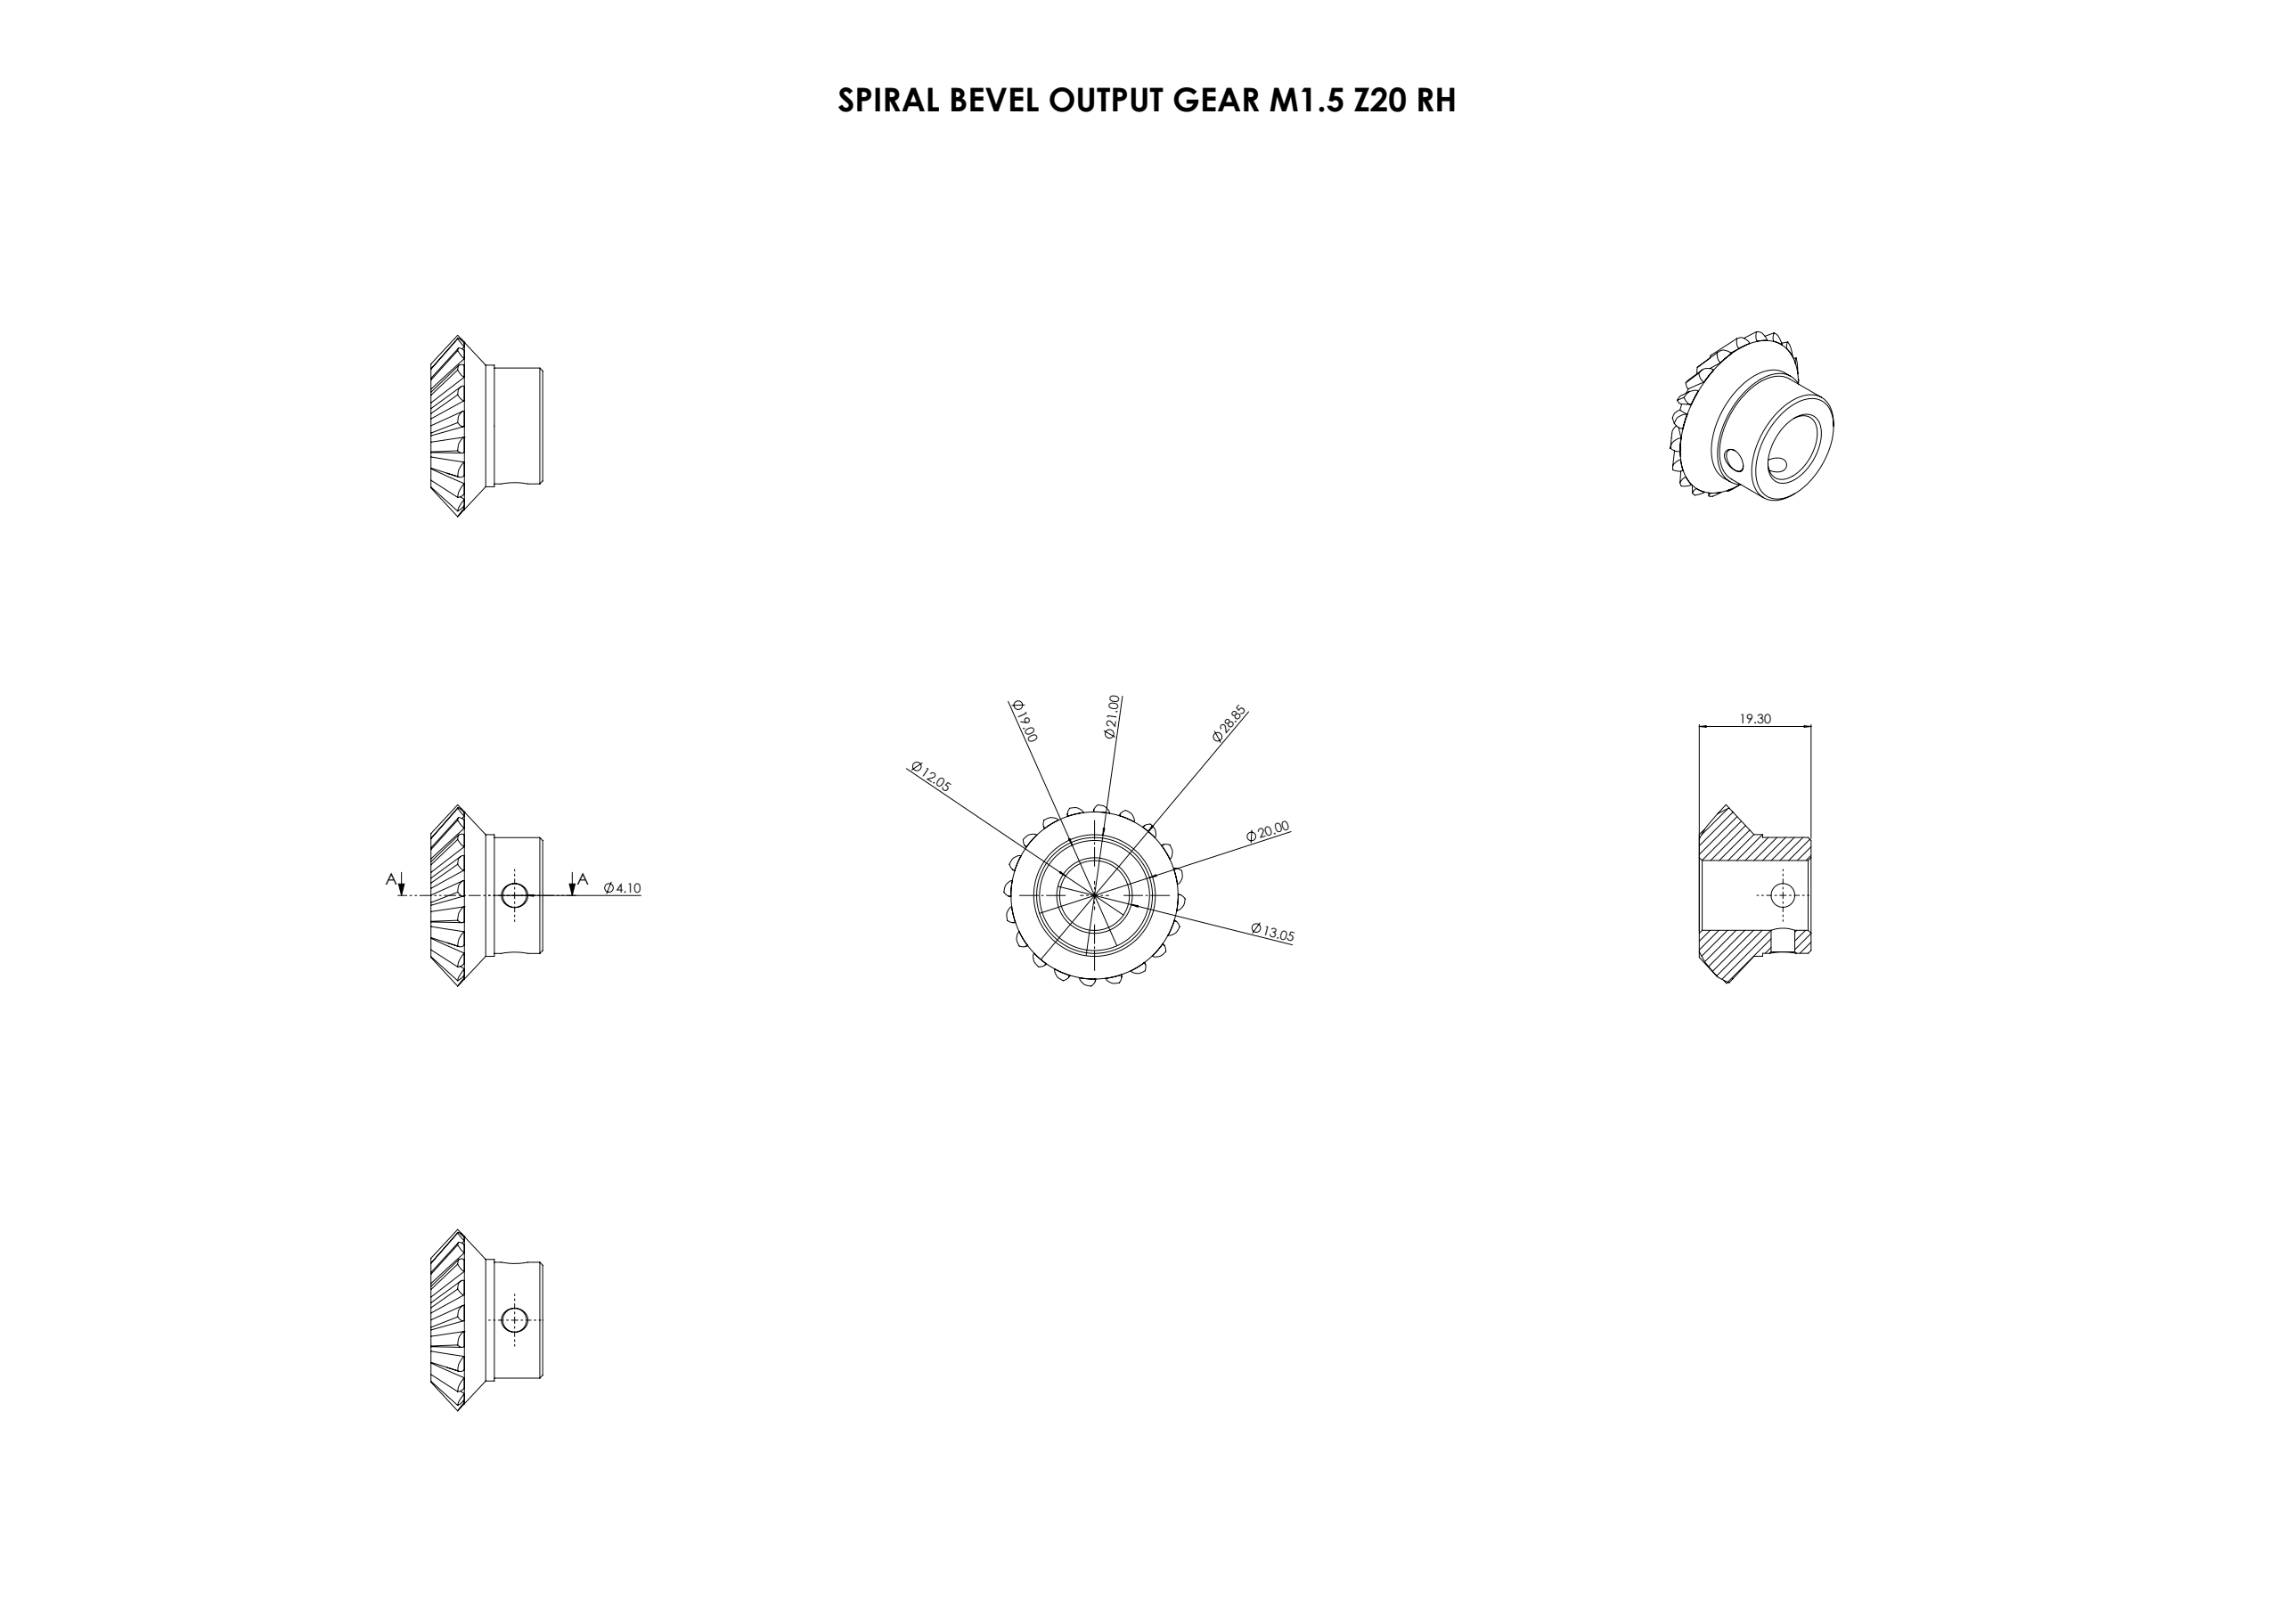
ISO-10303-21;
HEADER;
/* Generated by software containing ST-Developer
 * from STEP Tools, Inc. (www.steptools.com) 
 */

FILE_DESCRIPTION(
/* description */ (''),
/* implementation_level */ '2;1');

FILE_NAME(
/* name */ '03_Spiral_Bevel_Output_Gear_M1.5_Z20_RH.step',
/* time_stamp */ '2026-10-11T09:12:28-07:00',
/* author */ (''),
/* organization */ (''),
/* preprocessor_version */ 'ST-DEVELOPER v20.2',
/* originating_system */ 'Autodesk Translation Framework v15.15.0.0',
/* authorisation */ '');

FILE_SCHEMA (('AUTOMOTIVE_DESIGN { 1 0 10303 214 3 1 1 }'));
ENDSEC;

DATA;
#10=MECHANICAL_DESIGN_GEOMETRIC_PRESENTATION_REPRESENTATION('',(#649),#23254);
#133=B_SPLINE_SURFACE_WITH_KNOTS('',3,3,((#18119,#18120,#18121,#18122),
(#18123,#18124,#18125,#18126),(#18127,#18128,#18129,#18130),(#18131,#18132,
#18133,#18134),(#18135,#18136,#18137,#18138),(#18139,#18140,#18141,#18142)),
 .UNSPECIFIED.,.F.,.F.,.F.,(4,1,1,4),(4,4),(0.,0.285714285714286,0.571428571428571,
1.),(0.,1.),.UNSPECIFIED.);
#134=B_SPLINE_SURFACE_WITH_KNOTS('',3,3,((#18179,#18180,#18181,#18182),
(#18183,#18184,#18185,#18186),(#18187,#18188,#18189,#18190),(#18191,#18192,
#18193,#18194),(#18195,#18196,#18197,#18198),(#18199,#18200,#18201,#18202)),
 .UNSPECIFIED.,.F.,.F.,.F.,(4,1,1,4),(4,4),(0.,0.285714285714286,0.571428571428571,
1.),(0.,1.),.UNSPECIFIED.);
#135=B_SPLINE_SURFACE_WITH_KNOTS('',3,3,((#18239,#18240,#18241,#18242),
(#18243,#18244,#18245,#18246),(#18247,#18248,#18249,#18250),(#18251,#18252,
#18253,#18254),(#18255,#18256,#18257,#18258),(#18259,#18260,#18261,#18262)),
 .UNSPECIFIED.,.F.,.F.,.F.,(4,1,1,4),(4,4),(0.,0.285714285714286,0.571428571428571,
1.),(0.,1.),.UNSPECIFIED.);
#136=B_SPLINE_SURFACE_WITH_KNOTS('',3,3,((#18299,#18300,#18301,#18302),
(#18303,#18304,#18305,#18306),(#18307,#18308,#18309,#18310),(#18311,#18312,
#18313,#18314),(#18315,#18316,#18317,#18318),(#18319,#18320,#18321,#18322)),
 .UNSPECIFIED.,.F.,.F.,.F.,(4,1,1,4),(4,4),(0.,0.285714285714286,0.571428571428571,
1.),(0.,1.),.UNSPECIFIED.);
#137=B_SPLINE_SURFACE_WITH_KNOTS('',3,3,((#18359,#18360,#18361,#18362),
(#18363,#18364,#18365,#18366),(#18367,#18368,#18369,#18370),(#18371,#18372,
#18373,#18374),(#18375,#18376,#18377,#18378),(#18379,#18380,#18381,#18382)),
 .UNSPECIFIED.,.F.,.F.,.F.,(4,1,1,4),(4,4),(0.,0.285714285714286,0.571428571428571,
1.),(0.,1.),.UNSPECIFIED.);
#138=B_SPLINE_SURFACE_WITH_KNOTS('',3,3,((#18419,#18420,#18421,#18422),
(#18423,#18424,#18425,#18426),(#18427,#18428,#18429,#18430),(#18431,#18432,
#18433,#18434),(#18435,#18436,#18437,#18438),(#18439,#18440,#18441,#18442)),
 .UNSPECIFIED.,.F.,.F.,.F.,(4,1,1,4),(4,4),(0.,0.285714285714286,0.571428571428571,
1.),(0.,1.),.UNSPECIFIED.);
#139=B_SPLINE_SURFACE_WITH_KNOTS('',3,3,((#18479,#18480,#18481,#18482),
(#18483,#18484,#18485,#18486),(#18487,#18488,#18489,#18490),(#18491,#18492,
#18493,#18494),(#18495,#18496,#18497,#18498),(#18499,#18500,#18501,#18502)),
 .UNSPECIFIED.,.F.,.F.,.F.,(4,1,1,4),(4,4),(0.,0.285714285714286,0.571428571428571,
1.),(0.,1.),.UNSPECIFIED.);
#140=B_SPLINE_SURFACE_WITH_KNOTS('',3,3,((#18539,#18540,#18541,#18542),
(#18543,#18544,#18545,#18546),(#18547,#18548,#18549,#18550),(#18551,#18552,
#18553,#18554),(#18555,#18556,#18557,#18558),(#18559,#18560,#18561,#18562)),
 .UNSPECIFIED.,.F.,.F.,.F.,(4,1,1,4),(4,4),(0.,0.285714285714286,0.571428571428571,
1.),(0.,1.),.UNSPECIFIED.);
#141=B_SPLINE_SURFACE_WITH_KNOTS('',3,3,((#18599,#18600,#18601,#18602),
(#18603,#18604,#18605,#18606),(#18607,#18608,#18609,#18610),(#18611,#18612,
#18613,#18614),(#18615,#18616,#18617,#18618),(#18619,#18620,#18621,#18622)),
 .UNSPECIFIED.,.F.,.F.,.F.,(4,1,1,4),(4,4),(0.,0.285714285714286,0.571428571428571,
1.),(0.,1.),.UNSPECIFIED.);
#142=B_SPLINE_SURFACE_WITH_KNOTS('',3,3,((#18659,#18660,#18661,#18662),
(#18663,#18664,#18665,#18666),(#18667,#18668,#18669,#18670),(#18671,#18672,
#18673,#18674),(#18675,#18676,#18677,#18678),(#18679,#18680,#18681,#18682)),
 .UNSPECIFIED.,.F.,.F.,.F.,(4,1,1,4),(4,4),(0.,0.285714285714286,0.571428571428571,
1.),(0.,1.),.UNSPECIFIED.);
#143=B_SPLINE_SURFACE_WITH_KNOTS('',3,3,((#18719,#18720,#18721,#18722),
(#18723,#18724,#18725,#18726),(#18727,#18728,#18729,#18730),(#18731,#18732,
#18733,#18734),(#18735,#18736,#18737,#18738),(#18739,#18740,#18741,#18742)),
 .UNSPECIFIED.,.F.,.F.,.F.,(4,1,1,4),(4,4),(0.,0.285714285714286,0.571428571428571,
1.),(0.,1.),.UNSPECIFIED.);
#144=B_SPLINE_SURFACE_WITH_KNOTS('',3,3,((#18779,#18780,#18781,#18782),
(#18783,#18784,#18785,#18786),(#18787,#18788,#18789,#18790),(#18791,#18792,
#18793,#18794),(#18795,#18796,#18797,#18798),(#18799,#18800,#18801,#18802)),
 .UNSPECIFIED.,.F.,.F.,.F.,(4,1,1,4),(4,4),(0.,0.285714285714286,0.571428571428571,
1.),(0.,1.),.UNSPECIFIED.);
#145=B_SPLINE_SURFACE_WITH_KNOTS('',3,3,((#18839,#18840,#18841,#18842),
(#18843,#18844,#18845,#18846),(#18847,#18848,#18849,#18850),(#18851,#18852,
#18853,#18854),(#18855,#18856,#18857,#18858),(#18859,#18860,#18861,#18862)),
 .UNSPECIFIED.,.F.,.F.,.F.,(4,1,1,4),(4,4),(0.,0.285714285714286,0.571428571428571,
1.),(0.,1.),.UNSPECIFIED.);
#146=B_SPLINE_SURFACE_WITH_KNOTS('',3,3,((#18899,#18900,#18901,#18902),
(#18903,#18904,#18905,#18906),(#18907,#18908,#18909,#18910),(#18911,#18912,
#18913,#18914),(#18915,#18916,#18917,#18918),(#18919,#18920,#18921,#18922)),
 .UNSPECIFIED.,.F.,.F.,.F.,(4,1,1,4),(4,4),(0.,0.285714285714286,0.571428571428571,
1.),(0.,1.),.UNSPECIFIED.);
#147=B_SPLINE_SURFACE_WITH_KNOTS('',3,3,((#18959,#18960,#18961,#18962),
(#18963,#18964,#18965,#18966),(#18967,#18968,#18969,#18970),(#18971,#18972,
#18973,#18974),(#18975,#18976,#18977,#18978),(#18979,#18980,#18981,#18982)),
 .UNSPECIFIED.,.F.,.F.,.F.,(4,1,1,4),(4,4),(0.,0.285714285714286,0.571428571428571,
1.),(0.,1.),.UNSPECIFIED.);
#148=B_SPLINE_SURFACE_WITH_KNOTS('',3,3,((#19019,#19020,#19021,#19022),
(#19023,#19024,#19025,#19026),(#19027,#19028,#19029,#19030),(#19031,#19032,
#19033,#19034),(#19035,#19036,#19037,#19038),(#19039,#19040,#19041,#19042)),
 .UNSPECIFIED.,.F.,.F.,.F.,(4,1,1,4),(4,4),(0.,0.285714285714286,0.571428571428571,
1.),(0.,1.),.UNSPECIFIED.);
#149=B_SPLINE_SURFACE_WITH_KNOTS('',3,3,((#19079,#19080,#19081,#19082),
(#19083,#19084,#19085,#19086),(#19087,#19088,#19089,#19090),(#19091,#19092,
#19093,#19094),(#19095,#19096,#19097,#19098),(#19099,#19100,#19101,#19102)),
 .UNSPECIFIED.,.F.,.F.,.F.,(4,1,1,4),(4,4),(0.,0.285714285714286,0.571428571428571,
1.),(0.,1.),.UNSPECIFIED.);
#150=B_SPLINE_SURFACE_WITH_KNOTS('',3,3,((#19139,#19140,#19141,#19142),
(#19143,#19144,#19145,#19146),(#19147,#19148,#19149,#19150),(#19151,#19152,
#19153,#19154),(#19155,#19156,#19157,#19158),(#19159,#19160,#19161,#19162)),
 .UNSPECIFIED.,.F.,.F.,.F.,(4,1,1,4),(4,4),(0.,0.285714285714286,0.571428571428571,
1.),(0.,1.),.UNSPECIFIED.);
#151=B_SPLINE_SURFACE_WITH_KNOTS('',3,3,((#19199,#19200,#19201,#19202),
(#19203,#19204,#19205,#19206),(#19207,#19208,#19209,#19210),(#19211,#19212,
#19213,#19214),(#19215,#19216,#19217,#19218),(#19219,#19220,#19221,#19222)),
 .UNSPECIFIED.,.F.,.F.,.F.,(4,1,1,4),(4,4),(0.,0.285714285714286,0.571428571428571,
1.),(0.,1.),.UNSPECIFIED.);
#152=B_SPLINE_SURFACE_WITH_KNOTS('',3,3,((#19259,#19260,#19261,#19262),
(#19263,#19264,#19265,#19266),(#19267,#19268,#19269,#19270),(#19271,#19272,
#19273,#19274),(#19275,#19276,#19277,#19278),(#19279,#19280,#19281,#19282)),
 .UNSPECIFIED.,.F.,.F.,.F.,(4,1,1,4),(4,4),(0.,0.285714285714286,0.571428571428571,
1.),(0.,1.),.UNSPECIFIED.);
#153=B_SPLINE_SURFACE_WITH_KNOTS('',3,3,((#19319,#19320,#19321,#19322),
(#19323,#19324,#19325,#19326),(#19327,#19328,#19329,#19330),(#19331,#19332,
#19333,#19334),(#19335,#19336,#19337,#19338),(#19339,#19340,#19341,#19342),
(#19343,#19344,#19345,#19346),(#19347,#19348,#19349,#19350),(#19351,#19352,
#19353,#19354),(#19355,#19356,#19357,#19358),(#19359,#19360,#19361,#19362)),
 .UNSPECIFIED.,.F.,.F.,.F.,(4,1,1,1,1,1,1,1,4),(4,4),(0.,0.142857142857143,
0.285714285714286,0.357142857142857,0.428571428571429,0.571428571428571,
0.785714285714286,0.857142857142857,1.),(0.,1.),.UNSPECIFIED.);
#154=B_SPLINE_SURFACE_WITH_KNOTS('',3,3,((#19974,#19975,#19976,#19977),
(#19978,#19979,#19980,#19981),(#19982,#19983,#19984,#19985),(#19986,#19987,
#19988,#19989),(#19990,#19991,#19992,#19993),(#19994,#19995,#19996,#19997),
(#19998,#19999,#20000,#20001),(#20002,#20003,#20004,#20005),(#20006,#20007,
#20008,#20009),(#20010,#20011,#20012,#20013),(#20014,#20015,#20016,#20017)),
 .UNSPECIFIED.,.F.,.F.,.F.,(4,1,1,1,1,1,1,1,4),(4,4),(0.,0.142857142857143,
0.285714285714286,0.357142857142857,0.428571428571429,0.571428571428571,
0.785714285714286,0.857142857142857,1.),(0.,1.),.UNSPECIFIED.);
#155=B_SPLINE_SURFACE_WITH_KNOTS('',3,3,((#20025,#20026,#20027,#20028),
(#20029,#20030,#20031,#20032),(#20033,#20034,#20035,#20036),(#20037,#20038,
#20039,#20040),(#20041,#20042,#20043,#20044),(#20045,#20046,#20047,#20048),
(#20049,#20050,#20051,#20052),(#20053,#20054,#20055,#20056),(#20057,#20058,
#20059,#20060),(#20061,#20062,#20063,#20064),(#20065,#20066,#20067,#20068),
(#20069,#20070,#20071,#20072)),.UNSPECIFIED.,.F.,.F.,.F.,(4,1,1,1,1,1,1,
1,1,4),(4,4),(0.,0.142857142857143,0.285714285714286,0.321428571428571,
0.357142857142857,0.428571428571429,0.571428571428571,0.785714285714286,
0.857142857142857,1.),(0.,1.),.UNSPECIFIED.);
#156=B_SPLINE_SURFACE_WITH_KNOTS('',3,3,((#20080,#20081,#20082,#20083),
(#20084,#20085,#20086,#20087),(#20088,#20089,#20090,#20091),(#20092,#20093,
#20094,#20095),(#20096,#20097,#20098,#20099),(#20100,#20101,#20102,#20103),
(#20104,#20105,#20106,#20107),(#20108,#20109,#20110,#20111),(#20112,#20113,
#20114,#20115),(#20116,#20117,#20118,#20119),(#20120,#20121,#20122,#20123),
(#20124,#20125,#20126,#20127)),.UNSPECIFIED.,.F.,.F.,.F.,(4,1,1,1,1,1,1,
1,1,4),(4,4),(0.,0.142857142857143,0.285714285714286,0.321428571428571,
0.357142857142857,0.428571428571429,0.571428571428571,0.785714285714286,
0.857142857142857,1.),(0.,1.),.UNSPECIFIED.);
#157=B_SPLINE_SURFACE_WITH_KNOTS('',3,3,((#20135,#20136,#20137,#20138),
(#20139,#20140,#20141,#20142),(#20143,#20144,#20145,#20146),(#20147,#20148,
#20149,#20150),(#20151,#20152,#20153,#20154),(#20155,#20156,#20157,#20158),
(#20159,#20160,#20161,#20162),(#20163,#20164,#20165,#20166),(#20167,#20168,
#20169,#20170),(#20171,#20172,#20173,#20174),(#20175,#20176,#20177,#20178)),
 .UNSPECIFIED.,.F.,.F.,.F.,(4,1,1,1,1,1,1,1,4),(4,4),(0.,0.142857142857143,
0.285714285714286,0.357142857142857,0.428571428571429,0.571428571428571,
0.785714285714286,0.857142857142857,1.),(0.,1.),.UNSPECIFIED.);
#158=B_SPLINE_SURFACE_WITH_KNOTS('',3,3,((#20186,#20187,#20188,#20189),
(#20190,#20191,#20192,#20193),(#20194,#20195,#20196,#20197),(#20198,#20199,
#20200,#20201),(#20202,#20203,#20204,#20205),(#20206,#20207,#20208,#20209),
(#20210,#20211,#20212,#20213),(#20214,#20215,#20216,#20217),(#20218,#20219,
#20220,#20221),(#20222,#20223,#20224,#20225),(#20226,#20227,#20228,#20229)),
 .UNSPECIFIED.,.F.,.F.,.F.,(4,1,1,1,1,1,1,1,4),(4,4),(0.,0.142857142857143,
0.285714285714286,0.357142857142857,0.428571428571429,0.571428571428571,
0.785714285714286,0.857142857142857,1.),(0.,1.),.UNSPECIFIED.);
#159=B_SPLINE_SURFACE_WITH_KNOTS('',3,3,((#20237,#20238,#20239,#20240),
(#20241,#20242,#20243,#20244),(#20245,#20246,#20247,#20248),(#20249,#20250,
#20251,#20252),(#20253,#20254,#20255,#20256),(#20257,#20258,#20259,#20260),
(#20261,#20262,#20263,#20264),(#20265,#20266,#20267,#20268),(#20269,#20270,
#20271,#20272),(#20273,#20274,#20275,#20276),(#20277,#20278,#20279,#20280)),
 .UNSPECIFIED.,.F.,.F.,.F.,(4,1,1,1,1,1,1,1,4),(4,4),(0.,0.142857142857143,
0.285714285714286,0.357142857142857,0.428571428571429,0.571428571428571,
0.785714285714286,0.857142857142857,1.),(0.,1.),.UNSPECIFIED.);
#160=B_SPLINE_SURFACE_WITH_KNOTS('',3,3,((#20288,#20289,#20290,#20291),
(#20292,#20293,#20294,#20295),(#20296,#20297,#20298,#20299),(#20300,#20301,
#20302,#20303),(#20304,#20305,#20306,#20307),(#20308,#20309,#20310,#20311),
(#20312,#20313,#20314,#20315),(#20316,#20317,#20318,#20319),(#20320,#20321,
#20322,#20323),(#20324,#20325,#20326,#20327),(#20328,#20329,#20330,#20331),
(#20332,#20333,#20334,#20335)),.UNSPECIFIED.,.F.,.F.,.F.,(4,1,1,1,1,1,1,
1,1,4),(4,4),(0.,0.142857142857143,0.285714285714286,0.321428571428571,
0.357142857142857,0.428571428571429,0.571428571428571,0.785714285714286,
0.857142857142857,1.),(0.,1.),.UNSPECIFIED.);
#161=B_SPLINE_SURFACE_WITH_KNOTS('',3,3,((#20343,#20344,#20345,#20346),
(#20347,#20348,#20349,#20350),(#20351,#20352,#20353,#20354),(#20355,#20356,
#20357,#20358),(#20359,#20360,#20361,#20362),(#20363,#20364,#20365,#20366),
(#20367,#20368,#20369,#20370),(#20371,#20372,#20373,#20374),(#20375,#20376,
#20377,#20378),(#20379,#20380,#20381,#20382),(#20383,#20384,#20385,#20386),
(#20387,#20388,#20389,#20390)),.UNSPECIFIED.,.F.,.F.,.F.,(4,1,1,1,1,1,1,
1,1,4),(4,4),(0.,0.142857142857143,0.285714285714286,0.321428571428571,
0.357142857142857,0.428571428571429,0.571428571428571,0.785714285714286,
0.857142857142857,1.),(0.,1.),.UNSPECIFIED.);
#162=B_SPLINE_SURFACE_WITH_KNOTS('',3,3,((#20398,#20399,#20400,#20401),
(#20402,#20403,#20404,#20405),(#20406,#20407,#20408,#20409),(#20410,#20411,
#20412,#20413),(#20414,#20415,#20416,#20417),(#20418,#20419,#20420,#20421),
(#20422,#20423,#20424,#20425),(#20426,#20427,#20428,#20429),(#20430,#20431,
#20432,#20433),(#20434,#20435,#20436,#20437),(#20438,#20439,#20440,#20441)),
 .UNSPECIFIED.,.F.,.F.,.F.,(4,1,1,1,1,1,1,1,4),(4,4),(0.,0.142857142857143,
0.285714285714286,0.357142857142857,0.428571428571429,0.571428571428571,
0.785714285714286,0.857142857142857,1.),(0.,1.),.UNSPECIFIED.);
#163=B_SPLINE_SURFACE_WITH_KNOTS('',3,3,((#20449,#20450,#20451,#20452),
(#20453,#20454,#20455,#20456),(#20457,#20458,#20459,#20460),(#20461,#20462,
#20463,#20464),(#20465,#20466,#20467,#20468),(#20469,#20470,#20471,#20472),
(#20473,#20474,#20475,#20476),(#20477,#20478,#20479,#20480),(#20481,#20482,
#20483,#20484),(#20485,#20486,#20487,#20488),(#20489,#20490,#20491,#20492)),
 .UNSPECIFIED.,.F.,.F.,.F.,(4,1,1,1,1,1,1,1,4),(4,4),(0.,0.142857142857143,
0.285714285714286,0.357142857142857,0.428571428571429,0.571428571428571,
0.785714285714286,0.857142857142857,1.),(0.,1.),.UNSPECIFIED.);
#164=B_SPLINE_SURFACE_WITH_KNOTS('',3,3,((#20500,#20501,#20502,#20503),
(#20504,#20505,#20506,#20507),(#20508,#20509,#20510,#20511),(#20512,#20513,
#20514,#20515),(#20516,#20517,#20518,#20519),(#20520,#20521,#20522,#20523),
(#20524,#20525,#20526,#20527),(#20528,#20529,#20530,#20531),(#20532,#20533,
#20534,#20535),(#20536,#20537,#20538,#20539),(#20540,#20541,#20542,#20543)),
 .UNSPECIFIED.,.F.,.F.,.F.,(4,1,1,1,1,1,1,1,4),(4,4),(0.,0.142857142857143,
0.285714285714286,0.357142857142857,0.428571428571429,0.571428571428571,
0.785714285714286,0.857142857142857,1.),(0.,1.),.UNSPECIFIED.);
#165=B_SPLINE_SURFACE_WITH_KNOTS('',3,3,((#20551,#20552,#20553,#20554),
(#20555,#20556,#20557,#20558),(#20559,#20560,#20561,#20562),(#20563,#20564,
#20565,#20566),(#20567,#20568,#20569,#20570),(#20571,#20572,#20573,#20574),
(#20575,#20576,#20577,#20578),(#20579,#20580,#20581,#20582),(#20583,#20584,
#20585,#20586),(#20587,#20588,#20589,#20590),(#20591,#20592,#20593,#20594),
(#20595,#20596,#20597,#20598)),.UNSPECIFIED.,.F.,.F.,.F.,(4,1,1,1,1,1,1,
1,1,4),(4,4),(0.,0.142857142857143,0.285714285714286,0.321428571428571,
0.357142857142857,0.428571428571429,0.571428571428571,0.785714285714286,
0.857142857142857,1.),(0.,1.),.UNSPECIFIED.);
#166=B_SPLINE_SURFACE_WITH_KNOTS('',3,3,((#20606,#20607,#20608,#20609),
(#20610,#20611,#20612,#20613),(#20614,#20615,#20616,#20617),(#20618,#20619,
#20620,#20621),(#20622,#20623,#20624,#20625),(#20626,#20627,#20628,#20629),
(#20630,#20631,#20632,#20633),(#20634,#20635,#20636,#20637),(#20638,#20639,
#20640,#20641),(#20642,#20643,#20644,#20645),(#20646,#20647,#20648,#20649),
(#20650,#20651,#20652,#20653)),.UNSPECIFIED.,.F.,.F.,.F.,(4,1,1,1,1,1,1,
1,1,4),(4,4),(0.,0.142857142857143,0.285714285714286,0.321428571428571,
0.357142857142857,0.428571428571429,0.571428571428571,0.785714285714286,
0.857142857142857,1.),(0.,1.),.UNSPECIFIED.);
#167=B_SPLINE_SURFACE_WITH_KNOTS('',3,3,((#20661,#20662,#20663,#20664),
(#20665,#20666,#20667,#20668),(#20669,#20670,#20671,#20672),(#20673,#20674,
#20675,#20676),(#20677,#20678,#20679,#20680),(#20681,#20682,#20683,#20684),
(#20685,#20686,#20687,#20688),(#20689,#20690,#20691,#20692),(#20693,#20694,
#20695,#20696),(#20697,#20698,#20699,#20700),(#20701,#20702,#20703,#20704)),
 .UNSPECIFIED.,.F.,.F.,.F.,(4,1,1,1,1,1,1,1,4),(4,4),(0.,0.142857142857143,
0.285714285714286,0.357142857142857,0.428571428571429,0.571428571428571,
0.785714285714286,0.857142857142857,1.),(0.,1.),.UNSPECIFIED.);
#168=B_SPLINE_SURFACE_WITH_KNOTS('',3,3,((#20712,#20713,#20714,#20715),
(#20716,#20717,#20718,#20719),(#20720,#20721,#20722,#20723),(#20724,#20725,
#20726,#20727),(#20728,#20729,#20730,#20731),(#20732,#20733,#20734,#20735),
(#20736,#20737,#20738,#20739),(#20740,#20741,#20742,#20743),(#20744,#20745,
#20746,#20747),(#20748,#20749,#20750,#20751),(#20752,#20753,#20754,#20755)),
 .UNSPECIFIED.,.F.,.F.,.F.,(4,1,1,1,1,1,1,1,4),(4,4),(0.,0.142857142857143,
0.285714285714286,0.357142857142857,0.428571428571429,0.571428571428571,
0.785714285714286,0.857142857142857,1.),(0.,1.),.UNSPECIFIED.);
#169=B_SPLINE_SURFACE_WITH_KNOTS('',3,3,((#20763,#20764,#20765,#20766),
(#20767,#20768,#20769,#20770),(#20771,#20772,#20773,#20774),(#20775,#20776,
#20777,#20778),(#20779,#20780,#20781,#20782),(#20783,#20784,#20785,#20786),
(#20787,#20788,#20789,#20790),(#20791,#20792,#20793,#20794),(#20795,#20796,
#20797,#20798),(#20799,#20800,#20801,#20802),(#20803,#20804,#20805,#20806)),
 .UNSPECIFIED.,.F.,.F.,.F.,(4,1,1,1,1,1,1,1,4),(4,4),(0.,0.142857142857143,
0.285714285714286,0.357142857142857,0.428571428571429,0.571428571428571,
0.785714285714286,0.857142857142857,1.),(0.,1.),.UNSPECIFIED.);
#170=B_SPLINE_SURFACE_WITH_KNOTS('',3,3,((#20814,#20815,#20816,#20817),
(#20818,#20819,#20820,#20821),(#20822,#20823,#20824,#20825),(#20826,#20827,
#20828,#20829),(#20830,#20831,#20832,#20833),(#20834,#20835,#20836,#20837),
(#20838,#20839,#20840,#20841),(#20842,#20843,#20844,#20845),(#20846,#20847,
#20848,#20849),(#20850,#20851,#20852,#20853),(#20854,#20855,#20856,#20857),
(#20858,#20859,#20860,#20861)),.UNSPECIFIED.,.F.,.F.,.F.,(4,1,1,1,1,1,1,
1,1,4),(4,4),(0.,0.142857142857143,0.285714285714286,0.321428571428571,
0.357142857142857,0.428571428571429,0.571428571428571,0.785714285714286,
0.857142857142857,1.),(0.,1.),.UNSPECIFIED.);
#171=B_SPLINE_SURFACE_WITH_KNOTS('',3,3,((#20869,#20870,#20871,#20872),
(#20873,#20874,#20875,#20876),(#20877,#20878,#20879,#20880),(#20881,#20882,
#20883,#20884),(#20885,#20886,#20887,#20888),(#20889,#20890,#20891,#20892),
(#20893,#20894,#20895,#20896),(#20897,#20898,#20899,#20900),(#20901,#20902,
#20903,#20904),(#20905,#20906,#20907,#20908),(#20909,#20910,#20911,#20912),
(#20913,#20914,#20915,#20916)),.UNSPECIFIED.,.F.,.F.,.F.,(4,1,1,1,1,1,1,
1,1,4),(4,4),(0.,0.142857142857143,0.285714285714286,0.321428571428571,
0.357142857142857,0.428571428571429,0.571428571428571,0.785714285714286,
0.857142857142857,1.),(0.,1.),.UNSPECIFIED.);
#172=B_SPLINE_SURFACE_WITH_KNOTS('',3,3,((#20924,#20925,#20926,#20927),
(#20928,#20929,#20930,#20931),(#20932,#20933,#20934,#20935),(#20936,#20937,
#20938,#20939),(#20940,#20941,#20942,#20943),(#20944,#20945,#20946,#20947),
(#20948,#20949,#20950,#20951),(#20952,#20953,#20954,#20955),(#20956,#20957,
#20958,#20959),(#20960,#20961,#20962,#20963),(#20964,#20965,#20966,#20967)),
 .UNSPECIFIED.,.F.,.F.,.F.,(4,1,1,1,1,1,1,1,4),(4,4),(0.,0.142857142857143,
0.285714285714286,0.357142857142857,0.428571428571429,0.571428571428571,
0.785714285714286,0.857142857142857,1.),(0.,1.),.UNSPECIFIED.);
#255=(
BOUNDED_CURVE()
B_SPLINE_CURVE(5,(#16035,#16036,#16037,#16038,#16039,#16040,#16041,#16042,
#16043,#16044,#16045,#16046,#16047,#16048,#16049,#16050,#16051,#16052,#16053,
#16054,#16055,#16056,#16057,#16058,#16059,#16060,#16061,#16062,#16063,#16064,
#16065,#16066,#16067,#16068,#16069),.UNSPECIFIED.,.F.,.F.)
B_SPLINE_CURVE_WITH_KNOTS((6,1,1,1,1,1,1,1,1,1,1,1,1,1,1,1,1,1,1,1,1,1,
1,1,1,1,1,1,1,1,6),(0.,0.0333333333333333,0.0666666666666667,0.1,0.133333333333333,
0.166666666666667,0.2,0.233333333333333,0.266666666666667,0.3,0.333333333333333,
0.366666666666667,0.4,0.433333333333333,0.466666666666667,0.5,0.533333333333333,
0.566666666666667,0.6,0.633333333333333,0.666666666666667,0.7,0.733333333333333,
0.766666666666667,0.8,0.833333333333333,0.866666666666667,0.9,0.933333333333333,
0.966666666666667,1.),.UNSPECIFIED.)
CURVE()
GEOMETRIC_REPRESENTATION_ITEM()
RATIONAL_B_SPLINE_CURVE((1.,1.,1.,1.,1.,1.,1.,1.,1.,1.,1.,1.,1.,1.,1.,1.,
1.,1.,1.,1.,1.,1.,1.,1.,1.,1.,1.,1.,1.,1.,1.,1.,1.,1.,1.))
REPRESENTATION_ITEM('')
);
#256=(
BOUNDED_CURVE()
B_SPLINE_CURVE(5,(#16071,#16072,#16073,#16074,#16075,#16076,#16077,#16078,
#16079,#16080,#16081,#16082,#16083,#16084,#16085,#16086,#16087,#16088,#16089,
#16090,#16091,#16092,#16093,#16094,#16095,#16096,#16097,#16098,#16099,#16100,
#16101,#16102,#16103,#16104,#16105),.UNSPECIFIED.,.F.,.F.)
B_SPLINE_CURVE_WITH_KNOTS((6,1,1,1,1,1,1,1,1,1,1,1,1,1,1,1,1,1,1,1,1,1,
1,1,1,1,1,1,1,1,6),(0.,0.0333333333333333,0.0666666666666667,0.1,0.133333333333333,
0.166666666666667,0.2,0.233333333333333,0.266666666666667,0.3,0.333333333333333,
0.366666666666667,0.4,0.433333333333333,0.466666666666667,0.5,0.533333333333333,
0.566666666666667,0.6,0.633333333333333,0.666666666666667,0.7,0.733333333333333,
0.766666666666667,0.8,0.833333333333333,0.866666666666667,0.9,0.933333333333333,
0.966666666666667,1.),.UNSPECIFIED.)
CURVE()
GEOMETRIC_REPRESENTATION_ITEM()
RATIONAL_B_SPLINE_CURVE((1.,1.,1.,1.,1.,1.,1.,1.,1.,1.,1.,1.,1.,1.,1.,1.,
1.,1.,1.,1.,1.,1.,1.,1.,1.,1.,1.,1.,1.,1.,1.,1.,1.,1.,1.))
REPRESENTATION_ITEM('')
);
#257=(
BOUNDED_CURVE()
B_SPLINE_CURVE(5,(#16109,#16110,#16111,#16112,#16113,#16114,#16115,#16116,
#16117,#16118,#16119,#16120,#16121,#16122,#16123,#16124,#16125,#16126,#16127,
#16128,#16129,#16130,#16131,#16132,#16133,#16134,#16135,#16136,#16137,#16138,
#16139,#16140,#16141,#16142,#16143),.UNSPECIFIED.,.F.,.F.)
B_SPLINE_CURVE_WITH_KNOTS((6,1,1,1,1,1,1,1,1,1,1,1,1,1,1,1,1,1,1,1,1,1,
1,1,1,1,1,1,1,1,6),(0.,0.0333333333333333,0.0666666666666667,0.1,0.133333333333333,
0.166666666666667,0.2,0.233333333333333,0.266666666666667,0.3,0.333333333333333,
0.366666666666667,0.4,0.433333333333333,0.466666666666667,0.5,0.533333333333333,
0.566666666666667,0.6,0.633333333333333,0.666666666666667,0.7,0.733333333333333,
0.766666666666667,0.8,0.833333333333333,0.866666666666667,0.9,0.933333333333333,
0.966666666666667,1.),.UNSPECIFIED.)
CURVE()
GEOMETRIC_REPRESENTATION_ITEM()
RATIONAL_B_SPLINE_CURVE((1.,1.,1.,1.,1.,1.,1.,1.,1.,1.,1.,1.,1.,1.,1.,1.,
1.,1.,1.,1.,1.,1.,1.,1.,1.,1.,1.,1.,1.,1.,1.,1.,1.,1.,1.))
REPRESENTATION_ITEM('')
);
#258=(
BOUNDED_CURVE()
B_SPLINE_CURVE(5,(#16145,#16146,#16147,#16148,#16149,#16150,#16151,#16152,
#16153,#16154,#16155,#16156,#16157,#16158,#16159,#16160,#16161,#16162,#16163,
#16164,#16165,#16166,#16167,#16168,#16169,#16170,#16171,#16172,#16173,#16174,
#16175,#16176,#16177,#16178,#16179),.UNSPECIFIED.,.F.,.F.)
B_SPLINE_CURVE_WITH_KNOTS((6,1,1,1,1,1,1,1,1,1,1,1,1,1,1,1,1,1,1,1,1,1,
1,1,1,1,1,1,1,1,6),(0.,0.0333333333333333,0.0666666666666667,0.1,0.133333333333333,
0.166666666666667,0.2,0.233333333333333,0.266666666666667,0.3,0.333333333333333,
0.366666666666667,0.4,0.433333333333333,0.466666666666667,0.5,0.533333333333333,
0.566666666666667,0.6,0.633333333333333,0.666666666666667,0.7,0.733333333333333,
0.766666666666667,0.8,0.833333333333333,0.866666666666667,0.9,0.933333333333333,
0.966666666666667,1.),.UNSPECIFIED.)
CURVE()
GEOMETRIC_REPRESENTATION_ITEM()
RATIONAL_B_SPLINE_CURVE((1.,1.,1.,1.,1.,1.,1.,1.,1.,1.,1.,1.,1.,1.,1.,1.,
1.,1.,1.,1.,1.,1.,1.,1.,1.,1.,1.,1.,1.,1.,1.,1.,1.,1.,1.))
REPRESENTATION_ITEM('')
);
#259=(
BOUNDED_CURVE()
B_SPLINE_CURVE(5,(#16183,#16184,#16185,#16186,#16187,#16188,#16189,#16190,
#16191,#16192,#16193,#16194,#16195,#16196,#16197,#16198,#16199,#16200,#16201,
#16202,#16203,#16204,#16205,#16206,#16207,#16208,#16209,#16210,#16211,#16212,
#16213,#16214,#16215,#16216,#16217),.UNSPECIFIED.,.F.,.F.)
B_SPLINE_CURVE_WITH_KNOTS((6,1,1,1,1,1,1,1,1,1,1,1,1,1,1,1,1,1,1,1,1,1,
1,1,1,1,1,1,1,1,6),(0.,0.0333333333333333,0.0666666666666667,0.1,0.133333333333333,
0.166666666666667,0.2,0.233333333333333,0.266666666666667,0.3,0.333333333333333,
0.366666666666667,0.4,0.433333333333333,0.466666666666667,0.5,0.533333333333333,
0.566666666666667,0.6,0.633333333333333,0.666666666666667,0.7,0.733333333333333,
0.766666666666667,0.8,0.833333333333333,0.866666666666667,0.9,0.933333333333333,
0.966666666666667,1.),.UNSPECIFIED.)
CURVE()
GEOMETRIC_REPRESENTATION_ITEM()
RATIONAL_B_SPLINE_CURVE((1.,1.,1.,1.,1.,1.,1.,1.,1.,1.,1.,1.,1.,1.,1.,1.,
1.,1.,1.,1.,1.,1.,1.,1.,1.,1.,1.,1.,1.,1.,1.,1.,1.,1.,1.))
REPRESENTATION_ITEM('')
);
#260=(
BOUNDED_CURVE()
B_SPLINE_CURVE(5,(#16219,#16220,#16221,#16222,#16223,#16224,#16225,#16226,
#16227,#16228,#16229,#16230,#16231,#16232,#16233,#16234,#16235,#16236,#16237,
#16238,#16239,#16240,#16241,#16242,#16243,#16244,#16245,#16246,#16247,#16248,
#16249,#16250,#16251,#16252,#16253),.UNSPECIFIED.,.F.,.F.)
B_SPLINE_CURVE_WITH_KNOTS((6,1,1,1,1,1,1,1,1,1,1,1,1,1,1,1,1,1,1,1,1,1,
1,1,1,1,1,1,1,1,6),(0.,0.0333333333333333,0.0666666666666667,0.1,0.133333333333333,
0.166666666666667,0.2,0.233333333333333,0.266666666666667,0.3,0.333333333333333,
0.366666666666667,0.4,0.433333333333333,0.466666666666667,0.5,0.533333333333333,
0.566666666666667,0.6,0.633333333333333,0.666666666666667,0.7,0.733333333333333,
0.766666666666667,0.8,0.833333333333333,0.866666666666667,0.9,0.933333333333333,
0.966666666666667,1.),.UNSPECIFIED.)
CURVE()
GEOMETRIC_REPRESENTATION_ITEM()
RATIONAL_B_SPLINE_CURVE((1.,1.,1.,1.,1.,1.,1.,1.,1.,1.,1.,1.,1.,1.,1.,1.,
1.,1.,1.,1.,1.,1.,1.,1.,1.,1.,1.,1.,1.,1.,1.,1.,1.,1.,1.))
REPRESENTATION_ITEM('')
);
#261=(
BOUNDED_CURVE()
B_SPLINE_CURVE(5,(#16257,#16258,#16259,#16260,#16261,#16262,#16263,#16264,
#16265,#16266,#16267,#16268,#16269,#16270,#16271,#16272,#16273,#16274,#16275,
#16276,#16277,#16278,#16279,#16280,#16281,#16282,#16283,#16284,#16285,#16286,
#16287,#16288,#16289,#16290,#16291),.UNSPECIFIED.,.F.,.F.)
B_SPLINE_CURVE_WITH_KNOTS((6,1,1,1,1,1,1,1,1,1,1,1,1,1,1,1,1,1,1,1,1,1,
1,1,1,1,1,1,1,1,6),(0.,0.0333333333333333,0.0666666666666667,0.1,0.133333333333333,
0.166666666666667,0.2,0.233333333333333,0.266666666666667,0.3,0.333333333333333,
0.366666666666667,0.4,0.433333333333333,0.466666666666667,0.5,0.533333333333333,
0.566666666666667,0.6,0.633333333333333,0.666666666666667,0.7,0.733333333333333,
0.766666666666667,0.8,0.833333333333333,0.866666666666667,0.9,0.933333333333333,
0.966666666666667,1.),.UNSPECIFIED.)
CURVE()
GEOMETRIC_REPRESENTATION_ITEM()
RATIONAL_B_SPLINE_CURVE((1.,1.,1.,1.,1.,1.,1.,1.,1.,1.,1.,1.,1.,1.,1.,1.,
1.,1.,1.,1.,1.,1.,1.,1.,1.,1.,1.,1.,1.,1.,1.,1.,1.,1.,1.))
REPRESENTATION_ITEM('')
);
#262=(
BOUNDED_CURVE()
B_SPLINE_CURVE(5,(#16293,#16294,#16295,#16296,#16297,#16298,#16299,#16300,
#16301,#16302,#16303,#16304,#16305,#16306,#16307,#16308,#16309,#16310,#16311,
#16312,#16313,#16314,#16315,#16316,#16317,#16318,#16319,#16320,#16321,#16322,
#16323,#16324,#16325,#16326,#16327),.UNSPECIFIED.,.F.,.F.)
B_SPLINE_CURVE_WITH_KNOTS((6,1,1,1,1,1,1,1,1,1,1,1,1,1,1,1,1,1,1,1,1,1,
1,1,1,1,1,1,1,1,6),(0.,0.0333333333333333,0.0666666666666667,0.1,0.133333333333333,
0.166666666666667,0.2,0.233333333333333,0.266666666666667,0.3,0.333333333333333,
0.366666666666667,0.4,0.433333333333333,0.466666666666667,0.5,0.533333333333333,
0.566666666666667,0.6,0.633333333333333,0.666666666666667,0.7,0.733333333333333,
0.766666666666667,0.8,0.833333333333333,0.866666666666667,0.9,0.933333333333333,
0.966666666666667,1.),.UNSPECIFIED.)
CURVE()
GEOMETRIC_REPRESENTATION_ITEM()
RATIONAL_B_SPLINE_CURVE((1.,1.,1.,1.,1.,1.,1.,1.,1.,1.,1.,1.,1.,1.,1.,1.,
1.,1.,1.,1.,1.,1.,1.,1.,1.,1.,1.,1.,1.,1.,1.,1.,1.,1.,1.))
REPRESENTATION_ITEM('')
);
#263=(
BOUNDED_CURVE()
B_SPLINE_CURVE(5,(#16331,#16332,#16333,#16334,#16335,#16336,#16337,#16338,
#16339,#16340,#16341,#16342,#16343,#16344,#16345,#16346,#16347,#16348,#16349,
#16350,#16351,#16352,#16353,#16354,#16355,#16356,#16357,#16358,#16359,#16360,
#16361,#16362,#16363,#16364,#16365),.UNSPECIFIED.,.F.,.F.)
B_SPLINE_CURVE_WITH_KNOTS((6,1,1,1,1,1,1,1,1,1,1,1,1,1,1,1,1,1,1,1,1,1,
1,1,1,1,1,1,1,1,6),(0.,0.0333333333333333,0.0666666666666667,0.1,0.133333333333333,
0.166666666666667,0.2,0.233333333333333,0.266666666666667,0.3,0.333333333333333,
0.366666666666667,0.4,0.433333333333333,0.466666666666667,0.5,0.533333333333333,
0.566666666666667,0.6,0.633333333333333,0.666666666666667,0.7,0.733333333333333,
0.766666666666667,0.8,0.833333333333333,0.866666666666667,0.9,0.933333333333333,
0.966666666666667,1.),.UNSPECIFIED.)
CURVE()
GEOMETRIC_REPRESENTATION_ITEM()
RATIONAL_B_SPLINE_CURVE((1.,1.,1.,1.,1.,1.,1.,1.,1.,1.,1.,1.,1.,1.,1.,1.,
1.,1.,1.,1.,1.,1.,1.,1.,1.,1.,1.,1.,1.,1.,1.,1.,1.,1.,1.))
REPRESENTATION_ITEM('')
);
#264=(
BOUNDED_CURVE()
B_SPLINE_CURVE(5,(#16367,#16368,#16369,#16370,#16371,#16372,#16373,#16374,
#16375,#16376,#16377,#16378,#16379,#16380,#16381,#16382,#16383,#16384,#16385,
#16386,#16387,#16388,#16389,#16390,#16391,#16392,#16393,#16394,#16395,#16396,
#16397,#16398,#16399,#16400,#16401),.UNSPECIFIED.,.F.,.F.)
B_SPLINE_CURVE_WITH_KNOTS((6,1,1,1,1,1,1,1,1,1,1,1,1,1,1,1,1,1,1,1,1,1,
1,1,1,1,1,1,1,1,6),(0.,0.0333333333333333,0.0666666666666667,0.1,0.133333333333333,
0.166666666666667,0.2,0.233333333333333,0.266666666666667,0.3,0.333333333333333,
0.366666666666667,0.4,0.433333333333333,0.466666666666667,0.5,0.533333333333333,
0.566666666666667,0.6,0.633333333333333,0.666666666666667,0.7,0.733333333333333,
0.766666666666667,0.8,0.833333333333333,0.866666666666667,0.9,0.933333333333333,
0.966666666666667,1.),.UNSPECIFIED.)
CURVE()
GEOMETRIC_REPRESENTATION_ITEM()
RATIONAL_B_SPLINE_CURVE((1.,1.,1.,1.,1.,1.,1.,1.,1.,1.,1.,1.,1.,1.,1.,1.,
1.,1.,1.,1.,1.,1.,1.,1.,1.,1.,1.,1.,1.,1.,1.,1.,1.,1.,1.))
REPRESENTATION_ITEM('')
);
#265=(
BOUNDED_CURVE()
B_SPLINE_CURVE(5,(#16405,#16406,#16407,#16408,#16409,#16410,#16411,#16412,
#16413,#16414,#16415,#16416,#16417,#16418,#16419,#16420,#16421,#16422,#16423,
#16424,#16425,#16426,#16427,#16428,#16429,#16430,#16431,#16432,#16433,#16434,
#16435,#16436,#16437,#16438,#16439),.UNSPECIFIED.,.F.,.F.)
B_SPLINE_CURVE_WITH_KNOTS((6,1,1,1,1,1,1,1,1,1,1,1,1,1,1,1,1,1,1,1,1,1,
1,1,1,1,1,1,1,1,6),(0.,0.0333333333333333,0.0666666666666667,0.1,0.133333333333333,
0.166666666666667,0.2,0.233333333333333,0.266666666666667,0.3,0.333333333333333,
0.366666666666667,0.4,0.433333333333333,0.466666666666667,0.5,0.533333333333333,
0.566666666666667,0.6,0.633333333333333,0.666666666666667,0.7,0.733333333333333,
0.766666666666667,0.8,0.833333333333333,0.866666666666667,0.9,0.933333333333333,
0.966666666666667,1.),.UNSPECIFIED.)
CURVE()
GEOMETRIC_REPRESENTATION_ITEM()
RATIONAL_B_SPLINE_CURVE((1.,1.,1.,1.,1.,1.,1.,1.,1.,1.,1.,1.,1.,1.,1.,1.,
1.,1.,1.,1.,1.,1.,1.,1.,1.,1.,1.,1.,1.,1.,1.,1.,1.,1.,1.))
REPRESENTATION_ITEM('')
);
#266=(
BOUNDED_CURVE()
B_SPLINE_CURVE(5,(#16441,#16442,#16443,#16444,#16445,#16446,#16447,#16448,
#16449,#16450,#16451,#16452,#16453,#16454,#16455,#16456,#16457,#16458,#16459,
#16460,#16461,#16462,#16463,#16464,#16465,#16466,#16467,#16468,#16469,#16470,
#16471,#16472,#16473,#16474,#16475),.UNSPECIFIED.,.F.,.F.)
B_SPLINE_CURVE_WITH_KNOTS((6,1,1,1,1,1,1,1,1,1,1,1,1,1,1,1,1,1,1,1,1,1,
1,1,1,1,1,1,1,1,6),(0.,0.0333333333333333,0.0666666666666667,0.1,0.133333333333333,
0.166666666666667,0.2,0.233333333333333,0.266666666666667,0.3,0.333333333333333,
0.366666666666667,0.4,0.433333333333333,0.466666666666667,0.5,0.533333333333333,
0.566666666666667,0.6,0.633333333333333,0.666666666666667,0.7,0.733333333333333,
0.766666666666667,0.8,0.833333333333333,0.866666666666667,0.9,0.933333333333333,
0.966666666666667,1.),.UNSPECIFIED.)
CURVE()
GEOMETRIC_REPRESENTATION_ITEM()
RATIONAL_B_SPLINE_CURVE((1.,1.,1.,1.,1.,1.,1.,1.,1.,1.,1.,1.,1.,1.,1.,1.,
1.,1.,1.,1.,1.,1.,1.,1.,1.,1.,1.,1.,1.,1.,1.,1.,1.,1.,1.))
REPRESENTATION_ITEM('')
);
#267=(
BOUNDED_CURVE()
B_SPLINE_CURVE(5,(#16479,#16480,#16481,#16482,#16483,#16484,#16485,#16486,
#16487,#16488,#16489,#16490,#16491,#16492,#16493,#16494,#16495,#16496,#16497,
#16498,#16499,#16500,#16501,#16502,#16503,#16504,#16505,#16506,#16507,#16508,
#16509,#16510,#16511,#16512,#16513),.UNSPECIFIED.,.F.,.F.)
B_SPLINE_CURVE_WITH_KNOTS((6,1,1,1,1,1,1,1,1,1,1,1,1,1,1,1,1,1,1,1,1,1,
1,1,1,1,1,1,1,1,6),(0.,0.0333333333333333,0.0666666666666667,0.1,0.133333333333333,
0.166666666666667,0.2,0.233333333333333,0.266666666666667,0.3,0.333333333333333,
0.366666666666667,0.4,0.433333333333333,0.466666666666667,0.5,0.533333333333333,
0.566666666666667,0.6,0.633333333333333,0.666666666666667,0.7,0.733333333333333,
0.766666666666667,0.8,0.833333333333333,0.866666666666667,0.9,0.933333333333333,
0.966666666666667,1.),.UNSPECIFIED.)
CURVE()
GEOMETRIC_REPRESENTATION_ITEM()
RATIONAL_B_SPLINE_CURVE((1.,1.,1.,1.,1.,1.,1.,1.,1.,1.,1.,1.,1.,1.,1.,1.,
1.,1.,1.,1.,1.,1.,1.,1.,1.,1.,1.,1.,1.,1.,1.,1.,1.,1.,1.))
REPRESENTATION_ITEM('')
);
#268=(
BOUNDED_CURVE()
B_SPLINE_CURVE(5,(#16515,#16516,#16517,#16518,#16519,#16520,#16521,#16522,
#16523,#16524,#16525,#16526,#16527,#16528,#16529,#16530,#16531,#16532,#16533,
#16534,#16535,#16536,#16537,#16538,#16539,#16540,#16541,#16542,#16543,#16544,
#16545,#16546,#16547,#16548,#16549),.UNSPECIFIED.,.F.,.F.)
B_SPLINE_CURVE_WITH_KNOTS((6,1,1,1,1,1,1,1,1,1,1,1,1,1,1,1,1,1,1,1,1,1,
1,1,1,1,1,1,1,1,6),(0.,0.0333333333333333,0.0666666666666667,0.1,0.133333333333333,
0.166666666666667,0.2,0.233333333333333,0.266666666666667,0.3,0.333333333333333,
0.366666666666667,0.4,0.433333333333333,0.466666666666667,0.5,0.533333333333333,
0.566666666666667,0.6,0.633333333333333,0.666666666666667,0.7,0.733333333333333,
0.766666666666667,0.8,0.833333333333333,0.866666666666667,0.9,0.933333333333333,
0.966666666666667,1.),.UNSPECIFIED.)
CURVE()
GEOMETRIC_REPRESENTATION_ITEM()
RATIONAL_B_SPLINE_CURVE((1.,1.,1.,1.,1.,1.,1.,1.,1.,1.,1.,1.,1.,1.,1.,1.,
1.,1.,1.,1.,1.,1.,1.,1.,1.,1.,1.,1.,1.,1.,1.,1.,1.,1.,1.))
REPRESENTATION_ITEM('')
);
#269=(
BOUNDED_CURVE()
B_SPLINE_CURVE(5,(#16553,#16554,#16555,#16556,#16557,#16558,#16559,#16560,
#16561,#16562,#16563,#16564,#16565,#16566,#16567,#16568,#16569,#16570,#16571,
#16572,#16573,#16574,#16575,#16576,#16577,#16578,#16579,#16580,#16581,#16582,
#16583,#16584,#16585,#16586,#16587),.UNSPECIFIED.,.F.,.F.)
B_SPLINE_CURVE_WITH_KNOTS((6,1,1,1,1,1,1,1,1,1,1,1,1,1,1,1,1,1,1,1,1,1,
1,1,1,1,1,1,1,1,6),(0.,0.0333333333333333,0.0666666666666667,0.1,0.133333333333333,
0.166666666666667,0.2,0.233333333333333,0.266666666666667,0.3,0.333333333333333,
0.366666666666667,0.4,0.433333333333333,0.466666666666667,0.5,0.533333333333333,
0.566666666666667,0.6,0.633333333333333,0.666666666666667,0.7,0.733333333333333,
0.766666666666667,0.8,0.833333333333333,0.866666666666667,0.9,0.933333333333333,
0.966666666666667,1.),.UNSPECIFIED.)
CURVE()
GEOMETRIC_REPRESENTATION_ITEM()
RATIONAL_B_SPLINE_CURVE((1.,1.,1.,1.,1.,1.,1.,1.,1.,1.,1.,1.,1.,1.,1.,1.,
1.,1.,1.,1.,1.,1.,1.,1.,1.,1.,1.,1.,1.,1.,1.,1.,1.,1.,1.))
REPRESENTATION_ITEM('')
);
#270=(
BOUNDED_CURVE()
B_SPLINE_CURVE(5,(#16589,#16590,#16591,#16592,#16593,#16594,#16595,#16596,
#16597,#16598,#16599,#16600,#16601,#16602,#16603,#16604,#16605,#16606,#16607,
#16608,#16609,#16610,#16611,#16612,#16613,#16614,#16615,#16616,#16617,#16618,
#16619,#16620,#16621,#16622,#16623),.UNSPECIFIED.,.F.,.F.)
B_SPLINE_CURVE_WITH_KNOTS((6,1,1,1,1,1,1,1,1,1,1,1,1,1,1,1,1,1,1,1,1,1,
1,1,1,1,1,1,1,1,6),(0.,0.0333333333333333,0.0666666666666667,0.1,0.133333333333333,
0.166666666666667,0.2,0.233333333333333,0.266666666666667,0.3,0.333333333333333,
0.366666666666667,0.4,0.433333333333333,0.466666666666667,0.5,0.533333333333333,
0.566666666666667,0.6,0.633333333333333,0.666666666666667,0.7,0.733333333333333,
0.766666666666667,0.8,0.833333333333333,0.866666666666667,0.9,0.933333333333333,
0.966666666666667,1.),.UNSPECIFIED.)
CURVE()
GEOMETRIC_REPRESENTATION_ITEM()
RATIONAL_B_SPLINE_CURVE((1.,1.,1.,1.,1.,1.,1.,1.,1.,1.,1.,1.,1.,1.,1.,1.,
1.,1.,1.,1.,1.,1.,1.,1.,1.,1.,1.,1.,1.,1.,1.,1.,1.,1.,1.))
REPRESENTATION_ITEM('')
);
#271=(
BOUNDED_CURVE()
B_SPLINE_CURVE(5,(#16627,#16628,#16629,#16630,#16631,#16632,#16633,#16634,
#16635,#16636,#16637,#16638,#16639,#16640,#16641,#16642,#16643,#16644,#16645,
#16646,#16647,#16648,#16649,#16650,#16651,#16652,#16653,#16654,#16655,#16656,
#16657,#16658,#16659,#16660,#16661),.UNSPECIFIED.,.F.,.F.)
B_SPLINE_CURVE_WITH_KNOTS((6,1,1,1,1,1,1,1,1,1,1,1,1,1,1,1,1,1,1,1,1,1,
1,1,1,1,1,1,1,1,6),(0.,0.0333333333333333,0.0666666666666667,0.1,0.133333333333333,
0.166666666666667,0.2,0.233333333333333,0.266666666666667,0.3,0.333333333333333,
0.366666666666667,0.4,0.433333333333333,0.466666666666667,0.5,0.533333333333333,
0.566666666666667,0.6,0.633333333333333,0.666666666666667,0.7,0.733333333333333,
0.766666666666667,0.8,0.833333333333333,0.866666666666667,0.9,0.933333333333333,
0.966666666666667,1.),.UNSPECIFIED.)
CURVE()
GEOMETRIC_REPRESENTATION_ITEM()
RATIONAL_B_SPLINE_CURVE((1.,1.,1.,1.,1.,1.,1.,1.,1.,1.,1.,1.,1.,1.,1.,1.,
1.,1.,1.,1.,1.,1.,1.,1.,1.,1.,1.,1.,1.,1.,1.,1.,1.,1.,1.))
REPRESENTATION_ITEM('')
);
#272=(
BOUNDED_CURVE()
B_SPLINE_CURVE(5,(#16663,#16664,#16665,#16666,#16667,#16668,#16669,#16670,
#16671,#16672,#16673,#16674,#16675,#16676,#16677,#16678,#16679,#16680,#16681,
#16682,#16683,#16684,#16685,#16686,#16687,#16688,#16689,#16690,#16691,#16692,
#16693,#16694,#16695,#16696,#16697),.UNSPECIFIED.,.F.,.F.)
B_SPLINE_CURVE_WITH_KNOTS((6,1,1,1,1,1,1,1,1,1,1,1,1,1,1,1,1,1,1,1,1,1,
1,1,1,1,1,1,1,1,6),(0.,0.0333333333333333,0.0666666666666667,0.1,0.133333333333333,
0.166666666666667,0.2,0.233333333333333,0.266666666666667,0.3,0.333333333333333,
0.366666666666667,0.4,0.433333333333333,0.466666666666667,0.5,0.533333333333333,
0.566666666666667,0.6,0.633333333333333,0.666666666666667,0.7,0.733333333333333,
0.766666666666667,0.8,0.833333333333333,0.866666666666667,0.9,0.933333333333333,
0.966666666666667,1.),.UNSPECIFIED.)
CURVE()
GEOMETRIC_REPRESENTATION_ITEM()
RATIONAL_B_SPLINE_CURVE((1.,1.,1.,1.,1.,1.,1.,1.,1.,1.,1.,1.,1.,1.,1.,1.,
1.,1.,1.,1.,1.,1.,1.,1.,1.,1.,1.,1.,1.,1.,1.,1.,1.,1.,1.))
REPRESENTATION_ITEM('')
);
#273=(
BOUNDED_CURVE()
B_SPLINE_CURVE(5,(#16701,#16702,#16703,#16704,#16705,#16706,#16707,#16708,
#16709,#16710,#16711,#16712,#16713,#16714,#16715,#16716,#16717,#16718,#16719,
#16720,#16721,#16722,#16723,#16724,#16725,#16726,#16727,#16728,#16729,#16730,
#16731,#16732,#16733,#16734,#16735),.UNSPECIFIED.,.F.,.F.)
B_SPLINE_CURVE_WITH_KNOTS((6,1,1,1,1,1,1,1,1,1,1,1,1,1,1,1,1,1,1,1,1,1,
1,1,1,1,1,1,1,1,6),(0.,0.0333333333333333,0.0666666666666667,0.1,0.133333333333333,
0.166666666666667,0.2,0.233333333333333,0.266666666666667,0.3,0.333333333333333,
0.366666666666667,0.4,0.433333333333333,0.466666666666667,0.5,0.533333333333333,
0.566666666666667,0.6,0.633333333333333,0.666666666666667,0.7,0.733333333333333,
0.766666666666667,0.8,0.833333333333333,0.866666666666667,0.9,0.933333333333333,
0.966666666666667,1.),.UNSPECIFIED.)
CURVE()
GEOMETRIC_REPRESENTATION_ITEM()
RATIONAL_B_SPLINE_CURVE((1.,1.,1.,1.,1.,1.,1.,1.,1.,1.,1.,1.,1.,1.,1.,1.,
1.,1.,1.,1.,1.,1.,1.,1.,1.,1.,1.,1.,1.,1.,1.,1.,1.,1.,1.))
REPRESENTATION_ITEM('')
);
#274=(
BOUNDED_CURVE()
B_SPLINE_CURVE(5,(#16737,#16738,#16739,#16740,#16741,#16742,#16743,#16744,
#16745,#16746,#16747,#16748,#16749,#16750,#16751,#16752,#16753,#16754,#16755,
#16756,#16757,#16758,#16759,#16760,#16761,#16762,#16763,#16764,#16765,#16766,
#16767,#16768,#16769,#16770,#16771),.UNSPECIFIED.,.F.,.F.)
B_SPLINE_CURVE_WITH_KNOTS((6,1,1,1,1,1,1,1,1,1,1,1,1,1,1,1,1,1,1,1,1,1,
1,1,1,1,1,1,1,1,6),(0.,0.0333333333333333,0.0666666666666667,0.1,0.133333333333333,
0.166666666666667,0.2,0.233333333333333,0.266666666666667,0.3,0.333333333333333,
0.366666666666667,0.4,0.433333333333333,0.466666666666667,0.5,0.533333333333333,
0.566666666666667,0.6,0.633333333333333,0.666666666666667,0.7,0.733333333333333,
0.766666666666667,0.8,0.833333333333333,0.866666666666667,0.9,0.933333333333333,
0.966666666666667,1.),.UNSPECIFIED.)
CURVE()
GEOMETRIC_REPRESENTATION_ITEM()
RATIONAL_B_SPLINE_CURVE((1.,1.,1.,1.,1.,1.,1.,1.,1.,1.,1.,1.,1.,1.,1.,1.,
1.,1.,1.,1.,1.,1.,1.,1.,1.,1.,1.,1.,1.,1.,1.,1.,1.,1.,1.))
REPRESENTATION_ITEM('')
);
#275=(
BOUNDED_CURVE()
B_SPLINE_CURVE(5,(#16775,#16776,#16777,#16778,#16779,#16780,#16781,#16782,
#16783,#16784,#16785,#16786,#16787,#16788,#16789,#16790,#16791,#16792,#16793,
#16794,#16795,#16796,#16797,#16798,#16799,#16800,#16801,#16802,#16803,#16804,
#16805,#16806,#16807,#16808,#16809),.UNSPECIFIED.,.F.,.F.)
B_SPLINE_CURVE_WITH_KNOTS((6,1,1,1,1,1,1,1,1,1,1,1,1,1,1,1,1,1,1,1,1,1,
1,1,1,1,1,1,1,1,6),(0.,0.0333333333333333,0.0666666666666667,0.1,0.133333333333333,
0.166666666666667,0.2,0.233333333333333,0.266666666666667,0.3,0.333333333333333,
0.366666666666667,0.4,0.433333333333333,0.466666666666667,0.5,0.533333333333333,
0.566666666666667,0.6,0.633333333333333,0.666666666666667,0.7,0.733333333333333,
0.766666666666667,0.8,0.833333333333333,0.866666666666667,0.9,0.933333333333333,
0.966666666666667,1.),.UNSPECIFIED.)
CURVE()
GEOMETRIC_REPRESENTATION_ITEM()
RATIONAL_B_SPLINE_CURVE((1.,1.,1.,1.,1.,1.,1.,1.,1.,1.,1.,1.,1.,1.,1.,1.,
1.,1.,1.,1.,1.,1.,1.,1.,1.,1.,1.,1.,1.,1.,1.,1.,1.,1.,1.))
REPRESENTATION_ITEM('')
);
#276=(
BOUNDED_CURVE()
B_SPLINE_CURVE(5,(#16811,#16812,#16813,#16814,#16815,#16816,#16817,#16818,
#16819,#16820,#16821,#16822,#16823,#16824,#16825,#16826,#16827,#16828,#16829,
#16830,#16831,#16832,#16833,#16834,#16835,#16836,#16837,#16838,#16839,#16840,
#16841,#16842,#16843,#16844,#16845),.UNSPECIFIED.,.F.,.F.)
B_SPLINE_CURVE_WITH_KNOTS((6,1,1,1,1,1,1,1,1,1,1,1,1,1,1,1,1,1,1,1,1,1,
1,1,1,1,1,1,1,1,6),(0.,0.0333333333333333,0.0666666666666667,0.1,0.133333333333333,
0.166666666666667,0.2,0.233333333333333,0.266666666666667,0.3,0.333333333333333,
0.366666666666667,0.4,0.433333333333333,0.466666666666667,0.5,0.533333333333333,
0.566666666666667,0.6,0.633333333333333,0.666666666666667,0.7,0.733333333333333,
0.766666666666667,0.8,0.833333333333333,0.866666666666667,0.9,0.933333333333333,
0.966666666666667,1.),.UNSPECIFIED.)
CURVE()
GEOMETRIC_REPRESENTATION_ITEM()
RATIONAL_B_SPLINE_CURVE((1.,1.,1.,1.,1.,1.,1.,1.,1.,1.,1.,1.,1.,1.,1.,1.,
1.,1.,1.,1.,1.,1.,1.,1.,1.,1.,1.,1.,1.,1.,1.,1.,1.,1.,1.))
REPRESENTATION_ITEM('')
);
#277=(
BOUNDED_CURVE()
B_SPLINE_CURVE(5,(#16849,#16850,#16851,#16852,#16853,#16854,#16855,#16856,
#16857,#16858,#16859,#16860,#16861,#16862,#16863,#16864,#16865,#16866,#16867,
#16868,#16869,#16870,#16871,#16872,#16873,#16874,#16875,#16876,#16877,#16878,
#16879,#16880,#16881,#16882,#16883),.UNSPECIFIED.,.F.,.F.)
B_SPLINE_CURVE_WITH_KNOTS((6,1,1,1,1,1,1,1,1,1,1,1,1,1,1,1,1,1,1,1,1,1,
1,1,1,1,1,1,1,1,6),(0.,0.0333333333333333,0.0666666666666667,0.1,0.133333333333333,
0.166666666666667,0.2,0.233333333333333,0.266666666666667,0.3,0.333333333333333,
0.366666666666667,0.4,0.433333333333333,0.466666666666667,0.5,0.533333333333333,
0.566666666666667,0.6,0.633333333333333,0.666666666666667,0.7,0.733333333333333,
0.766666666666667,0.8,0.833333333333333,0.866666666666667,0.9,0.933333333333333,
0.966666666666667,1.),.UNSPECIFIED.)
CURVE()
GEOMETRIC_REPRESENTATION_ITEM()
RATIONAL_B_SPLINE_CURVE((1.,1.,1.,1.,1.,1.,1.,1.,1.,1.,1.,1.,1.,1.,1.,1.,
1.,1.,1.,1.,1.,1.,1.,1.,1.,1.,1.,1.,1.,1.,1.,1.,1.,1.,1.))
REPRESENTATION_ITEM('')
);
#278=(
BOUNDED_CURVE()
B_SPLINE_CURVE(5,(#16885,#16886,#16887,#16888,#16889,#16890,#16891,#16892,
#16893,#16894,#16895,#16896,#16897,#16898,#16899,#16900,#16901,#16902,#16903,
#16904,#16905,#16906,#16907,#16908,#16909,#16910,#16911,#16912,#16913,#16914,
#16915,#16916,#16917,#16918,#16919),.UNSPECIFIED.,.F.,.F.)
B_SPLINE_CURVE_WITH_KNOTS((6,1,1,1,1,1,1,1,1,1,1,1,1,1,1,1,1,1,1,1,1,1,
1,1,1,1,1,1,1,1,6),(0.,0.0333333333333333,0.0666666666666667,0.1,0.133333333333333,
0.166666666666667,0.2,0.233333333333333,0.266666666666667,0.3,0.333333333333333,
0.366666666666667,0.4,0.433333333333333,0.466666666666667,0.5,0.533333333333333,
0.566666666666667,0.6,0.633333333333333,0.666666666666667,0.7,0.733333333333333,
0.766666666666667,0.8,0.833333333333333,0.866666666666667,0.9,0.933333333333333,
0.966666666666667,1.),.UNSPECIFIED.)
CURVE()
GEOMETRIC_REPRESENTATION_ITEM()
RATIONAL_B_SPLINE_CURVE((1.,1.,1.,1.,1.,1.,1.,1.,1.,1.,1.,1.,1.,1.,1.,1.,
1.,1.,1.,1.,1.,1.,1.,1.,1.,1.,1.,1.,1.,1.,1.,1.,1.,1.,1.))
REPRESENTATION_ITEM('')
);
#279=(
BOUNDED_CURVE()
B_SPLINE_CURVE(5,(#16923,#16924,#16925,#16926,#16927,#16928,#16929,#16930,
#16931,#16932,#16933,#16934,#16935,#16936,#16937,#16938,#16939,#16940,#16941,
#16942,#16943,#16944,#16945,#16946,#16947,#16948,#16949,#16950,#16951,#16952,
#16953,#16954,#16955,#16956,#16957),.UNSPECIFIED.,.F.,.F.)
B_SPLINE_CURVE_WITH_KNOTS((6,1,1,1,1,1,1,1,1,1,1,1,1,1,1,1,1,1,1,1,1,1,
1,1,1,1,1,1,1,1,6),(0.,0.0333333333333333,0.0666666666666667,0.1,0.133333333333333,
0.166666666666667,0.2,0.233333333333333,0.266666666666667,0.3,0.333333333333333,
0.366666666666667,0.4,0.433333333333333,0.466666666666667,0.5,0.533333333333333,
0.566666666666667,0.6,0.633333333333333,0.666666666666667,0.7,0.733333333333333,
0.766666666666667,0.8,0.833333333333333,0.866666666666667,0.9,0.933333333333333,
0.966666666666667,1.),.UNSPECIFIED.)
CURVE()
GEOMETRIC_REPRESENTATION_ITEM()
RATIONAL_B_SPLINE_CURVE((1.,1.,1.,1.,1.,1.,1.,1.,1.,1.,1.,1.,1.,1.,1.,1.,
1.,1.,1.,1.,1.,1.,1.,1.,1.,1.,1.,1.,1.,1.,1.,1.,1.,1.,1.))
REPRESENTATION_ITEM('')
);
#280=(
BOUNDED_CURVE()
B_SPLINE_CURVE(5,(#16959,#16960,#16961,#16962,#16963,#16964,#16965,#16966,
#16967,#16968,#16969,#16970,#16971,#16972,#16973,#16974,#16975,#16976,#16977,
#16978,#16979,#16980,#16981,#16982,#16983,#16984,#16985,#16986,#16987,#16988,
#16989,#16990,#16991,#16992,#16993),.UNSPECIFIED.,.F.,.F.)
B_SPLINE_CURVE_WITH_KNOTS((6,1,1,1,1,1,1,1,1,1,1,1,1,1,1,1,1,1,1,1,1,1,
1,1,1,1,1,1,1,1,6),(0.,0.0333333333333333,0.0666666666666667,0.1,0.133333333333333,
0.166666666666667,0.2,0.233333333333333,0.266666666666667,0.3,0.333333333333333,
0.366666666666667,0.4,0.433333333333333,0.466666666666667,0.5,0.533333333333333,
0.566666666666667,0.6,0.633333333333333,0.666666666666667,0.7,0.733333333333333,
0.766666666666667,0.8,0.833333333333333,0.866666666666667,0.9,0.933333333333333,
0.966666666666667,1.),.UNSPECIFIED.)
CURVE()
GEOMETRIC_REPRESENTATION_ITEM()
RATIONAL_B_SPLINE_CURVE((1.,1.,1.,1.,1.,1.,1.,1.,1.,1.,1.,1.,1.,1.,1.,1.,
1.,1.,1.,1.,1.,1.,1.,1.,1.,1.,1.,1.,1.,1.,1.,1.,1.,1.,1.))
REPRESENTATION_ITEM('')
);
#281=(
BOUNDED_CURVE()
B_SPLINE_CURVE(5,(#16997,#16998,#16999,#17000,#17001,#17002,#17003,#17004,
#17005,#17006,#17007,#17008,#17009,#17010,#17011,#17012,#17013,#17014,#17015,
#17016,#17017,#17018,#17019,#17020,#17021,#17022,#17023,#17024,#17025,#17026,
#17027,#17028,#17029,#17030,#17031),.UNSPECIFIED.,.F.,.F.)
B_SPLINE_CURVE_WITH_KNOTS((6,1,1,1,1,1,1,1,1,1,1,1,1,1,1,1,1,1,1,1,1,1,
1,1,1,1,1,1,1,1,6),(0.,0.0333333333333333,0.0666666666666667,0.1,0.133333333333333,
0.166666666666667,0.2,0.233333333333333,0.266666666666667,0.3,0.333333333333333,
0.366666666666667,0.4,0.433333333333333,0.466666666666667,0.5,0.533333333333333,
0.566666666666667,0.6,0.633333333333333,0.666666666666667,0.7,0.733333333333333,
0.766666666666667,0.8,0.833333333333333,0.866666666666667,0.9,0.933333333333333,
0.966666666666667,1.),.UNSPECIFIED.)
CURVE()
GEOMETRIC_REPRESENTATION_ITEM()
RATIONAL_B_SPLINE_CURVE((1.,1.,1.,1.,1.,1.,1.,1.,1.,1.,1.,1.,1.,1.,1.,1.,
1.,1.,1.,1.,1.,1.,1.,1.,1.,1.,1.,1.,1.,1.,1.,1.,1.,1.,1.))
REPRESENTATION_ITEM('')
);
#282=(
BOUNDED_CURVE()
B_SPLINE_CURVE(5,(#17033,#17034,#17035,#17036,#17037,#17038,#17039,#17040,
#17041,#17042,#17043,#17044,#17045,#17046,#17047,#17048,#17049,#17050,#17051,
#17052,#17053,#17054,#17055,#17056,#17057,#17058,#17059,#17060,#17061,#17062,
#17063,#17064,#17065,#17066,#17067),.UNSPECIFIED.,.F.,.F.)
B_SPLINE_CURVE_WITH_KNOTS((6,1,1,1,1,1,1,1,1,1,1,1,1,1,1,1,1,1,1,1,1,1,
1,1,1,1,1,1,1,1,6),(0.,0.0333333333333333,0.0666666666666667,0.1,0.133333333333333,
0.166666666666667,0.2,0.233333333333333,0.266666666666667,0.3,0.333333333333333,
0.366666666666667,0.4,0.433333333333333,0.466666666666667,0.5,0.533333333333333,
0.566666666666667,0.6,0.633333333333333,0.666666666666667,0.7,0.733333333333333,
0.766666666666667,0.8,0.833333333333333,0.866666666666667,0.9,0.933333333333333,
0.966666666666667,1.),.UNSPECIFIED.)
CURVE()
GEOMETRIC_REPRESENTATION_ITEM()
RATIONAL_B_SPLINE_CURVE((1.,1.,1.,1.,1.,1.,1.,1.,1.,1.,1.,1.,1.,1.,1.,1.,
1.,1.,1.,1.,1.,1.,1.,1.,1.,1.,1.,1.,1.,1.,1.,1.,1.,1.,1.))
REPRESENTATION_ITEM('')
);
#283=(
BOUNDED_CURVE()
B_SPLINE_CURVE(5,(#17071,#17072,#17073,#17074,#17075,#17076,#17077,#17078,
#17079,#17080,#17081,#17082,#17083,#17084,#17085,#17086,#17087,#17088,#17089,
#17090,#17091,#17092,#17093,#17094,#17095,#17096,#17097,#17098,#17099,#17100,
#17101,#17102,#17103,#17104,#17105),.UNSPECIFIED.,.F.,.F.)
B_SPLINE_CURVE_WITH_KNOTS((6,1,1,1,1,1,1,1,1,1,1,1,1,1,1,1,1,1,1,1,1,1,
1,1,1,1,1,1,1,1,6),(0.,0.0333333333333333,0.0666666666666667,0.1,0.133333333333333,
0.166666666666667,0.2,0.233333333333333,0.266666666666667,0.3,0.333333333333333,
0.366666666666667,0.4,0.433333333333333,0.466666666666667,0.5,0.533333333333333,
0.566666666666667,0.6,0.633333333333333,0.666666666666667,0.7,0.733333333333333,
0.766666666666667,0.8,0.833333333333333,0.866666666666667,0.9,0.933333333333333,
0.966666666666667,1.),.UNSPECIFIED.)
CURVE()
GEOMETRIC_REPRESENTATION_ITEM()
RATIONAL_B_SPLINE_CURVE((1.,1.,1.,1.,1.,1.,1.,1.,1.,1.,1.,1.,1.,1.,1.,1.,
1.,1.,1.,1.,1.,1.,1.,1.,1.,1.,1.,1.,1.,1.,1.,1.,1.,1.,1.))
REPRESENTATION_ITEM('')
);
#284=(
BOUNDED_CURVE()
B_SPLINE_CURVE(5,(#17107,#17108,#17109,#17110,#17111,#17112,#17113,#17114,
#17115,#17116,#17117,#17118,#17119,#17120,#17121,#17122,#17123,#17124,#17125,
#17126,#17127,#17128,#17129,#17130,#17131,#17132,#17133,#17134,#17135,#17136,
#17137,#17138,#17139,#17140,#17141),.UNSPECIFIED.,.F.,.F.)
B_SPLINE_CURVE_WITH_KNOTS((6,1,1,1,1,1,1,1,1,1,1,1,1,1,1,1,1,1,1,1,1,1,
1,1,1,1,1,1,1,1,6),(0.,0.0333333333333333,0.0666666666666667,0.1,0.133333333333333,
0.166666666666667,0.2,0.233333333333333,0.266666666666667,0.3,0.333333333333333,
0.366666666666667,0.4,0.433333333333333,0.466666666666667,0.5,0.533333333333333,
0.566666666666667,0.6,0.633333333333333,0.666666666666667,0.7,0.733333333333333,
0.766666666666667,0.8,0.833333333333333,0.866666666666667,0.9,0.933333333333333,
0.966666666666667,1.),.UNSPECIFIED.)
CURVE()
GEOMETRIC_REPRESENTATION_ITEM()
RATIONAL_B_SPLINE_CURVE((1.,1.,1.,1.,1.,1.,1.,1.,1.,1.,1.,1.,1.,1.,1.,1.,
1.,1.,1.,1.,1.,1.,1.,1.,1.,1.,1.,1.,1.,1.,1.,1.,1.,1.,1.))
REPRESENTATION_ITEM('')
);
#285=(
BOUNDED_CURVE()
B_SPLINE_CURVE(5,(#17145,#17146,#17147,#17148,#17149,#17150,#17151,#17152,
#17153,#17154,#17155,#17156,#17157,#17158,#17159,#17160,#17161,#17162,#17163,
#17164,#17165,#17166,#17167,#17168,#17169,#17170,#17171,#17172,#17173,#17174,
#17175,#17176,#17177,#17178,#17179),.UNSPECIFIED.,.F.,.F.)
B_SPLINE_CURVE_WITH_KNOTS((6,1,1,1,1,1,1,1,1,1,1,1,1,1,1,1,1,1,1,1,1,1,
1,1,1,1,1,1,1,1,6),(0.,0.0333333333333333,0.0666666666666667,0.1,0.133333333333333,
0.166666666666667,0.2,0.233333333333333,0.266666666666667,0.3,0.333333333333333,
0.366666666666667,0.4,0.433333333333333,0.466666666666667,0.5,0.533333333333333,
0.566666666666667,0.6,0.633333333333333,0.666666666666667,0.7,0.733333333333333,
0.766666666666667,0.8,0.833333333333333,0.866666666666667,0.9,0.933333333333333,
0.966666666666667,1.),.UNSPECIFIED.)
CURVE()
GEOMETRIC_REPRESENTATION_ITEM()
RATIONAL_B_SPLINE_CURVE((1.,1.,1.,1.,1.,1.,1.,1.,1.,1.,1.,1.,1.,1.,1.,1.,
1.,1.,1.,1.,1.,1.,1.,1.,1.,1.,1.,1.,1.,1.,1.,1.,1.,1.,1.))
REPRESENTATION_ITEM('')
);
#286=(
BOUNDED_CURVE()
B_SPLINE_CURVE(5,(#17181,#17182,#17183,#17184,#17185,#17186,#17187,#17188,
#17189,#17190,#17191,#17192,#17193,#17194,#17195,#17196,#17197,#17198,#17199,
#17200,#17201,#17202,#17203,#17204,#17205,#17206,#17207,#17208,#17209,#17210,
#17211,#17212,#17213,#17214,#17215),.UNSPECIFIED.,.F.,.F.)
B_SPLINE_CURVE_WITH_KNOTS((6,1,1,1,1,1,1,1,1,1,1,1,1,1,1,1,1,1,1,1,1,1,
1,1,1,1,1,1,1,1,6),(0.,0.0333333333333333,0.0666666666666667,0.1,0.133333333333333,
0.166666666666667,0.2,0.233333333333333,0.266666666666667,0.3,0.333333333333333,
0.366666666666667,0.4,0.433333333333333,0.466666666666667,0.5,0.533333333333333,
0.566666666666667,0.6,0.633333333333333,0.666666666666667,0.7,0.733333333333333,
0.766666666666667,0.8,0.833333333333333,0.866666666666667,0.9,0.933333333333333,
0.966666666666667,1.),.UNSPECIFIED.)
CURVE()
GEOMETRIC_REPRESENTATION_ITEM()
RATIONAL_B_SPLINE_CURVE((1.,1.,1.,1.,1.,1.,1.,1.,1.,1.,1.,1.,1.,1.,1.,1.,
1.,1.,1.,1.,1.,1.,1.,1.,1.,1.,1.,1.,1.,1.,1.,1.,1.,1.,1.))
REPRESENTATION_ITEM('')
);
#287=(
BOUNDED_CURVE()
B_SPLINE_CURVE(5,(#17219,#17220,#17221,#17222,#17223,#17224,#17225,#17226,
#17227,#17228,#17229,#17230,#17231,#17232,#17233,#17234,#17235,#17236,#17237,
#17238,#17239,#17240,#17241,#17242,#17243,#17244,#17245,#17246,#17247,#17248,
#17249,#17250,#17251,#17252,#17253),.UNSPECIFIED.,.F.,.F.)
B_SPLINE_CURVE_WITH_KNOTS((6,1,1,1,1,1,1,1,1,1,1,1,1,1,1,1,1,1,1,1,1,1,
1,1,1,1,1,1,1,1,6),(0.,0.0333333333333333,0.0666666666666667,0.1,0.133333333333333,
0.166666666666667,0.2,0.233333333333333,0.266666666666667,0.3,0.333333333333333,
0.366666666666667,0.4,0.433333333333333,0.466666666666667,0.5,0.533333333333333,
0.566666666666667,0.6,0.633333333333333,0.666666666666667,0.7,0.733333333333333,
0.766666666666667,0.8,0.833333333333333,0.866666666666667,0.9,0.933333333333333,
0.966666666666667,1.),.UNSPECIFIED.)
CURVE()
GEOMETRIC_REPRESENTATION_ITEM()
RATIONAL_B_SPLINE_CURVE((1.,1.,1.,1.,1.,1.,1.,1.,1.,1.,1.,1.,1.,1.,1.,1.,
1.,1.,1.,1.,1.,1.,1.,1.,1.,1.,1.,1.,1.,1.,1.,1.,1.,1.,1.))
REPRESENTATION_ITEM('')
);
#288=(
BOUNDED_CURVE()
B_SPLINE_CURVE(5,(#17255,#17256,#17257,#17258,#17259,#17260,#17261,#17262,
#17263,#17264,#17265,#17266,#17267,#17268,#17269,#17270,#17271,#17272,#17273,
#17274,#17275,#17276,#17277,#17278,#17279,#17280,#17281,#17282,#17283,#17284,
#17285,#17286,#17287,#17288,#17289),.UNSPECIFIED.,.F.,.F.)
B_SPLINE_CURVE_WITH_KNOTS((6,1,1,1,1,1,1,1,1,1,1,1,1,1,1,1,1,1,1,1,1,1,
1,1,1,1,1,1,1,1,6),(0.,0.0333333333333333,0.0666666666666667,0.1,0.133333333333333,
0.166666666666667,0.2,0.233333333333333,0.266666666666667,0.3,0.333333333333333,
0.366666666666667,0.4,0.433333333333333,0.466666666666667,0.5,0.533333333333333,
0.566666666666667,0.6,0.633333333333333,0.666666666666667,0.7,0.733333333333333,
0.766666666666667,0.8,0.833333333333333,0.866666666666667,0.9,0.933333333333333,
0.966666666666667,1.),.UNSPECIFIED.)
CURVE()
GEOMETRIC_REPRESENTATION_ITEM()
RATIONAL_B_SPLINE_CURVE((1.,1.,1.,1.,1.,1.,1.,1.,1.,1.,1.,1.,1.,1.,1.,1.,
1.,1.,1.,1.,1.,1.,1.,1.,1.,1.,1.,1.,1.,1.,1.,1.,1.,1.,1.))
REPRESENTATION_ITEM('')
);
#289=(
BOUNDED_CURVE()
B_SPLINE_CURVE(5,(#17293,#17294,#17295,#17296,#17297,#17298,#17299,#17300,
#17301,#17302,#17303,#17304,#17305,#17306,#17307,#17308,#17309,#17310,#17311,
#17312,#17313,#17314,#17315,#17316,#17317,#17318,#17319,#17320,#17321,#17322,
#17323,#17324,#17325,#17326,#17327),.UNSPECIFIED.,.F.,.F.)
B_SPLINE_CURVE_WITH_KNOTS((6,1,1,1,1,1,1,1,1,1,1,1,1,1,1,1,1,1,1,1,1,1,
1,1,1,1,1,1,1,1,6),(0.,0.0333333333333333,0.0666666666666667,0.1,0.133333333333333,
0.166666666666667,0.2,0.233333333333333,0.266666666666667,0.3,0.333333333333333,
0.366666666666667,0.4,0.433333333333333,0.466666666666667,0.5,0.533333333333333,
0.566666666666667,0.6,0.633333333333333,0.666666666666667,0.7,0.733333333333333,
0.766666666666667,0.8,0.833333333333333,0.866666666666667,0.9,0.933333333333333,
0.966666666666667,1.),.UNSPECIFIED.)
CURVE()
GEOMETRIC_REPRESENTATION_ITEM()
RATIONAL_B_SPLINE_CURVE((1.,1.,1.,1.,1.,1.,1.,1.,1.,1.,1.,1.,1.,1.,1.,1.,
1.,1.,1.,1.,1.,1.,1.,1.,1.,1.,1.,1.,1.,1.,1.,1.,1.,1.,1.))
REPRESENTATION_ITEM('')
);
#290=(
BOUNDED_CURVE()
B_SPLINE_CURVE(5,(#17329,#17330,#17331,#17332,#17333,#17334,#17335,#17336,
#17337,#17338,#17339,#17340,#17341,#17342,#17343,#17344,#17345,#17346,#17347,
#17348,#17349,#17350,#17351,#17352,#17353,#17354,#17355,#17356,#17357,#17358,
#17359,#17360,#17361,#17362,#17363),.UNSPECIFIED.,.F.,.F.)
B_SPLINE_CURVE_WITH_KNOTS((6,1,1,1,1,1,1,1,1,1,1,1,1,1,1,1,1,1,1,1,1,1,
1,1,1,1,1,1,1,1,6),(0.,0.0333333333333333,0.0666666666666667,0.1,0.133333333333333,
0.166666666666667,0.2,0.233333333333333,0.266666666666667,0.3,0.333333333333333,
0.366666666666667,0.4,0.433333333333333,0.466666666666667,0.5,0.533333333333333,
0.566666666666667,0.6,0.633333333333333,0.666666666666667,0.7,0.733333333333333,
0.766666666666667,0.8,0.833333333333333,0.866666666666667,0.9,0.933333333333333,
0.966666666666667,1.),.UNSPECIFIED.)
CURVE()
GEOMETRIC_REPRESENTATION_ITEM()
RATIONAL_B_SPLINE_CURVE((1.,1.,1.,1.,1.,1.,1.,1.,1.,1.,1.,1.,1.,1.,1.,1.,
1.,1.,1.,1.,1.,1.,1.,1.,1.,1.,1.,1.,1.,1.,1.,1.,1.,1.,1.))
REPRESENTATION_ITEM('')
);
#291=(
BOUNDED_CURVE()
B_SPLINE_CURVE(5,(#17367,#17368,#17369,#17370,#17371,#17372,#17373,#17374,
#17375,#17376,#17377,#17378,#17379,#17380,#17381,#17382,#17383,#17384,#17385,
#17386,#17387,#17388,#17389,#17390,#17391,#17392,#17393,#17394,#17395,#17396,
#17397,#17398,#17399,#17400,#17401),.UNSPECIFIED.,.F.,.F.)
B_SPLINE_CURVE_WITH_KNOTS((6,1,1,1,1,1,1,1,1,1,1,1,1,1,1,1,1,1,1,1,1,1,
1,1,1,1,1,1,1,1,6),(0.,0.0333333333333333,0.0666666666666667,0.1,0.133333333333333,
0.166666666666667,0.2,0.233333333333333,0.266666666666667,0.3,0.333333333333333,
0.366666666666667,0.4,0.433333333333333,0.466666666666667,0.5,0.533333333333333,
0.566666666666667,0.6,0.633333333333333,0.666666666666667,0.7,0.733333333333333,
0.766666666666667,0.8,0.833333333333333,0.866666666666667,0.9,0.933333333333333,
0.966666666666667,1.),.UNSPECIFIED.)
CURVE()
GEOMETRIC_REPRESENTATION_ITEM()
RATIONAL_B_SPLINE_CURVE((1.,1.,1.,1.,1.,1.,1.,1.,1.,1.,1.,1.,1.,1.,1.,1.,
1.,1.,1.,1.,1.,1.,1.,1.,1.,1.,1.,1.,1.,1.,1.,1.,1.,1.,1.))
REPRESENTATION_ITEM('')
);
#292=(
BOUNDED_CURVE()
B_SPLINE_CURVE(5,(#17403,#17404,#17405,#17406,#17407,#17408,#17409,#17410,
#17411,#17412,#17413,#17414,#17415,#17416,#17417,#17418,#17419,#17420,#17421,
#17422,#17423,#17424,#17425,#17426,#17427,#17428,#17429,#17430,#17431,#17432,
#17433,#17434,#17435,#17436,#17437),.UNSPECIFIED.,.F.,.F.)
B_SPLINE_CURVE_WITH_KNOTS((6,1,1,1,1,1,1,1,1,1,1,1,1,1,1,1,1,1,1,1,1,1,
1,1,1,1,1,1,1,1,6),(0.,0.0333333333333333,0.0666666666666667,0.1,0.133333333333333,
0.166666666666667,0.2,0.233333333333333,0.266666666666667,0.3,0.333333333333333,
0.366666666666667,0.4,0.433333333333333,0.466666666666667,0.5,0.533333333333333,
0.566666666666667,0.6,0.633333333333333,0.666666666666667,0.7,0.733333333333333,
0.766666666666667,0.8,0.833333333333333,0.866666666666667,0.9,0.933333333333333,
0.966666666666667,1.),.UNSPECIFIED.)
CURVE()
GEOMETRIC_REPRESENTATION_ITEM()
RATIONAL_B_SPLINE_CURVE((1.,1.,1.,1.,1.,1.,1.,1.,1.,1.,1.,1.,1.,1.,1.,1.,
1.,1.,1.,1.,1.,1.,1.,1.,1.,1.,1.,1.,1.,1.,1.,1.,1.,1.,1.))
REPRESENTATION_ITEM('')
);
#293=(
BOUNDED_CURVE()
B_SPLINE_CURVE(5,(#17441,#17442,#17443,#17444,#17445,#17446,#17447,#17448,
#17449,#17450,#17451,#17452,#17453,#17454,#17455,#17456,#17457,#17458,#17459,
#17460,#17461,#17462,#17463,#17464,#17465,#17466,#17467,#17468,#17469,#17470,
#17471,#17472,#17473,#17474,#17475),.UNSPECIFIED.,.F.,.F.)
B_SPLINE_CURVE_WITH_KNOTS((6,1,1,1,1,1,1,1,1,1,1,1,1,1,1,1,1,1,1,1,1,1,
1,1,1,1,1,1,1,1,6),(0.,0.0333333333333333,0.0666666666666667,0.1,0.133333333333333,
0.166666666666667,0.2,0.233333333333333,0.266666666666667,0.3,0.333333333333333,
0.366666666666667,0.4,0.433333333333333,0.466666666666667,0.5,0.533333333333333,
0.566666666666667,0.6,0.633333333333333,0.666666666666667,0.7,0.733333333333333,
0.766666666666667,0.8,0.833333333333333,0.866666666666667,0.9,0.933333333333333,
0.966666666666667,1.),.UNSPECIFIED.)
CURVE()
GEOMETRIC_REPRESENTATION_ITEM()
RATIONAL_B_SPLINE_CURVE((1.,1.,1.,1.,1.,1.,1.,1.,1.,1.,1.,1.,1.,1.,1.,1.,
1.,1.,1.,1.,1.,1.,1.,1.,1.,1.,1.,1.,1.,1.,1.,1.,1.,1.,1.))
REPRESENTATION_ITEM('')
);
#294=(
BOUNDED_CURVE()
B_SPLINE_CURVE(5,(#17476,#17477,#17478,#17479,#17480,#17481,#17482,#17483,
#17484,#17485,#17486,#17487,#17488,#17489,#17490,#17491,#17492,#17493,#17494,
#17495,#17496,#17497,#17498,#17499,#17500,#17501,#17502,#17503,#17504,#17505,
#17506,#17507,#17508,#17509,#17510),.UNSPECIFIED.,.F.,.F.)
B_SPLINE_CURVE_WITH_KNOTS((6,1,1,1,1,1,1,1,1,1,1,1,1,1,1,1,1,1,1,1,1,1,
1,1,1,1,1,1,1,1,6),(0.,0.0333333333333333,0.0666666666666667,0.1,0.133333333333333,
0.166666666666667,0.2,0.233333333333333,0.266666666666667,0.3,0.333333333333333,
0.366666666666667,0.4,0.433333333333333,0.466666666666667,0.5,0.533333333333333,
0.566666666666667,0.6,0.633333333333333,0.666666666666667,0.7,0.733333333333333,
0.766666666666667,0.8,0.833333333333333,0.866666666666667,0.9,0.933333333333333,
0.966666666666667,1.),.UNSPECIFIED.)
CURVE()
GEOMETRIC_REPRESENTATION_ITEM()
RATIONAL_B_SPLINE_CURVE((1.,1.,1.,1.,1.,1.,1.,1.,1.,1.,1.,1.,1.,1.,1.,1.,
1.,1.,1.,1.,1.,1.,1.,1.,1.,1.,1.,1.,1.,1.,1.,1.,1.,1.,1.))
REPRESENTATION_ITEM('')
);
#295=(
BOUNDED_CURVE()
B_SPLINE_CURVE(5,(#18173,#18174,#18175,#18176,#18177,#18178),
 .UNSPECIFIED.,.F.,.F.)
B_SPLINE_CURVE_WITH_KNOTS((6,6),(0.,0.0167044419729414),.UNSPECIFIED.)
CURVE()
GEOMETRIC_REPRESENTATION_ITEM()
RATIONAL_B_SPLINE_CURVE((1.,1.,1.,1.,1.,1.))
REPRESENTATION_ITEM('')
);
#296=(
BOUNDED_CURVE()
B_SPLINE_CURVE(5,(#18233,#18234,#18235,#18236,#18237,#18238),
 .UNSPECIFIED.,.F.,.F.)
B_SPLINE_CURVE_WITH_KNOTS((6,6),(0.,0.0167044419729412),.UNSPECIFIED.)
CURVE()
GEOMETRIC_REPRESENTATION_ITEM()
RATIONAL_B_SPLINE_CURVE((1.,1.,1.,1.,1.,1.))
REPRESENTATION_ITEM('')
);
#297=(
BOUNDED_CURVE()
B_SPLINE_CURVE(5,(#18293,#18294,#18295,#18296,#18297,#18298),
 .UNSPECIFIED.,.F.,.F.)
B_SPLINE_CURVE_WITH_KNOTS((6,6),(0.,0.016704441972942),.UNSPECIFIED.)
CURVE()
GEOMETRIC_REPRESENTATION_ITEM()
RATIONAL_B_SPLINE_CURVE((1.,1.,1.,1.,1.,1.))
REPRESENTATION_ITEM('')
);
#298=(
BOUNDED_CURVE()
B_SPLINE_CURVE(5,(#18353,#18354,#18355,#18356,#18357,#18358),
 .UNSPECIFIED.,.F.,.F.)
B_SPLINE_CURVE_WITH_KNOTS((6,6),(0.,0.0167044419729414),.UNSPECIFIED.)
CURVE()
GEOMETRIC_REPRESENTATION_ITEM()
RATIONAL_B_SPLINE_CURVE((1.,1.,1.,1.,1.,1.))
REPRESENTATION_ITEM('')
);
#299=(
BOUNDED_CURVE()
B_SPLINE_CURVE(5,(#18413,#18414,#18415,#18416,#18417,#18418),
 .UNSPECIFIED.,.F.,.F.)
B_SPLINE_CURVE_WITH_KNOTS((6,6),(0.,0.0167044419729419),.UNSPECIFIED.)
CURVE()
GEOMETRIC_REPRESENTATION_ITEM()
RATIONAL_B_SPLINE_CURVE((1.,1.,1.,1.,1.,1.))
REPRESENTATION_ITEM('')
);
#300=(
BOUNDED_CURVE()
B_SPLINE_CURVE(5,(#18473,#18474,#18475,#18476,#18477,#18478),
 .UNSPECIFIED.,.F.,.F.)
B_SPLINE_CURVE_WITH_KNOTS((6,6),(0.,0.0167044419729413),.UNSPECIFIED.)
CURVE()
GEOMETRIC_REPRESENTATION_ITEM()
RATIONAL_B_SPLINE_CURVE((1.,1.,1.,1.,1.,1.))
REPRESENTATION_ITEM('')
);
#301=(
BOUNDED_CURVE()
B_SPLINE_CURVE(5,(#18533,#18534,#18535,#18536,#18537,#18538),
 .UNSPECIFIED.,.F.,.F.)
B_SPLINE_CURVE_WITH_KNOTS((6,6),(0.,0.016704441972941),.UNSPECIFIED.)
CURVE()
GEOMETRIC_REPRESENTATION_ITEM()
RATIONAL_B_SPLINE_CURVE((1.,1.,1.,1.,1.,1.))
REPRESENTATION_ITEM('')
);
#302=(
BOUNDED_CURVE()
B_SPLINE_CURVE(5,(#18593,#18594,#18595,#18596,#18597,#18598),
 .UNSPECIFIED.,.F.,.F.)
B_SPLINE_CURVE_WITH_KNOTS((6,6),(0.,0.0167044419729416),.UNSPECIFIED.)
CURVE()
GEOMETRIC_REPRESENTATION_ITEM()
RATIONAL_B_SPLINE_CURVE((1.,1.,1.,1.,1.,1.))
REPRESENTATION_ITEM('')
);
#303=(
BOUNDED_CURVE()
B_SPLINE_CURVE(5,(#18653,#18654,#18655,#18656,#18657,#18658),
 .UNSPECIFIED.,.F.,.F.)
B_SPLINE_CURVE_WITH_KNOTS((6,6),(0.,0.0167044419729408),.UNSPECIFIED.)
CURVE()
GEOMETRIC_REPRESENTATION_ITEM()
RATIONAL_B_SPLINE_CURVE((1.,1.,1.,1.,1.,1.))
REPRESENTATION_ITEM('')
);
#304=(
BOUNDED_CURVE()
B_SPLINE_CURVE(5,(#18713,#18714,#18715,#18716,#18717,#18718),
 .UNSPECIFIED.,.F.,.F.)
B_SPLINE_CURVE_WITH_KNOTS((6,6),(0.,0.0167044419729419),.UNSPECIFIED.)
CURVE()
GEOMETRIC_REPRESENTATION_ITEM()
RATIONAL_B_SPLINE_CURVE((1.,1.,1.,1.,1.,1.))
REPRESENTATION_ITEM('')
);
#305=(
BOUNDED_CURVE()
B_SPLINE_CURVE(5,(#18773,#18774,#18775,#18776,#18777,#18778),
 .UNSPECIFIED.,.F.,.F.)
B_SPLINE_CURVE_WITH_KNOTS((6,6),(0.,0.016704441972942),.UNSPECIFIED.)
CURVE()
GEOMETRIC_REPRESENTATION_ITEM()
RATIONAL_B_SPLINE_CURVE((1.,1.,1.,1.,1.,1.))
REPRESENTATION_ITEM('')
);
#306=(
BOUNDED_CURVE()
B_SPLINE_CURVE(5,(#18833,#18834,#18835,#18836,#18837,#18838),
 .UNSPECIFIED.,.F.,.F.)
B_SPLINE_CURVE_WITH_KNOTS((6,6),(0.,0.016704441972941),.UNSPECIFIED.)
CURVE()
GEOMETRIC_REPRESENTATION_ITEM()
RATIONAL_B_SPLINE_CURVE((1.,1.,1.,1.,1.,1.))
REPRESENTATION_ITEM('')
);
#307=(
BOUNDED_CURVE()
B_SPLINE_CURVE(5,(#18893,#18894,#18895,#18896,#18897,#18898),
 .UNSPECIFIED.,.F.,.F.)
B_SPLINE_CURVE_WITH_KNOTS((6,6),(0.,0.0167044419729416),.UNSPECIFIED.)
CURVE()
GEOMETRIC_REPRESENTATION_ITEM()
RATIONAL_B_SPLINE_CURVE((1.,1.,1.,1.,1.,1.))
REPRESENTATION_ITEM('')
);
#308=(
BOUNDED_CURVE()
B_SPLINE_CURVE(5,(#18953,#18954,#18955,#18956,#18957,#18958),
 .UNSPECIFIED.,.F.,.F.)
B_SPLINE_CURVE_WITH_KNOTS((6,6),(0.,0.0167044419729408),.UNSPECIFIED.)
CURVE()
GEOMETRIC_REPRESENTATION_ITEM()
RATIONAL_B_SPLINE_CURVE((1.,1.,1.,1.,1.,1.))
REPRESENTATION_ITEM('')
);
#309=(
BOUNDED_CURVE()
B_SPLINE_CURVE(5,(#19013,#19014,#19015,#19016,#19017,#19018),
 .UNSPECIFIED.,.F.,.F.)
B_SPLINE_CURVE_WITH_KNOTS((6,6),(0.,0.0167044419729419),.UNSPECIFIED.)
CURVE()
GEOMETRIC_REPRESENTATION_ITEM()
RATIONAL_B_SPLINE_CURVE((1.,1.,1.,1.,1.,1.))
REPRESENTATION_ITEM('')
);
#310=(
BOUNDED_CURVE()
B_SPLINE_CURVE(5,(#19073,#19074,#19075,#19076,#19077,#19078),
 .UNSPECIFIED.,.F.,.F.)
B_SPLINE_CURVE_WITH_KNOTS((6,6),(0.,0.0167044419729415),.UNSPECIFIED.)
CURVE()
GEOMETRIC_REPRESENTATION_ITEM()
RATIONAL_B_SPLINE_CURVE((1.,1.,1.,1.,1.,1.))
REPRESENTATION_ITEM('')
);
#311=(
BOUNDED_CURVE()
B_SPLINE_CURVE(5,(#19133,#19134,#19135,#19136,#19137,#19138),
 .UNSPECIFIED.,.F.,.F.)
B_SPLINE_CURVE_WITH_KNOTS((6,6),(0.,0.0167044419729417),.UNSPECIFIED.)
CURVE()
GEOMETRIC_REPRESENTATION_ITEM()
RATIONAL_B_SPLINE_CURVE((1.,1.,1.,1.,1.,1.))
REPRESENTATION_ITEM('')
);
#312=(
BOUNDED_CURVE()
B_SPLINE_CURVE(5,(#19193,#19194,#19195,#19196,#19197,#19198),
 .UNSPECIFIED.,.F.,.F.)
B_SPLINE_CURVE_WITH_KNOTS((6,6),(0.,0.0167044419729418),.UNSPECIFIED.)
CURVE()
GEOMETRIC_REPRESENTATION_ITEM()
RATIONAL_B_SPLINE_CURVE((1.,1.,1.,1.,1.,1.))
REPRESENTATION_ITEM('')
);
#313=(
BOUNDED_CURVE()
B_SPLINE_CURVE(5,(#19253,#19254,#19255,#19256,#19257,#19258),
 .UNSPECIFIED.,.F.,.F.)
B_SPLINE_CURVE_WITH_KNOTS((6,6),(0.,0.0167044419729408),.UNSPECIFIED.)
CURVE()
GEOMETRIC_REPRESENTATION_ITEM()
RATIONAL_B_SPLINE_CURVE((1.,1.,1.,1.,1.,1.))
REPRESENTATION_ITEM('')
);
#314=(
BOUNDED_CURVE()
B_SPLINE_CURVE(5,(#19313,#19314,#19315,#19316,#19317,#19318),
 .UNSPECIFIED.,.F.,.F.)
B_SPLINE_CURVE_WITH_KNOTS((6,6),(0.,0.0167044419729419),.UNSPECIFIED.)
CURVE()
GEOMETRIC_REPRESENTATION_ITEM()
RATIONAL_B_SPLINE_CURVE((1.,1.,1.,1.,1.,1.))
REPRESENTATION_ITEM('')
);
#315=(
BOUNDED_CURVE()
B_SPLINE_CURVE(5,(#19364,#19365,#19366,#19367,#19368,#19369),
 .UNSPECIFIED.,.F.,.F.)
B_SPLINE_CURVE_WITH_KNOTS((6,6),(0.984324037881896,1.),.UNSPECIFIED.)
CURVE()
GEOMETRIC_REPRESENTATION_ITEM()
RATIONAL_B_SPLINE_CURVE((1.,1.,1.,1.,1.,1.))
REPRESENTATION_ITEM('')
);
#316=(
BOUNDED_CURVE()
B_SPLINE_CURVE(5,(#20018,#20019,#20020,#20021,#20022,#20023),
 .UNSPECIFIED.,.F.,.F.)
B_SPLINE_CURVE_WITH_KNOTS((6,6),(0.984324037881896,1.),.UNSPECIFIED.)
CURVE()
GEOMETRIC_REPRESENTATION_ITEM()
RATIONAL_B_SPLINE_CURVE((1.,1.,1.,1.,1.,1.))
REPRESENTATION_ITEM('')
);
#317=(
BOUNDED_CURVE()
B_SPLINE_CURVE(5,(#20073,#20074,#20075,#20076,#20077,#20078),
 .UNSPECIFIED.,.F.,.F.)
B_SPLINE_CURVE_WITH_KNOTS((6,6),(0.984324037881895,1.),.UNSPECIFIED.)
CURVE()
GEOMETRIC_REPRESENTATION_ITEM()
RATIONAL_B_SPLINE_CURVE((1.,1.,1.,1.,1.,1.))
REPRESENTATION_ITEM('')
);
#318=(
BOUNDED_CURVE()
B_SPLINE_CURVE(5,(#20128,#20129,#20130,#20131,#20132,#20133),
 .UNSPECIFIED.,.F.,.F.)
B_SPLINE_CURVE_WITH_KNOTS((6,6),(0.984324037881896,1.),.UNSPECIFIED.)
CURVE()
GEOMETRIC_REPRESENTATION_ITEM()
RATIONAL_B_SPLINE_CURVE((1.,1.,1.,1.,1.,1.))
REPRESENTATION_ITEM('')
);
#319=(
BOUNDED_CURVE()
B_SPLINE_CURVE(5,(#20179,#20180,#20181,#20182,#20183,#20184),
 .UNSPECIFIED.,.F.,.F.)
B_SPLINE_CURVE_WITH_KNOTS((6,6),(0.984324037881896,1.),.UNSPECIFIED.)
CURVE()
GEOMETRIC_REPRESENTATION_ITEM()
RATIONAL_B_SPLINE_CURVE((1.,1.,1.,1.,1.,1.))
REPRESENTATION_ITEM('')
);
#320=(
BOUNDED_CURVE()
B_SPLINE_CURVE(5,(#20230,#20231,#20232,#20233,#20234,#20235),
 .UNSPECIFIED.,.F.,.F.)
B_SPLINE_CURVE_WITH_KNOTS((6,6),(0.984324037881896,1.),.UNSPECIFIED.)
CURVE()
GEOMETRIC_REPRESENTATION_ITEM()
RATIONAL_B_SPLINE_CURVE((1.,1.,1.,1.,1.,1.))
REPRESENTATION_ITEM('')
);
#321=(
BOUNDED_CURVE()
B_SPLINE_CURVE(5,(#20281,#20282,#20283,#20284,#20285,#20286),
 .UNSPECIFIED.,.F.,.F.)
B_SPLINE_CURVE_WITH_KNOTS((6,6),(0.984324037881896,1.),.UNSPECIFIED.)
CURVE()
GEOMETRIC_REPRESENTATION_ITEM()
RATIONAL_B_SPLINE_CURVE((1.,1.,1.,1.,1.,1.))
REPRESENTATION_ITEM('')
);
#322=(
BOUNDED_CURVE()
B_SPLINE_CURVE(5,(#20336,#20337,#20338,#20339,#20340,#20341),
 .UNSPECIFIED.,.F.,.F.)
B_SPLINE_CURVE_WITH_KNOTS((6,6),(0.984324037881896,1.),.UNSPECIFIED.)
CURVE()
GEOMETRIC_REPRESENTATION_ITEM()
RATIONAL_B_SPLINE_CURVE((1.,1.,1.,1.,1.,1.))
REPRESENTATION_ITEM('')
);
#323=(
BOUNDED_CURVE()
B_SPLINE_CURVE(5,(#20391,#20392,#20393,#20394,#20395,#20396),
 .UNSPECIFIED.,.F.,.F.)
B_SPLINE_CURVE_WITH_KNOTS((6,6),(0.984324037881896,1.),.UNSPECIFIED.)
CURVE()
GEOMETRIC_REPRESENTATION_ITEM()
RATIONAL_B_SPLINE_CURVE((1.,1.,1.,1.,1.,1.))
REPRESENTATION_ITEM('')
);
#324=(
BOUNDED_CURVE()
B_SPLINE_CURVE(5,(#20442,#20443,#20444,#20445,#20446,#20447),
 .UNSPECIFIED.,.F.,.F.)
B_SPLINE_CURVE_WITH_KNOTS((6,6),(0.984324037881896,1.),.UNSPECIFIED.)
CURVE()
GEOMETRIC_REPRESENTATION_ITEM()
RATIONAL_B_SPLINE_CURVE((1.,1.,1.,1.,1.,1.))
REPRESENTATION_ITEM('')
);
#325=(
BOUNDED_CURVE()
B_SPLINE_CURVE(5,(#20493,#20494,#20495,#20496,#20497,#20498),
 .UNSPECIFIED.,.F.,.F.)
B_SPLINE_CURVE_WITH_KNOTS((6,6),(0.984324037881895,1.),.UNSPECIFIED.)
CURVE()
GEOMETRIC_REPRESENTATION_ITEM()
RATIONAL_B_SPLINE_CURVE((1.,1.,1.,1.,1.,1.))
REPRESENTATION_ITEM('')
);
#326=(
BOUNDED_CURVE()
B_SPLINE_CURVE(5,(#20544,#20545,#20546,#20547,#20548,#20549),
 .UNSPECIFIED.,.F.,.F.)
B_SPLINE_CURVE_WITH_KNOTS((6,6),(0.984324037881896,1.),.UNSPECIFIED.)
CURVE()
GEOMETRIC_REPRESENTATION_ITEM()
RATIONAL_B_SPLINE_CURVE((1.,1.,1.,1.,1.,1.))
REPRESENTATION_ITEM('')
);
#327=(
BOUNDED_CURVE()
B_SPLINE_CURVE(5,(#20599,#20600,#20601,#20602,#20603,#20604),
 .UNSPECIFIED.,.F.,.F.)
B_SPLINE_CURVE_WITH_KNOTS((6,6),(0.984324037881896,1.),.UNSPECIFIED.)
CURVE()
GEOMETRIC_REPRESENTATION_ITEM()
RATIONAL_B_SPLINE_CURVE((1.,1.,1.,1.,1.,1.))
REPRESENTATION_ITEM('')
);
#328=(
BOUNDED_CURVE()
B_SPLINE_CURVE(5,(#20654,#20655,#20656,#20657,#20658,#20659),
 .UNSPECIFIED.,.F.,.F.)
B_SPLINE_CURVE_WITH_KNOTS((6,6),(0.984324037881896,1.),.UNSPECIFIED.)
CURVE()
GEOMETRIC_REPRESENTATION_ITEM()
RATIONAL_B_SPLINE_CURVE((1.,1.,1.,1.,1.,1.))
REPRESENTATION_ITEM('')
);
#329=(
BOUNDED_CURVE()
B_SPLINE_CURVE(5,(#20705,#20706,#20707,#20708,#20709,#20710),
 .UNSPECIFIED.,.F.,.F.)
B_SPLINE_CURVE_WITH_KNOTS((6,6),(0.984324037881896,1.),.UNSPECIFIED.)
CURVE()
GEOMETRIC_REPRESENTATION_ITEM()
RATIONAL_B_SPLINE_CURVE((1.,1.,1.,1.,1.,1.))
REPRESENTATION_ITEM('')
);
#330=(
BOUNDED_CURVE()
B_SPLINE_CURVE(5,(#20756,#20757,#20758,#20759,#20760,#20761),
 .UNSPECIFIED.,.F.,.F.)
B_SPLINE_CURVE_WITH_KNOTS((6,6),(0.984324037881896,1.),.UNSPECIFIED.)
CURVE()
GEOMETRIC_REPRESENTATION_ITEM()
RATIONAL_B_SPLINE_CURVE((1.,1.,1.,1.,1.,1.))
REPRESENTATION_ITEM('')
);
#331=(
BOUNDED_CURVE()
B_SPLINE_CURVE(5,(#20807,#20808,#20809,#20810,#20811,#20812),
 .UNSPECIFIED.,.F.,.F.)
B_SPLINE_CURVE_WITH_KNOTS((6,6),(0.984324037881896,1.),.UNSPECIFIED.)
CURVE()
GEOMETRIC_REPRESENTATION_ITEM()
RATIONAL_B_SPLINE_CURVE((1.,1.,1.,1.,1.,1.))
REPRESENTATION_ITEM('')
);
#332=(
BOUNDED_CURVE()
B_SPLINE_CURVE(5,(#20862,#20863,#20864,#20865,#20866,#20867),
 .UNSPECIFIED.,.F.,.F.)
B_SPLINE_CURVE_WITH_KNOTS((6,6),(0.984324037881896,1.),.UNSPECIFIED.)
CURVE()
GEOMETRIC_REPRESENTATION_ITEM()
RATIONAL_B_SPLINE_CURVE((1.,1.,1.,1.,1.,1.))
REPRESENTATION_ITEM('')
);
#333=(
BOUNDED_CURVE()
B_SPLINE_CURVE(5,(#20917,#20918,#20919,#20920,#20921,#20922),
 .UNSPECIFIED.,.F.,.F.)
B_SPLINE_CURVE_WITH_KNOTS((6,6),(0.984324037881896,1.),.UNSPECIFIED.)
CURVE()
GEOMETRIC_REPRESENTATION_ITEM()
RATIONAL_B_SPLINE_CURVE((1.,1.,1.,1.,1.,1.))
REPRESENTATION_ITEM('')
);
#334=(
BOUNDED_CURVE()
B_SPLINE_CURVE(5,(#20968,#20969,#20970,#20971,#20972,#20973),
 .UNSPECIFIED.,.F.,.F.)
B_SPLINE_CURVE_WITH_KNOTS((6,6),(0.984324037881896,1.),.UNSPECIFIED.)
CURVE()
GEOMETRIC_REPRESENTATION_ITEM()
RATIONAL_B_SPLINE_CURVE((1.,1.,1.,1.,1.,1.))
REPRESENTATION_ITEM('')
);
#427=B_SPLINE_CURVE_WITH_KNOTS('',3,(#15846,#15847,#15848,#15849,#15850,
#15851,#15852,#15853,#15854,#15855),.UNSPECIFIED.,.F.,.F.,(4,2,2,2,4),(0.331186461688063,
0.41497096063171,0.498755459575358,0.580564191475742,0.662372923376126),
 .UNSPECIFIED.);
#428=B_SPLINE_CURVE_WITH_KNOTS('',3,(#15857,#15858,#15859,#15860,#15861,
#15862,#15863,#15864,#15865,#15866,#15867,#15868,#15869,#15870,#15871,#15872,
#15873,#15874,#15875),.UNSPECIFIED.,.F.,.F.,(4,2,2,2,3,2,2,2,4),(0.993559385064188,
1.07734388400784,1.16112838295148,1.24293711485187,1.32474584675225,1.40655457865263,
1.48836331055302,1.57214780949667,1.65593230844031),.UNSPECIFIED.);
#429=B_SPLINE_CURVE_WITH_KNOTS('',3,(#15876,#15877,#15878,#15879,#15880,
#15881,#15882,#15883,#15884,#15885),.UNSPECIFIED.,.F.,.F.,(4,2,2,2,4),(0.662372923376126,
0.744181655276509,0.825990387176893,0.909774886120541,0.993559385064188),
 .UNSPECIFIED.);
#430=B_SPLINE_CURVE_WITH_KNOTS('',3,(#15893,#15894,#15895,#15896,#15897,
#15898,#15899,#15900,#15901,#15902),.UNSPECIFIED.,.F.,.F.,(4,2,2,2,4),(0.934777550778115,
1.01265597092338,1.09053439106865,1.1684522293864,1.24637006770415),
 .UNSPECIFIED.);
#431=B_SPLINE_CURVE_WITH_KNOTS('',3,(#15904,#15905,#15906,#15907,#15908,
#15909,#15910,#15911,#15912,#15913,#15914,#15915,#15916,#15917,#15918,#15919,
#15920,#15921),.UNSPECIFIED.,.F.,.F.,(4,2,2,2,2,2,2,2,4),(0.311592516926038,
0.389470937071308,0.467349357216578,0.545267195534327,0.623185033852077,
0.701102872169826,0.779020710487576,0.856899130632846,0.934777550778115),
 .UNSPECIFIED.);
#432=B_SPLINE_CURVE_WITH_KNOTS('',3,(#15922,#15923,#15924,#15925,#15926,
#15927,#15928,#15929,#15930,#15931),.UNSPECIFIED.,.F.,.F.,(4,2,2,2,4),(0.,
0.0779178383177495,0.155835676635499,0.233714096780769,0.311592516926038),
 .UNSPECIFIED.);
#433=B_SPLINE_CURVE_WITH_KNOTS('',3,(#15935,#15936,#15937,#15938,#15939,
#15940,#15941,#15942,#15943,#15944,#15945,#15946,#15947,#15948,#15949,#15950,
#15951,#15952),.UNSPECIFIED.,.F.,.F.,(4,2,2,2,2,2,2,2,4),(0.331186461688063,
0.41497096063171,0.498755459575358,0.580564191475742,0.662372923376126,
0.744181655276509,0.825990387176893,0.909774886120541,0.993559385064188),
 .UNSPECIFIED.);
#434=B_SPLINE_CURVE_WITH_KNOTS('',3,(#15956,#15957,#15958,#15959,#15960,
#15961,#15962,#15963,#15964,#15965,#15966,#15967,#15968,#15969,#15970,#15971,
#15972,#15973,#15974),.UNSPECIFIED.,.F.,.F.,(4,2,2,2,3,2,2,2,4),(0.993559385064188,
1.07734388400784,1.16112838295148,1.24293711485187,1.32474584675225,1.40655457865263,
1.48836331055302,1.57214780949667,1.65593230844031),.UNSPECIFIED.);
#435=B_SPLINE_CURVE_WITH_KNOTS('',3,(#15979,#15980,#15981,#15982,#15983,
#15984,#15985,#15986,#15987,#15988),.UNSPECIFIED.,.F.,.F.,(4,2,2,2,4),(0.,
0.0779178383177495,0.155835676635499,0.233714096780769,0.311592516926038),
 .UNSPECIFIED.);
#436=B_SPLINE_CURVE_WITH_KNOTS('',3,(#15989,#15990,#15991,#15992,#15993,
#15994,#15995,#15996,#15997,#15998,#15999,#16000,#16001,#16002,#16003,#16004,
#16005,#16006,#16007,#16008,#16009,#16010,#16011,#16012,#16013,#16014),
 .UNSPECIFIED.,.F.,.F.,(4,2,2,2,2,2,2,2,2,2,2,2,4),(0.311592516926038,0.389470937071308,
0.467349357216578,0.545267195534327,0.623185033852077,0.701102872169826,
0.779020710487576,0.856899130632846,0.934777550778115,1.01265597092338,
1.09053439106865,1.1684522293864,1.24637006770415),.UNSPECIFIED.);
#437=B_SPLINE_CURVE_WITH_KNOTS('',3,(#17532,#17533,#17534,#17535,#17536,
#17537,#17538,#17539,#17540,#17541,#17542,#17543,#17544,#17545),
 .UNSPECIFIED.,.F.,.F.,(4,2,2,2,2,2,4),(-0.255031134424107,-0.227793077275375,
-0.200453310558795,-0.154190090586012,-0.0736931236043211,-0.0424502065770208,
0.),.UNSPECIFIED.);
#438=B_SPLINE_CURVE_WITH_KNOTS('',3,(#17547,#17548,#17549,#17550,#17551,
#17552,#17553,#17554,#17555,#17556),.UNSPECIFIED.,.F.,.F.,(4,2,2,2,4),(-0.479798392309333,
-0.376300454690274,-0.276804242236344,-0.133663587529964,0.),
 .UNSPECIFIED.);
#439=B_SPLINE_CURVE_WITH_KNOTS('',3,(#17561,#17562,#17563,#17564,#17565,
#17566,#17567,#17568,#17569,#17570,#17571,#17572,#17573,#17574),
 .UNSPECIFIED.,.F.,.F.,(4,2,2,2,2,2,4),(-0.255031134475439,-0.227793077318937,
-0.200453310595062,-0.154190090611401,-0.0736931236137319,-0.0424502065803019,
0.),.UNSPECIFIED.);
#440=B_SPLINE_CURVE_WITH_KNOTS('',3,(#17576,#17577,#17578,#17579,#17580,
#17581,#17582,#17583,#17584,#17585),.UNSPECIFIED.,.F.,.F.,(4,2,2,2,4),(-0.479798392297146,
-0.37630045468042,-0.27680424222853,-0.133663587527001,0.),
 .UNSPECIFIED.);
#441=B_SPLINE_CURVE_WITH_KNOTS('',3,(#17590,#17591,#17592,#17593,#17594,
#17595,#17596,#17597,#17598,#17599,#17600,#17601,#17602,#17603),
 .UNSPECIFIED.,.F.,.F.,(4,2,2,2,2,2,4),(-0.255031134390982,-0.227793077246187,
-0.200453310533645,-0.154190090567835,-0.0736931235979434,-0.0424502065748416,
0.),.UNSPECIFIED.);
#442=B_SPLINE_CURVE_WITH_KNOTS('',3,(#17605,#17606,#17607,#17608,#17609,
#17610,#17611,#17612,#17613,#17614),.UNSPECIFIED.,.F.,.F.,(4,2,2,2,4),(-0.479798392957855,
-0.376300455154524,-0.276804242523407,-0.133663587595138,0.),
 .UNSPECIFIED.);
#443=B_SPLINE_CURVE_WITH_KNOTS('',3,(#17619,#17620,#17621,#17622,#17623,
#17624,#17625,#17626,#17627,#17628,#17629,#17630,#17631,#17632),
 .UNSPECIFIED.,.F.,.F.,(4,2,2,2,2,2,4),(-0.25503113453975,-0.227793077375508,
-0.200453310643473,-0.154190090645765,-0.0736931236262053,-0.042450206584545,
0.),.UNSPECIFIED.);
#444=B_SPLINE_CURVE_WITH_KNOTS('',3,(#17634,#17635,#17636,#17637,#17638,
#17639,#17640,#17641,#17642,#17643),.UNSPECIFIED.,.F.,.F.,(4,2,2,2,4),(-0.4797983929588,
-0.376300455156708,-0.276804242527526,-0.133663587598599,0.),
 .UNSPECIFIED.);
#445=B_SPLINE_CURVE_WITH_KNOTS('',3,(#17648,#17649,#17650,#17651,#17652,
#17653,#17654,#17655,#17656,#17657,#17658,#17659,#17660,#17661),
 .UNSPECIFIED.,.F.,.F.,(4,2,2,2,2,2,4),(-0.255031134416776,-0.227793077270562,
-0.200453310555608,-0.15419009058357,-0.0736931236038192,-0.0424502065768682,
0.),.UNSPECIFIED.);
#446=B_SPLINE_CURVE_WITH_KNOTS('',3,(#17663,#17664,#17665,#17666,#17667,
#17668,#17669,#17670,#17671,#17672),.UNSPECIFIED.,.F.,.F.,(4,2,2,2,4),(-0.479798392586391,
-0.376300454883909,-0.276804242349972,-0.133663587552267,0.),
 .UNSPECIFIED.);
#447=B_SPLINE_CURVE_WITH_KNOTS('',3,(#17677,#17678,#17679,#17680,#17681,
#17682,#17683,#17684,#17685,#17686,#17687,#17688,#17689,#17690),
 .UNSPECIFIED.,.F.,.F.,(4,2,2,2,2,2,4),(-0.255031134441827,-0.227793077287078,
-0.200453310565949,-0.154190090589066,-0.0736931236047745,-0.0424502065771008,
0.),.UNSPECIFIED.);
#448=B_SPLINE_CURVE_WITH_KNOTS('',3,(#17692,#17693,#17694,#17695,#17696,
#17697,#17698,#17699,#17700,#17701),.UNSPECIFIED.,.F.,.F.,(4,2,2,2,4),(-0.479798392309589,
-0.376300454691115,-0.276804242237601,-0.133663587530458,0.),
 .UNSPECIFIED.);
#449=B_SPLINE_CURVE_WITH_KNOTS('',3,(#17706,#17707,#17708,#17709,#17710,
#17711,#17712,#17713,#17714,#17715,#17716,#17717,#17718,#17719),
 .UNSPECIFIED.,.F.,.F.,(4,2,2,2,2,2,4),(-0.255031134477938,-0.227793077321361,
-0.20045331059734,-0.154190090613293,-0.0736931236147239,-0.0424502065806451,
0.),.UNSPECIFIED.);
#450=B_SPLINE_CURVE_WITH_KNOTS('',3,(#17721,#17722,#17723,#17724,#17725,
#17726,#17727,#17728,#17729,#17730),.UNSPECIFIED.,.F.,.F.,(4,2,2,2,4),(-0.479798392040146,
-0.376300454496221,-0.276804242114272,-0.133663587500383,0.),
 .UNSPECIFIED.);
#451=B_SPLINE_CURVE_WITH_KNOTS('',3,(#17735,#17736,#17737,#17738,#17739,
#17740,#17741,#17742,#17743,#17744,#17745,#17746,#17747,#17748),
 .UNSPECIFIED.,.F.,.F.,(4,2,2,2,2,2,4),(-0.255031134491615,-0.227793077335448,
-0.200453310611234,-0.154190090625469,-0.0736931236214063,-0.0424502065831927,
0.),.UNSPECIFIED.);
#452=B_SPLINE_CURVE_WITH_KNOTS('',3,(#17750,#17751,#17752,#17753,#17754,
#17755,#17756,#17757,#17758,#17759),.UNSPECIFIED.,.F.,.F.,(4,2,2,2,4),(-0.479798392731553,
-0.376300454992231,-0.276804242422527,-0.133663587571995,0.),
 .UNSPECIFIED.);
#453=B_SPLINE_CURVE_WITH_KNOTS('',3,(#17764,#17765,#17766,#17767,#17768,
#17769,#17770,#17771,#17772,#17773,#17774,#17775,#17776,#17777),
 .UNSPECIFIED.,.F.,.F.,(4,2,2,2,2,2,4),(-0.255031134337196,-0.227793077196323,
-0.200453310488615,-0.154190090533156,-0.0736931235840354,-0.0424502065698458,
0.),.UNSPECIFIED.);
#454=B_SPLINE_CURVE_WITH_KNOTS('',3,(#17779,#17780,#17781,#17782,#17783,
#17784,#17785,#17786,#17787,#17788),.UNSPECIFIED.,.F.,.F.,(4,2,2,2,4),(-0.479798391697847,
-0.376300454258333,-0.276804241976759,-0.133663587475283,0.),
 .UNSPECIFIED.);
#455=B_SPLINE_CURVE_WITH_KNOTS('',3,(#17793,#17794,#17795,#17796,#17797,
#17798,#17799,#17800,#17801,#17802,#17803,#17804,#17805,#17806),
 .UNSPECIFIED.,.F.,.F.,(4,2,2,2,2,2,4),(-0.255031134300382,-0.227793077166129,
-0.200453310466903,-0.154190090528462,-0.0736931235865039,-0.0424502065710793,
0.),.UNSPECIFIED.);
#456=B_SPLINE_CURVE_WITH_KNOTS('',3,(#17808,#17809,#17810,#17811,#17812,
#17813,#17814,#17815,#17816,#17817),.UNSPECIFIED.,.F.,.F.,(4,2,2,2,4),(-0.479798391515407,
-0.376300454120398,-0.276804241882046,-0.133663587447611,0.),
 .UNSPECIFIED.);
#457=B_SPLINE_CURVE_WITH_KNOTS('',3,(#17822,#17823,#17824,#17825,#17826,
#17827,#17828,#17829,#17830,#17831,#17832,#17833,#17834,#17835),
 .UNSPECIFIED.,.F.,.F.,(4,2,2,2,2,2,4),(-0.255031134433992,-0.227793077286409,
-0.200453310570116,-0.154190090595771,-0.0736931236079108,-0.0424502065782311,
0.),.UNSPECIFIED.);
#458=B_SPLINE_CURVE_WITH_KNOTS('',3,(#17837,#17838,#17839,#17840,#17841,
#17842,#17843,#17844,#17845,#17846),.UNSPECIFIED.,.F.,.F.,(4,2,2,2,4),(-0.479798392302676,
-0.376300454686334,-0.276804242234968,-0.133663587529961,0.),
 .UNSPECIFIED.);
#459=B_SPLINE_CURVE_WITH_KNOTS('',3,(#17851,#17852,#17853,#17854,#17855,
#17856,#17857,#17858,#17859,#17860,#17861,#17862,#17863,#17864),
 .UNSPECIFIED.,.F.,.F.,(4,2,2,2,2,2,4),(-0.255031134436975,-0.227793077286682,
-0.200453310569877,-0.154190090598983,-0.0736931236101461,-0.0424502065791056,
0.),.UNSPECIFIED.);
#460=B_SPLINE_CURVE_WITH_KNOTS('',3,(#17866,#17867,#17868,#17869,#17870,
#17871,#17872,#17873,#17874,#17875),.UNSPECIFIED.,.F.,.F.,(4,2,2,2,4),(-0.479798392050366,
-0.37630045450428,-0.276804242120537,-0.133663587502534,0.),
 .UNSPECIFIED.);
#461=B_SPLINE_CURVE_WITH_KNOTS('',3,(#17880,#17881,#17882,#17883,#17884,
#17885,#17886,#17887,#17888,#17889,#17890,#17891,#17892,#17893),
 .UNSPECIFIED.,.F.,.F.,(4,2,2,2,2,2,4),(-0.255031134555854,-0.227793077394919,
-0.200453310664611,-0.154190090665751,-0.0736931236342781,-0.0424502065874606,
0.),.UNSPECIFIED.);
#462=B_SPLINE_CURVE_WITH_KNOTS('',3,(#17895,#17896,#17897,#17898,#17899,
#17900,#17901,#17902,#17903,#17904),.UNSPECIFIED.,.F.,.F.,(4,2,2,2,4),(-0.479798392574118,
-0.376300454878286,-0.276804242350487,-0.133663587555216,0.),
 .UNSPECIFIED.);
#463=B_SPLINE_CURVE_WITH_KNOTS('',3,(#17909,#17910,#17911,#17912,#17913,
#17914,#17915,#17916,#17917,#17918,#17919,#17920,#17921,#17922),
 .UNSPECIFIED.,.F.,.F.,(4,2,2,2,2,2,4),(-0.255031134589258,-0.227793077418444,
-0.200453310681013,-0.154190090675844,-0.0736931236365812,-0.042450206588134,
0.),.UNSPECIFIED.);
#464=B_SPLINE_CURVE_WITH_KNOTS('',3,(#17924,#17925,#17926,#17927,#17928,
#17929,#17930,#17931,#17932,#17933),.UNSPECIFIED.,.F.,.F.,(4,2,2,2,4),(-0.479798391705042,
-0.376300454262635,-0.276804241978204,-0.13366358747526,0.),
 .UNSPECIFIED.);
#465=B_SPLINE_CURVE_WITH_KNOTS('',3,(#17938,#17939,#17940,#17941,#17942,
#17943,#17944,#17945,#17946,#17947,#17948,#17949,#17950,#17951),
 .UNSPECIFIED.,.F.,.F.,(4,2,2,2,2,2,4),(-0.255031134410801,-0.227793077261618,
-0.200453310546074,-0.154190090578359,-0.0736931236015757,-0.0424502065760304,
0.),.UNSPECIFIED.);
#466=B_SPLINE_CURVE_WITH_KNOTS('',3,(#17953,#17954,#17955,#17956,#17957,
#17958,#17959,#17960,#17961,#17962),.UNSPECIFIED.,.F.,.F.,(4,2,2,2,4),(-0.47979839227541,
-0.376300454666073,-0.27680424222116,-0.133663587524637,0.),
 .UNSPECIFIED.);
#467=B_SPLINE_CURVE_WITH_KNOTS('',3,(#17967,#17968,#17969,#17970,#17971,
#17972,#17973,#17974,#17975,#17976,#17977,#17978,#17979,#17980),
 .UNSPECIFIED.,.F.,.F.,(4,2,2,2,2,2,4),(-0.255031134458131,-0.227793077304459,
-0.200453310582776,-0.154190090601721,-0.0736931236097356,-0.0424502065788514,
0.),.UNSPECIFIED.);
#468=B_SPLINE_CURVE_WITH_KNOTS('',3,(#17982,#17983,#17984,#17985,#17986,
#17987,#17988,#17989,#17990,#17991),.UNSPECIFIED.,.F.,.F.,(4,2,2,2,4),(-0.479798392316289,
-0.37630045469605,-0.276804242240997,-0.133663587531333,0.),
 .UNSPECIFIED.);
#469=B_SPLINE_CURVE_WITH_KNOTS('',3,(#17996,#17997,#17998,#17999,#18000,
#18001,#18002,#18003,#18004,#18005,#18006,#18007,#18008,#18009),
 .UNSPECIFIED.,.F.,.F.,(4,2,2,2,2,2,4),(-0.255031134442356,-0.227793077291177,
-0.200453310572288,-0.154190090596086,-0.0736931236086164,-0.0424502065785607,
0.),.UNSPECIFIED.);
#470=B_SPLINE_CURVE_WITH_KNOTS('',3,(#18011,#18012,#18013,#18014,#18015,
#18016,#18017,#18018,#18019,#18020),.UNSPECIFIED.,.F.,.F.,(4,2,2,2,4),(-0.479798392585983,
-0.37630045488836,-0.276804242358604,-0.133663587557499,0.),
 .UNSPECIFIED.);
#471=B_SPLINE_CURVE_WITH_KNOTS('',3,(#18025,#18026,#18027,#18028,#18029,
#18030,#18031,#18032,#18033,#18034,#18035,#18036,#18037,#18038),
 .UNSPECIFIED.,.F.,.F.,(4,2,2,2,2,2,4),(-0.255031134477192,-0.227793077319635,
-0.200453310596239,-0.154190090616096,-0.0736931236157987,-0.0424502065810278,
0.),.UNSPECIFIED.);
#472=B_SPLINE_CURVE_WITH_KNOTS('',3,(#18040,#18041,#18042,#18043,#18044,
#18045,#18046,#18047,#18048,#18049),.UNSPECIFIED.,.F.,.F.,(4,2,2,2,4),(-0.479798392969913,
-0.376300455164432,-0.276804242530612,-0.133663587597497,0.),
 .UNSPECIFIED.);
#473=B_SPLINE_CURVE_WITH_KNOTS('',3,(#18054,#18055,#18056,#18057,#18058,
#18059,#18060,#18061,#18062,#18063,#18064,#18065,#18066,#18067),
 .UNSPECIFIED.,.F.,.F.,(4,2,2,2,2,2,4),(-0.255031134454417,-0.227793077300734,
-0.200453310579618,-0.154190090600756,-0.0736931236102396,-0.0424502065790721,
0.),.UNSPECIFIED.);
#474=B_SPLINE_CURVE_WITH_KNOTS('',3,(#18069,#18070,#18071,#18072,#18073,
#18074,#18075,#18076,#18077,#18078),.UNSPECIFIED.,.F.,.F.,(4,2,2,2,4),(-0.479798391685298,
-0.376300454251086,-0.276804241974231,-0.13366358747526,0.),
 .UNSPECIFIED.);
#475=B_SPLINE_CURVE_WITH_KNOTS('',3,(#18093,#18094,#18095,#18096,#18097,
#18098,#18099,#18100,#18101,#18102,#18103,#18104,#18105,#18106),
 .UNSPECIFIED.,.F.,.F.,(4,2,2,2,2,2,4),(-0.255031134441405,-0.227793077289669,
-0.200453310571579,-0.154190090599269,-0.073693123610816,-0.0424502065793788,
0.),.UNSPECIFIED.);
#476=B_SPLINE_CURVE_WITH_KNOTS('',3,(#18108,#18109,#18110,#18111,#18112,
#18113,#18114,#18115,#18116,#18117),.UNSPECIFIED.,.F.,.F.,(4,2,2,2,4),(-0.47979839202925,
-0.37630045448809,-0.276804242109191,-0.13366358749908,0.),
 .UNSPECIFIED.);
#477=B_SPLINE_CURVE_WITH_KNOTS('',3,(#18145,#18146,#18147,#18148,#18149,
#18150,#18151,#18152,#18153,#18154,#18155,#18156,#18157,#18158,#18159,#18160,
#18161,#18162,#18163,#18164,#18165,#18166,#18167,#18168,#18169,#18170,#18171,
#18172),.UNSPECIFIED.,.F.,.F.,(4,3,3,3,3,3,3,3,3,4),(0.,0.10419502125344,
0.208837694316349,0.315309080210678,0.394143302470623,0.474642117912927,
0.555269967633744,0.636143661419361,0.718213150424091,0.797153516796196),
 .UNSPECIFIED.);
#478=B_SPLINE_CURVE_WITH_KNOTS('',3,(#18205,#18206,#18207,#18208,#18209,
#18210,#18211,#18212,#18213,#18214,#18215,#18216,#18217,#18218,#18219,#18220,
#18221,#18222,#18223,#18224,#18225,#18226,#18227,#18228,#18229,#18230,#18231,
#18232),.UNSPECIFIED.,.F.,.F.,(4,3,3,3,3,3,3,3,3,4),(0.,0.104195149650902,
0.208837865524772,0.315309089419264,0.394143302470425,0.474642042092398,
0.555269910768279,0.636143270035123,0.718211827223173,0.797153516795923),
 .UNSPECIFIED.);
#479=B_SPLINE_CURVE_WITH_KNOTS('',3,(#18265,#18266,#18267,#18268,#18269,
#18270,#18271,#18272,#18273,#18274,#18275,#18276,#18277,#18278,#18279,#18280,
#18281,#18282,#18283,#18284,#18285,#18286,#18287,#18288,#18289,#18290,#18291,
#18292),.UNSPECIFIED.,.F.,.F.,(4,3,3,3,3,3,3,3,3,4),(0.,0.104195119607756,
0.208837825459222,0.315309087260799,0.394143302470401,0.474642059835697,
0.555269924075725,0.636143361633792,0.718212136889593,0.797153516795811),
 .UNSPECIFIED.);
#480=B_SPLINE_CURVE_WITH_KNOTS('',3,(#18325,#18326,#18327,#18328,#18329,
#18330,#18331,#18332,#18333,#18334,#18335,#18336,#18337,#18338,#18339,#18340,
#18341,#18342,#18343,#18344,#18345,#18346,#18347,#18348,#18349,#18350,#18351,
#18352),.UNSPECIFIED.,.F.,.F.,(4,3,3,3,3,3,3,3,3,4),(0.,0.104194925859371,
0.208837567155458,0.315309073394225,0.394143302470344,0.474642174225039,
0.555270009867713,0.636143952047701,0.718214133082137,0.797153516795737),
 .UNSPECIFIED.);
#481=B_SPLINE_CURVE_WITH_KNOTS('',3,(#18385,#18386,#18387,#18388,#18389,
#18390,#18391,#18392,#18393,#18394,#18395,#18396,#18397,#18398,#18399,#18400,
#18401,#18402,#18403,#18404,#18405,#18406,#18407,#18408,#18409,#18410,#18411,
#18412),.UNSPECIFIED.,.F.,.F.,(4,3,3,3,3,3,3,3,3,4),(0.,0.104194711471012,
0.208837281501618,0.315309058162189,0.394143302470344,0.47464230072316,
0.555270104741296,0.636144604731537,0.71821634019969,0.797153516795704),
 .UNSPECIFIED.);
#482=B_SPLINE_CURVE_WITH_KNOTS('',3,(#18445,#18446,#18447,#18448,#18449,
#18450,#18451,#18452,#18453,#18454,#18455,#18456,#18457,#18458,#18459,#18460,
#18461,#18462,#18463,#18464,#18465,#18466,#18467,#18468,#18469,#18470,#18471,
#18472),.UNSPECIFIED.,.F.,.F.,(4,3,3,3,3,3,3,3,3,4),(0.,0.104195021253205,
0.208837694315724,0.315309080210004,0.394143302470563,0.474642117912995,
0.555269967633764,0.636143661419282,0.718213150423912,0.797153516796073),
 .UNSPECIFIED.);
#483=B_SPLINE_CURVE_WITH_KNOTS('',3,(#18505,#18506,#18507,#18508,#18509,
#18510,#18511,#18512,#18513,#18514,#18515,#18516,#18517,#18518,#18519,#18520,
#18521,#18522,#18523,#18524,#18525,#18526,#18527,#18528,#18529,#18530,#18531,
#18532),.UNSPECIFIED.,.F.,.F.,(4,3,3,3,3,3,3,3,3,4),(0.,0.104195149651105,
0.208837865524873,0.315309089419088,0.394143302470483,0.474642042092258,
0.555269910768202,0.636143270034896,0.718211827223,0.797153516796034),
 .UNSPECIFIED.);
#484=B_SPLINE_CURVE_WITH_KNOTS('',3,(#18565,#18566,#18567,#18568,#18569,
#18570,#18571,#18572,#18573,#18574,#18575,#18576,#18577,#18578,#18579,#18580,
#18581,#18582,#18583,#18584,#18585,#18586,#18587,#18588,#18589,#18590,#18591,
#18592),.UNSPECIFIED.,.F.,.F.,(4,3,3,3,3,3,3,3,3,4),(0.,0.104195119607856,
0.208837825459762,0.315309087261884,0.394143302470623,0.474642059835987,
0.555269924076029,0.636143361634067,0.718212136889809,0.797153516796157),
 .UNSPECIFIED.);
#485=B_SPLINE_CURVE_WITH_KNOTS('',3,(#18625,#18626,#18627,#18628,#18629,
#18630,#18631,#18632,#18633,#18634,#18635,#18636,#18637,#18638,#18639,#18640,
#18641,#18642,#18643,#18644,#18645,#18646,#18647,#18648,#18649,#18650,#18651,
#18652),.UNSPECIFIED.,.F.,.F.,(4,3,3,3,3,3,3,3,3,4),(0.,0.104194925859672,
0.208837567155869,0.31530907339494,0.394143302470401,0.474642174225063,
0.555270009867749,0.636143952047726,0.71821413308218,0.797153516795805),
 .UNSPECIFIED.);
#486=B_SPLINE_CURVE_WITH_KNOTS('',3,(#18685,#18686,#18687,#18688,#18689,
#18690,#18691,#18692,#18693,#18694,#18695,#18696,#18697,#18698,#18699,#18700,
#18701,#18702,#18703,#18704,#18705,#18706,#18707,#18708,#18709,#18710,#18711,
#18712),.UNSPECIFIED.,.F.,.F.,(4,3,3,3,3,3,3,3,3,4),(0.,0.104194711471136,
0.208837281501506,0.315309058162058,0.394143302470353,0.474642300722815,
0.555270104741049,0.636144604731284,0.718216340199488,0.797153516795751),
 .UNSPECIFIED.);
#487=B_SPLINE_CURVE_WITH_KNOTS('',3,(#18745,#18746,#18747,#18748,#18749,
#18750,#18751,#18752,#18753,#18754,#18755,#18756,#18757,#18758,#18759,#18760,
#18761,#18762,#18763,#18764,#18765,#18766,#18767,#18768,#18769,#18770,#18771,
#18772),.UNSPECIFIED.,.F.,.F.,(4,3,3,3,3,3,3,3,3,4),(0.,0.104195021253541,
0.208837694316027,0.315309080210591,0.394143302470527,0.474642117912781,
0.555269967633599,0.636143661419217,0.718213150423855,0.797153516796053),
 .UNSPECIFIED.);
#488=B_SPLINE_CURVE_WITH_KNOTS('',3,(#18805,#18806,#18807,#18808,#18809,
#18810,#18811,#18812,#18813,#18814,#18815,#18816,#18817,#18818,#18819,#18820,
#18821,#18822,#18823,#18824,#18825,#18826,#18827,#18828,#18829,#18830,#18831,
#18832),.UNSPECIFIED.,.F.,.F.,(4,3,3,3,3,3,3,3,3,4),(0.,0.104195149650553,
0.208837865524795,0.315309089419618,0.394143302470498,0.474642042092278,
0.555269910768226,0.636143270034951,0.718211827223001,0.797153516796067),
 .UNSPECIFIED.);
#489=B_SPLINE_CURVE_WITH_KNOTS('',3,(#18865,#18866,#18867,#18868,#18869,
#18870,#18871,#18872,#18873,#18874,#18875,#18876,#18877,#18878,#18879,#18880,
#18881,#18882,#18883,#18884,#18885,#18886,#18887,#18888,#18889,#18890,#18891,
#18892),.UNSPECIFIED.,.F.,.F.,(4,3,3,3,3,3,3,3,3,4),(0.,0.104195119607818,
0.208837825459189,0.315309087261459,0.394143302470449,0.474642059835694,
0.555269924075731,0.636143361633688,0.718212136889352,0.797153516795842),
 .UNSPECIFIED.);
#490=B_SPLINE_CURVE_WITH_KNOTS('',3,(#18925,#18926,#18927,#18928,#18929,
#18930,#18931,#18932,#18933,#18934,#18935,#18936,#18937,#18938,#18939,#18940,
#18941,#18942,#18943,#18944,#18945,#18946,#18947,#18948,#18949,#18950,#18951,
#18952),.UNSPECIFIED.,.F.,.F.,(4,3,3,3,3,3,3,3,3,4),(0.,0.104194925859784,
0.208837567155939,0.31530907339513,0.394143302470471,0.474642174225348,
0.555270009867996,0.636143952047895,0.718214133082319,0.797153516795942),
 .UNSPECIFIED.);
#491=B_SPLINE_CURVE_WITH_KNOTS('',3,(#18985,#18986,#18987,#18988,#18989,
#18990,#18991,#18992,#18993,#18994,#18995,#18996,#18997,#18998,#18999,#19000,
#19001,#19002,#19003,#19004,#19005,#19006,#19007,#19008,#19009,#19010,#19011,
#19012),.UNSPECIFIED.,.F.,.F.,(4,3,3,3,3,3,3,3,3,4),(0.,0.104194711471186,
0.208837281501366,0.315309058162388,0.394143302470451,0.474642300723038,
0.555270104741255,0.636144604731555,0.718216340199711,0.797153516795907),
 .UNSPECIFIED.);
#492=B_SPLINE_CURVE_WITH_KNOTS('',3,(#19045,#19046,#19047,#19048,#19049,
#19050,#19051,#19052,#19053,#19054,#19055,#19056,#19057,#19058,#19059,#19060,
#19061,#19062,#19063,#19064,#19065,#19066,#19067,#19068,#19069,#19070,#19071,
#19072),.UNSPECIFIED.,.F.,.F.,(4,3,3,3,3,3,3,3,3,4),(0.,0.104195021253042,
0.208837694315628,0.315309080210067,0.394143302470476,0.474642117912826,
0.55526996763361,0.636143661419199,0.718213150423859,0.797153516795962),
 .UNSPECIFIED.);
#493=B_SPLINE_CURVE_WITH_KNOTS('',3,(#19105,#19106,#19107,#19108,#19109,
#19110,#19111,#19112,#19113,#19114,#19115,#19116,#19117,#19118,#19119,#19120,
#19121,#19122,#19123,#19124,#19125,#19126,#19127,#19128,#19129,#19130,#19131,
#19132),.UNSPECIFIED.,.F.,.F.,(4,3,3,3,3,3,3,3,3,4),(0.,0.104195149650775,
0.208837865524784,0.315309089419042,0.394143302470323,0.474642042092065,
0.555269910767973,0.636143270034795,0.71821182722283,0.797153516795697),
 .UNSPECIFIED.);
#494=B_SPLINE_CURVE_WITH_KNOTS('',3,(#19165,#19166,#19167,#19168,#19169,
#19170,#19171,#19172,#19173,#19174,#19175,#19176,#19177,#19178,#19179,#19180,
#19181,#19182,#19183,#19184,#19185,#19186,#19187,#19188,#19189,#19190,#19191,
#19192),.UNSPECIFIED.,.F.,.F.,(4,3,3,3,3,3,3,3,3,4),(0.,0.104195119607863,
0.208837825459412,0.31530908726121,0.394143302470542,0.474642059835598,
0.555269924075699,0.63614336163368,0.718212136889433,0.797153516796002),
 .UNSPECIFIED.);
#495=B_SPLINE_CURVE_WITH_KNOTS('',3,(#19225,#19226,#19227,#19228,#19229,
#19230,#19231,#19232,#19233,#19234,#19235,#19236,#19237,#19238,#19239,#19240,
#19241,#19242,#19243,#19244,#19245,#19246,#19247,#19248,#19249,#19250,#19251,
#19252),.UNSPECIFIED.,.F.,.F.,(4,3,3,3,3,3,3,3,3,4),(0.,0.104194925859466,
0.208837567155331,0.315309073394099,0.394143302470382,0.474642174224968,
0.555270009867677,0.636143952047661,0.718214133082044,0.797153516795802),
 .UNSPECIFIED.);
#496=B_SPLINE_CURVE_WITH_KNOTS('',3,(#19285,#19286,#19287,#19288,#19289,
#19290,#19291,#19292,#19293,#19294,#19295,#19296,#19297,#19298,#19299,#19300,
#19301,#19302,#19303,#19304,#19305,#19306,#19307,#19308,#19309,#19310,#19311,
#19312),.UNSPECIFIED.,.F.,.F.,(4,3,3,3,3,3,3,3,3,4),(0.,0.104194711470983,
0.208837281501467,0.315309058162056,0.394143302470363,0.474642300723069,
0.555270104741244,0.636144604731482,0.718216340199667,0.797153516795768),
 .UNSPECIFIED.);
#497=B_SPLINE_CURVE_WITH_KNOTS('',3,(#19370,#19371,#19372,#19373,#19374,
#19375,#19376,#19377,#19378,#19379,#19380,#19381,#19382,#19383,#19384,#19385,
#19386,#19387,#19388,#19389,#19390,#19391,#19392,#19393,#19394,#19395,#19396,
#19397),.UNSPECIFIED.,.F.,.F.,(4,3,3,3,3,3,3,3,3,4),(0.,0.0913693045581491,
0.175304752632241,0.256829545365516,0.336180776983803,0.39678509935003,
0.504865678023162,0.611029081983863,0.715415587626191,0.795801737615653),
 .UNSPECIFIED.);
#498=B_SPLINE_CURVE_WITH_KNOTS('',3,(#19405,#19406,#19407,#19408,#19409,
#19410,#19411,#19412,#19413,#19414,#19415,#19416,#19417,#19418,#19419,#19420,
#19421,#19422,#19423,#19424,#19425,#19426,#19427,#19428,#19429,#19430,#19431,
#19432),.UNSPECIFIED.,.F.,.F.,(4,3,3,3,3,3,3,3,3,4),(0.,0.091300847639123,
0.17522519587234,0.256743850114013,0.336091868063455,0.396785099350019,
0.50484847748811,0.610985103772719,0.715329935719015,0.795801737615632),
 .UNSPECIFIED.);
#499=B_SPLINE_CURVE_WITH_KNOTS('',3,(#19435,#19436,#19437,#19438,#19439,
#19440,#19441,#19442,#19443,#19444,#19445,#19446,#19447,#19448,#19449,#19450,
#19451,#19452,#19453,#19454,#19455,#19456,#19457,#19458,#19459,#19460,#19461,
#19462),.UNSPECIFIED.,.F.,.F.,(4,3,3,3,3,3,3,3,3,4),(0.,0.0913055244675908,
0.175231740459174,0.256751333955076,0.336099680903453,0.396785099350007,
0.504849076375648,0.610985832253314,0.715329675493193,0.795801737615589),
 .UNSPECIFIED.);
#500=B_SPLINE_CURVE_WITH_KNOTS('',3,(#19465,#19466,#19467,#19468,#19469,
#19470,#19471,#19472,#19473,#19474,#19475,#19476,#19477,#19478,#19479,#19480,
#19481,#19482,#19483,#19484,#19485,#19486,#19487,#19488,#19489,#19490,#19491,
#19492),.UNSPECIFIED.,.F.,.F.,(4,3,3,3,3,3,3,3,3,4),(0.,0.0913671480398549,
0.1753017609357,0.256826133349693,0.336177213290906,0.396785099349999,0.504865390200783,
0.611028723085786,0.71541568566786,0.795801737615528),.UNSPECIFIED.);
#501=B_SPLINE_CURVE_WITH_KNOTS('',3,(#19495,#19496,#19497,#19498,#19499,
#19500,#19501,#19502,#19503,#19504,#19505,#19506,#19507,#19508,#19509,#19510,
#19511,#19512,#19513,#19514,#19515,#19516,#19517,#19518,#19519,#19520,#19521,
#19522),.UNSPECIFIED.,.F.,.F.,(4,3,3,3,3,3,3,3,3,4),(0.,0.0913693045581935,
0.175304752632336,0.256829545365578,0.336180776983921,0.396785099350045,
0.504865678023515,0.611029081984597,0.715415587626544,0.795801737615703),
 .UNSPECIFIED.);
#502=B_SPLINE_CURVE_WITH_KNOTS('',3,(#19525,#19526,#19527,#19528,#19529,
#19530,#19531,#19532,#19533,#19534,#19535,#19536,#19537,#19538,#19539,#19540,
#19541,#19542,#19543,#19544,#19545,#19546,#19547,#19548,#19549,#19550,#19551,
#19552),.UNSPECIFIED.,.F.,.F.,(4,3,3,3,3,3,3,3,3,4),(0.,0.0913663024514722,
0.175300588104174,0.256824795817819,0.336175816276576,0.396785099350014,
0.504865277207551,0.611028582106192,0.71541572388289,0.795801737615583),
 .UNSPECIFIED.);
#503=B_SPLINE_CURVE_WITH_KNOTS('',3,(#19555,#19556,#19557,#19558,#19559,
#19560,#19561,#19562,#19563,#19564,#19565,#19566,#19567,#19568,#19569,#19570,
#19571,#19572,#19573,#19574,#19575,#19576,#19577,#19578,#19579,#19580,#19581,
#19582),.UNSPECIFIED.,.F.,.F.,(4,3,3,3,3,3,3,3,3,4),(0.,0.0913008476389673,
0.175225195872217,0.256743850113661,0.3360918680631,0.396785099350015,0.504848477488003,
0.610985103772403,0.715329935719092,0.795801737615593),.UNSPECIFIED.);
#504=B_SPLINE_CURVE_WITH_KNOTS('',3,(#19585,#19586,#19587,#19588,#19589,
#19590,#19591,#19592,#19593,#19594,#19595,#19596,#19597,#19598,#19599,#19600,
#19601,#19602,#19603,#19604,#19605,#19606,#19607,#19608,#19609,#19610,#19611,
#19612),.UNSPECIFIED.,.F.,.F.,(4,3,3,3,3,3,3,3,3,4),(0.,0.0913055244674033,
0.175231740458983,0.256751333954684,0.336099680903084,0.396785099350008,
0.504849076375157,0.610985832252606,0.715329675492173,0.795801737615577),
 .UNSPECIFIED.);
#505=B_SPLINE_CURVE_WITH_KNOTS('',3,(#19615,#19616,#19617,#19618,#19619,
#19620,#19621,#19622,#19623,#19624,#19625,#19626,#19627,#19628,#19629,#19630,
#19631,#19632,#19633,#19634,#19635,#19636,#19637,#19638,#19639,#19640,#19641,
#19642),.UNSPECIFIED.,.F.,.F.,(4,3,3,3,3,3,3,3,3,4),(0.,0.0913671480397717,
0.175301760935616,0.256826133349839,0.33617721329114,0.396785099349993,
0.504865390200107,0.611028723084967,0.715415685666501,0.795801737615502),
 .UNSPECIFIED.);
#506=B_SPLINE_CURVE_WITH_KNOTS('',3,(#19645,#19646,#19647,#19648,#19649,
#19650,#19651,#19652,#19653,#19654,#19655,#19656,#19657,#19658,#19659,#19660,
#19661,#19662,#19663,#19664,#19665,#19666,#19667,#19668,#19669,#19670,#19671,
#19672),.UNSPECIFIED.,.F.,.F.,(4,3,3,3,3,3,3,3,3,4),(0.,0.0913663024513228,
0.175300588104033,0.256824795817617,0.336175816276443,0.396785099350013,
0.504865277207549,0.61102858210682,0.715415723883384,0.795801737615587),
 .UNSPECIFIED.);
#507=B_SPLINE_CURVE_WITH_KNOTS('',3,(#19675,#19676,#19677,#19678,#19679,
#19680,#19681,#19682,#19683,#19684,#19685,#19686,#19687,#19688,#19689,#19690,
#19691,#19692,#19693,#19694,#19695,#19696,#19697,#19698,#19699,#19700,#19701,
#19702),.UNSPECIFIED.,.F.,.F.,(4,3,3,3,3,3,3,3,3,4),(0.,0.0913008476389372,
0.175225195872126,0.256743850113633,0.336091868062983,0.396785099350007,
0.504848477488055,0.610985103772565,0.715329935719059,0.795801737615582),
 .UNSPECIFIED.);
#508=B_SPLINE_CURVE_WITH_KNOTS('',3,(#19705,#19706,#19707,#19708,#19709,
#19710,#19711,#19712,#19713,#19714,#19715,#19716,#19717,#19718,#19719,#19720,
#19721,#19722,#19723,#19724,#19725,#19726,#19727,#19728,#19729,#19730,#19731,
#19732),.UNSPECIFIED.,.F.,.F.,(4,3,3,3,3,3,3,3,3,4),(0.,0.0913055244673888,
0.175231740458997,0.256751333954802,0.336099680903054,0.396785099350015,
0.504849076375127,0.610985832252708,0.715329675492648,0.795801737615576),
 .UNSPECIFIED.);
#509=B_SPLINE_CURVE_WITH_KNOTS('',3,(#19735,#19736,#19737,#19738,#19739,
#19740,#19741,#19742,#19743,#19744,#19745,#19746,#19747,#19748,#19749,#19750,
#19751,#19752,#19753,#19754,#19755,#19756,#19757,#19758,#19759,#19760,#19761,
#19762),.UNSPECIFIED.,.F.,.F.,(4,3,3,3,3,3,3,3,3,4),(0.,0.0913671480401054,
0.175301760935917,0.256826133350214,0.336177213291394,0.396785099349986,
0.504865390200262,0.611028723085204,0.715415685667019,0.795801737615469),
 .UNSPECIFIED.);
#510=B_SPLINE_CURVE_WITH_KNOTS('',3,(#19765,#19766,#19767,#19768,#19769,
#19770,#19771,#19772,#19773,#19774,#19775,#19776,#19777,#19778,#19779,#19780,
#19781,#19782,#19783,#19784,#19785,#19786,#19787,#19788,#19789,#19790,#19791,
#19792),.UNSPECIFIED.,.F.,.F.,(4,3,3,3,3,3,3,3,3,4),(0.,0.0913693045578756,
0.175304752632037,0.256829545365211,0.336180776983551,0.396785099350051,
0.504865678023637,0.611029081985028,0.715415587627274,0.79580173761574),
 .UNSPECIFIED.);
#511=B_SPLINE_CURVE_WITH_KNOTS('',3,(#19795,#19796,#19797,#19798,#19799,
#19800,#19801,#19802,#19803,#19804,#19805,#19806,#19807,#19808,#19809,#19810,
#19811,#19812,#19813,#19814,#19815,#19816,#19817,#19818,#19819,#19820,#19821,
#19822),.UNSPECIFIED.,.F.,.F.,(4,3,3,3,3,3,3,3,3,4),(0.,0.0913663024515618,
0.175300588104283,0.256824795817736,0.336175816276531,0.396785099350011,
0.504865277207547,0.611028582106704,0.715415723883272,0.795801737615553),
 .UNSPECIFIED.);
#512=B_SPLINE_CURVE_WITH_KNOTS('',3,(#19825,#19826,#19827,#19828,#19829,
#19830,#19831,#19832,#19833,#19834,#19835,#19836,#19837,#19838,#19839,#19840,
#19841,#19842,#19843,#19844,#19845,#19846,#19847,#19848,#19849,#19850,#19851,
#19852),.UNSPECIFIED.,.F.,.F.,(4,3,3,3,3,3,3,3,3,4),(0.,0.0913008476390098,
0.175225195872273,0.256743850113871,0.3360918680633,0.396785099350018,0.5048484774884,
0.610985103772909,0.715329935719289,0.795801737615643),.UNSPECIFIED.);
#513=B_SPLINE_CURVE_WITH_KNOTS('',3,(#19855,#19856,#19857,#19858,#19859,
#19860,#19861,#19862,#19863,#19864,#19865,#19866,#19867,#19868,#19869,#19870,
#19871,#19872,#19873,#19874,#19875,#19876,#19877,#19878,#19879,#19880,#19881,
#19882),.UNSPECIFIED.,.F.,.F.,(4,3,3,3,3,3,3,3,3,4),(0.,0.0913055244672643,
0.175231740458797,0.256751333954625,0.336099680903062,0.396785099349991,
0.504849076374745,0.610985832251881,0.715329675491931,0.795801737615494),
 .UNSPECIFIED.);
#514=B_SPLINE_CURVE_WITH_KNOTS('',3,(#19885,#19886,#19887,#19888,#19889,
#19890,#19891,#19892,#19893,#19894,#19895,#19896,#19897,#19898,#19899,#19900,
#19901,#19902,#19903,#19904,#19905,#19906,#19907,#19908,#19909,#19910,#19911,
#19912),.UNSPECIFIED.,.F.,.F.,(4,3,3,3,3,3,3,3,3,4),(0.,0.0913671480398292,
0.175301760935665,0.256826133349879,0.336177213291251,0.396785099350001,
0.504865390199928,0.611028723084993,0.715415685666863,0.795801737615546),
 .UNSPECIFIED.);
#515=B_SPLINE_CURVE_WITH_KNOTS('',3,(#19915,#19916,#19917,#19918,#19919,
#19920,#19921,#19922,#19923,#19924,#19925,#19926,#19927,#19928,#19929,#19930,
#19931,#19932,#19933,#19934,#19935,#19936,#19937,#19938,#19939,#19940,#19941,
#19942),.UNSPECIFIED.,.F.,.F.,(4,3,3,3,3,3,3,3,3,4),(0.,0.0913693045582462,
0.175304752632388,0.256829545365668,0.336180776983957,0.396785099350025,
0.50486567802321,0.6110290819841,0.715415587626411,0.795801737615617),
 .UNSPECIFIED.);
#516=B_SPLINE_CURVE_WITH_KNOTS('',3,(#19945,#19946,#19947,#19948,#19949,
#19950,#19951,#19952,#19953,#19954,#19955,#19956,#19957,#19958,#19959,#19960,
#19961,#19962,#19963,#19964,#19965,#19966,#19967,#19968,#19969,#19970,#19971,
#19972),.UNSPECIFIED.,.F.,.F.,(4,3,3,3,3,3,3,3,3,4),(0.,0.0913663024513698,
0.175300588104129,0.256824795817702,0.336175816276519,0.396785099350012,
0.504865277207553,0.611028582106785,0.71541572388335,0.795801737615573),
 .UNSPECIFIED.);
#629=SHAPE_REPRESENTATION_RELATIONSHIP('SRR','None',#23302,#639);
#639=ADVANCED_BREP_SHAPE_REPRESENTATION('',(#659),#23246);
#649=STYLED_ITEM('',(#23455),#659);
#659=MANIFOLD_SOLID_BREP('Body1',#7027);
#708=CONICAL_SURFACE('',#7413,2.175,0.785398163397448);
#709=CONICAL_SURFACE('',#7416,2.175,0.785398163397448);
#710=CONICAL_SURFACE('',#7419,6.275,0.785398163397448);
#711=CONICAL_SURFACE('',#7447,6.275,0.785398163397451);
#712=CONICAL_SURFACE('',#7451,9.75,0.785398163397451);
#713=CONICAL_SURFACE('',#7456,14.5,0.817645045832702);
#714=CONICAL_SURFACE('',#7458,14.5,0.817645045832702);
#715=CONICAL_SURFACE('',#7460,14.5,0.817645045832702);
#716=CONICAL_SURFACE('',#7462,14.5,0.817645045832702);
#717=CONICAL_SURFACE('',#7464,14.5,0.817645045832702);
#718=CONICAL_SURFACE('',#7466,14.5,0.817645045832702);
#719=CONICAL_SURFACE('',#7468,14.5,0.817645045832702);
#720=CONICAL_SURFACE('',#7470,14.5,0.817645045832702);
#721=CONICAL_SURFACE('',#7472,14.5,0.817645045832702);
#722=CONICAL_SURFACE('',#7474,14.5,0.817645045832702);
#723=CONICAL_SURFACE('',#7476,14.5,0.817645045832702);
#724=CONICAL_SURFACE('',#7478,14.5,0.817645045832702);
#725=CONICAL_SURFACE('',#7480,14.5,0.817645045832702);
#726=CONICAL_SURFACE('',#7482,14.5,0.817645045832702);
#727=CONICAL_SURFACE('',#7484,14.5,0.817645045832702);
#728=CONICAL_SURFACE('',#7486,14.5,0.817645045832702);
#729=CONICAL_SURFACE('',#7488,14.5,0.817645045832702);
#730=CONICAL_SURFACE('',#7490,14.5,0.817645045832702);
#731=CONICAL_SURFACE('',#7492,14.5,0.817645045832702);
#732=CONICAL_SURFACE('',#7494,14.5,0.817645045832702);
#733=CONICAL_SURFACE('',#7499,14.5,0.817645045832702);
#734=CONICAL_SURFACE('',#7503,12.1473403730037,0.739193465255218);
#803=FACE_BOUND('',#1569,.T.);
#804=FACE_BOUND('',#1571,.T.);
#805=FACE_BOUND('',#1574,.T.);
#806=FACE_BOUND('',#1577,.T.);
#807=FACE_BOUND('',#1662,.T.);
#909=PLANE('',#7426);
#910=PLANE('',#7449);
#911=PLANE('',#7501);
#912=PLANE('',#7524);
#913=PLANE('',#7525);
#914=PLANE('',#7526);
#915=PLANE('',#7527);
#916=PLANE('',#7528);
#917=PLANE('',#7529);
#918=PLANE('',#7530);
#919=PLANE('',#7531);
#920=PLANE('',#7532);
#921=PLANE('',#7533);
#922=PLANE('',#7534);
#923=PLANE('',#7535);
#924=PLANE('',#7536);
#925=PLANE('',#7537);
#926=PLANE('',#7538);
#927=PLANE('',#7539);
#928=PLANE('',#7540);
#929=PLANE('',#7541);
#930=PLANE('',#7542);
#931=PLANE('',#7543);
#1145=FACE_OUTER_BOUND('',#1563,.T.);
#1146=FACE_OUTER_BOUND('',#1564,.T.);
#1147=FACE_OUTER_BOUND('',#1565,.T.);
#1148=FACE_OUTER_BOUND('',#1566,.T.);
#1149=FACE_OUTER_BOUND('',#1567,.T.);
#1150=FACE_OUTER_BOUND('',#1568,.T.);
#1151=FACE_OUTER_BOUND('',#1570,.T.);
#1152=FACE_OUTER_BOUND('',#1572,.T.);
#1153=FACE_OUTER_BOUND('',#1573,.T.);
#1154=FACE_OUTER_BOUND('',#1575,.T.);
#1155=FACE_OUTER_BOUND('',#1576,.T.);
#1156=FACE_OUTER_BOUND('',#1578,.T.);
#1157=FACE_OUTER_BOUND('',#1579,.T.);
#1158=FACE_OUTER_BOUND('',#1580,.T.);
#1159=FACE_OUTER_BOUND('',#1581,.T.);
#1160=FACE_OUTER_BOUND('',#1582,.T.);
#1161=FACE_OUTER_BOUND('',#1583,.T.);
#1162=FACE_OUTER_BOUND('',#1584,.T.);
#1163=FACE_OUTER_BOUND('',#1585,.T.);
#1164=FACE_OUTER_BOUND('',#1586,.T.);
#1165=FACE_OUTER_BOUND('',#1587,.T.);
#1166=FACE_OUTER_BOUND('',#1588,.T.);
#1167=FACE_OUTER_BOUND('',#1589,.T.);
#1168=FACE_OUTER_BOUND('',#1590,.T.);
#1169=FACE_OUTER_BOUND('',#1591,.T.);
#1170=FACE_OUTER_BOUND('',#1592,.T.);
#1171=FACE_OUTER_BOUND('',#1593,.T.);
#1172=FACE_OUTER_BOUND('',#1594,.T.);
#1173=FACE_OUTER_BOUND('',#1595,.T.);
#1174=FACE_OUTER_BOUND('',#1596,.T.);
#1175=FACE_OUTER_BOUND('',#1597,.T.);
#1176=FACE_OUTER_BOUND('',#1598,.T.);
#1177=FACE_OUTER_BOUND('',#1599,.T.);
#1178=FACE_OUTER_BOUND('',#1600,.T.);
#1179=FACE_OUTER_BOUND('',#1601,.T.);
#1180=FACE_OUTER_BOUND('',#1602,.T.);
#1181=FACE_OUTER_BOUND('',#1603,.T.);
#1182=FACE_OUTER_BOUND('',#1604,.T.);
#1183=FACE_OUTER_BOUND('',#1605,.T.);
#1184=FACE_OUTER_BOUND('',#1606,.T.);
#1185=FACE_OUTER_BOUND('',#1607,.T.);
#1186=FACE_OUTER_BOUND('',#1608,.T.);
#1187=FACE_OUTER_BOUND('',#1609,.T.);
#1188=FACE_OUTER_BOUND('',#1610,.T.);
#1189=FACE_OUTER_BOUND('',#1611,.T.);
#1190=FACE_OUTER_BOUND('',#1612,.T.);
#1191=FACE_OUTER_BOUND('',#1613,.T.);
#1192=FACE_OUTER_BOUND('',#1614,.T.);
#1193=FACE_OUTER_BOUND('',#1615,.T.);
#1194=FACE_OUTER_BOUND('',#1616,.T.);
#1195=FACE_OUTER_BOUND('',#1617,.T.);
#1196=FACE_OUTER_BOUND('',#1618,.T.);
#1197=FACE_OUTER_BOUND('',#1619,.T.);
#1198=FACE_OUTER_BOUND('',#1620,.T.);
#1199=FACE_OUTER_BOUND('',#1621,.T.);
#1200=FACE_OUTER_BOUND('',#1622,.T.);
#1201=FACE_OUTER_BOUND('',#1623,.T.);
#1202=FACE_OUTER_BOUND('',#1624,.T.);
#1203=FACE_OUTER_BOUND('',#1625,.T.);
#1204=FACE_OUTER_BOUND('',#1626,.T.);
#1205=FACE_OUTER_BOUND('',#1627,.T.);
#1206=FACE_OUTER_BOUND('',#1628,.T.);
#1207=FACE_OUTER_BOUND('',#1629,.T.);
#1208=FACE_OUTER_BOUND('',#1630,.T.);
#1209=FACE_OUTER_BOUND('',#1631,.T.);
#1210=FACE_OUTER_BOUND('',#1632,.T.);
#1211=FACE_OUTER_BOUND('',#1633,.T.);
#1212=FACE_OUTER_BOUND('',#1634,.T.);
#1213=FACE_OUTER_BOUND('',#1635,.T.);
#1214=FACE_OUTER_BOUND('',#1636,.T.);
#1215=FACE_OUTER_BOUND('',#1637,.T.);
#1216=FACE_OUTER_BOUND('',#1638,.T.);
#1217=FACE_OUTER_BOUND('',#1639,.T.);
#1218=FACE_OUTER_BOUND('',#1640,.T.);
#1219=FACE_OUTER_BOUND('',#1641,.T.);
#1220=FACE_OUTER_BOUND('',#1642,.T.);
#1221=FACE_OUTER_BOUND('',#1643,.T.);
#1222=FACE_OUTER_BOUND('',#1644,.T.);
#1223=FACE_OUTER_BOUND('',#1645,.T.);
#1224=FACE_OUTER_BOUND('',#1646,.T.);
#1225=FACE_OUTER_BOUND('',#1647,.T.);
#1226=FACE_OUTER_BOUND('',#1648,.T.);
#1227=FACE_OUTER_BOUND('',#1649,.T.);
#1228=FACE_OUTER_BOUND('',#1650,.T.);
#1229=FACE_OUTER_BOUND('',#1651,.T.);
#1230=FACE_OUTER_BOUND('',#1652,.T.);
#1231=FACE_OUTER_BOUND('',#1653,.T.);
#1232=FACE_OUTER_BOUND('',#1654,.T.);
#1233=FACE_OUTER_BOUND('',#1655,.T.);
#1234=FACE_OUTER_BOUND('',#1656,.T.);
#1235=FACE_OUTER_BOUND('',#1657,.T.);
#1236=FACE_OUTER_BOUND('',#1658,.T.);
#1237=FACE_OUTER_BOUND('',#1659,.T.);
#1238=FACE_OUTER_BOUND('',#1660,.T.);
#1239=FACE_OUTER_BOUND('',#1661,.T.);
#1563=EDGE_LOOP('',(#5313,#5314,#5315,#5316,#5317,#5318));
#1564=EDGE_LOOP('',(#5319,#5320,#5321,#5322,#5323,#5324));
#1565=EDGE_LOOP('',(#5325,#5326,#5327,#5328,#5329));
#1566=EDGE_LOOP('',(#5330,#5331,#5332,#5333,#5334));
#1567=EDGE_LOOP('',(#5335,#5336,#5337,#5338,#5339));
#1568=EDGE_LOOP('',(#5340,#5341,#5342,#5343,#5344,#5345,#5346,#5347,#5348,
#5349,#5350));
#1569=EDGE_LOOP('',(#5351,#5352));
#1570=EDGE_LOOP('',(#5353,#5354,#5355,#5356,#5357,#5358,#5359,#5360,#5361,
#5362,#5363,#5364,#5365,#5366,#5367,#5368,#5369,#5370,#5371,#5372,#5373,
#5374,#5375,#5376,#5377,#5378,#5379,#5380,#5381,#5382,#5383,#5384,#5385,
#5386,#5387,#5388,#5389,#5390,#5391,#5392,#5393,#5394,#5395,#5396,#5397,
#5398,#5399,#5400,#5401,#5402,#5403,#5404,#5405,#5406,#5407,#5408,#5409,
#5410,#5411,#5412));
#1571=EDGE_LOOP('',(#5413));
#1572=EDGE_LOOP('',(#5414,#5415,#5416,#5417,#5418));
#1573=EDGE_LOOP('',(#5419));
#1574=EDGE_LOOP('',(#5420));
#1575=EDGE_LOOP('',(#5421,#5422,#5423,#5424,#5425));
#1576=EDGE_LOOP('',(#5426,#5427,#5428,#5429,#5430,#5431,#5432,#5433,#5434,
#5435));
#1577=EDGE_LOOP('',(#5436,#5437));
#1578=EDGE_LOOP('',(#5438,#5439,#5440));
#1579=EDGE_LOOP('',(#5441,#5442,#5443));
#1580=EDGE_LOOP('',(#5444,#5445,#5446));
#1581=EDGE_LOOP('',(#5447,#5448,#5449));
#1582=EDGE_LOOP('',(#5450,#5451,#5452));
#1583=EDGE_LOOP('',(#5453,#5454,#5455));
#1584=EDGE_LOOP('',(#5456,#5457,#5458));
#1585=EDGE_LOOP('',(#5459,#5460,#5461));
#1586=EDGE_LOOP('',(#5462,#5463,#5464));
#1587=EDGE_LOOP('',(#5465,#5466,#5467));
#1588=EDGE_LOOP('',(#5468,#5469,#5470));
#1589=EDGE_LOOP('',(#5471,#5472,#5473));
#1590=EDGE_LOOP('',(#5474,#5475,#5476));
#1591=EDGE_LOOP('',(#5477,#5478,#5479));
#1592=EDGE_LOOP('',(#5480,#5481,#5482));
#1593=EDGE_LOOP('',(#5483,#5484,#5485));
#1594=EDGE_LOOP('',(#5486,#5487,#5488));
#1595=EDGE_LOOP('',(#5489,#5490,#5491));
#1596=EDGE_LOOP('',(#5492,#5493,#5494));
#1597=EDGE_LOOP('',(#5495,#5496,#5497,#5498));
#1598=EDGE_LOOP('',(#5499,#5500,#5501,#5502));
#1599=EDGE_LOOP('',(#5503,#5504,#5505));
#1600=EDGE_LOOP('',(#5506,#5507,#5508,#5509,#5510));
#1601=EDGE_LOOP('',(#5511,#5512,#5513,#5514,#5515));
#1602=EDGE_LOOP('',(#5516,#5517,#5518,#5519,#5520));
#1603=EDGE_LOOP('',(#5521,#5522,#5523,#5524,#5525));
#1604=EDGE_LOOP('',(#5526,#5527,#5528,#5529,#5530));
#1605=EDGE_LOOP('',(#5531,#5532,#5533,#5534,#5535));
#1606=EDGE_LOOP('',(#5536,#5537,#5538,#5539,#5540));
#1607=EDGE_LOOP('',(#5541,#5542,#5543,#5544,#5545));
#1608=EDGE_LOOP('',(#5546,#5547,#5548,#5549,#5550));
#1609=EDGE_LOOP('',(#5551,#5552,#5553,#5554,#5555));
#1610=EDGE_LOOP('',(#5556,#5557,#5558,#5559,#5560));
#1611=EDGE_LOOP('',(#5561,#5562,#5563,#5564,#5565));
#1612=EDGE_LOOP('',(#5566,#5567,#5568,#5569,#5570));
#1613=EDGE_LOOP('',(#5571,#5572,#5573,#5574,#5575));
#1614=EDGE_LOOP('',(#5576,#5577,#5578,#5579,#5580));
#1615=EDGE_LOOP('',(#5581,#5582,#5583,#5584,#5585));
#1616=EDGE_LOOP('',(#5586,#5587,#5588,#5589,#5590));
#1617=EDGE_LOOP('',(#5591,#5592,#5593,#5594,#5595));
#1618=EDGE_LOOP('',(#5596,#5597,#5598,#5599,#5600));
#1619=EDGE_LOOP('',(#5601,#5602,#5603,#5604,#5605));
#1620=EDGE_LOOP('',(#5606,#5607,#5608,#5609,#5610));
#1621=EDGE_LOOP('',(#5611,#5612,#5613,#5614));
#1622=EDGE_LOOP('',(#5615,#5616,#5617,#5618,#5619,#5620,#5621,#5622,#5623,
#5624,#5625,#5626,#5627,#5628,#5629,#5630,#5631,#5632,#5633,#5634,#5635,
#5636,#5637,#5638,#5639,#5640,#5641,#5642,#5643,#5644,#5645,#5646,#5647,
#5648,#5649,#5650,#5651,#5652,#5653,#5654,#5655,#5656,#5657,#5658,#5659,
#5660,#5661,#5662,#5663,#5664,#5665,#5666,#5667,#5668,#5669,#5670,#5671,
#5672,#5673,#5674,#5675,#5676,#5677,#5678,#5679,#5680,#5681,#5682,#5683,
#5684,#5685,#5686,#5687,#5688,#5689,#5690,#5691,#5692,#5693,#5694,#5695,
#5696,#5697,#5698));
#1623=EDGE_LOOP('',(#5699,#5700,#5701,#5702,#5703));
#1624=EDGE_LOOP('',(#5704,#5705,#5706,#5707));
#1625=EDGE_LOOP('',(#5708,#5709,#5710,#5711,#5712));
#1626=EDGE_LOOP('',(#5713,#5714,#5715,#5716));
#1627=EDGE_LOOP('',(#5717,#5718,#5719,#5720,#5721));
#1628=EDGE_LOOP('',(#5722,#5723,#5724,#5725));
#1629=EDGE_LOOP('',(#5726,#5727,#5728,#5729,#5730));
#1630=EDGE_LOOP('',(#5731,#5732,#5733,#5734));
#1631=EDGE_LOOP('',(#5735,#5736,#5737,#5738,#5739));
#1632=EDGE_LOOP('',(#5740,#5741,#5742,#5743));
#1633=EDGE_LOOP('',(#5744,#5745,#5746,#5747,#5748));
#1634=EDGE_LOOP('',(#5749,#5750,#5751,#5752));
#1635=EDGE_LOOP('',(#5753,#5754,#5755,#5756,#5757));
#1636=EDGE_LOOP('',(#5758,#5759,#5760,#5761));
#1637=EDGE_LOOP('',(#5762,#5763,#5764,#5765,#5766));
#1638=EDGE_LOOP('',(#5767,#5768,#5769,#5770));
#1639=EDGE_LOOP('',(#5771,#5772,#5773,#5774,#5775));
#1640=EDGE_LOOP('',(#5776,#5777,#5778,#5779,#5780));
#1641=EDGE_LOOP('',(#5781,#5782,#5783,#5784,#5785));
#1642=EDGE_LOOP('',(#5786,#5787,#5788,#5789));
#1643=EDGE_LOOP('',(#5790,#5791,#5792,#5793,#5794));
#1644=EDGE_LOOP('',(#5795,#5796,#5797,#5798));
#1645=EDGE_LOOP('',(#5799,#5800,#5801,#5802,#5803));
#1646=EDGE_LOOP('',(#5804,#5805,#5806,#5807));
#1647=EDGE_LOOP('',(#5808,#5809,#5810,#5811,#5812));
#1648=EDGE_LOOP('',(#5813,#5814,#5815,#5816));
#1649=EDGE_LOOP('',(#5817,#5818,#5819,#5820,#5821));
#1650=EDGE_LOOP('',(#5822,#5823,#5824,#5825));
#1651=EDGE_LOOP('',(#5826,#5827,#5828,#5829,#5830));
#1652=EDGE_LOOP('',(#5831,#5832,#5833,#5834));
#1653=EDGE_LOOP('',(#5835,#5836,#5837,#5838,#5839));
#1654=EDGE_LOOP('',(#5840,#5841,#5842,#5843));
#1655=EDGE_LOOP('',(#5844,#5845,#5846,#5847,#5848));
#1656=EDGE_LOOP('',(#5849,#5850,#5851,#5852));
#1657=EDGE_LOOP('',(#5853,#5854,#5855,#5856,#5857));
#1658=EDGE_LOOP('',(#5858,#5859,#5860,#5861));
#1659=EDGE_LOOP('',(#5862,#5863,#5864,#5865,#5866));
#1660=EDGE_LOOP('',(#5867,#5868,#5869,#5870));
#1661=EDGE_LOOP('',(#5871));
#1662=EDGE_LOOP('',(#5872));
#1959=LINE('',#15887,#2218);
#1960=LINE('',#15891,#2219);
#1961=LINE('',#15954,#2220);
#1962=LINE('',#15977,#2221);
#1963=LINE('',#16019,#2222);
#1964=LINE('',#16028,#2223);
#1965=LINE('',#16029,#2224);
#1966=LINE('',#17513,#2225);
#1967=LINE('',#17520,#2226);
#1968=LINE('',#17525,#2227);
#1969=LINE('',#17527,#2228);
#1970=LINE('',#18084,#2229);
#1971=LINE('',#18088,#2230);
#1972=LINE('',#18143,#2231);
#1973=LINE('',#18203,#2232);
#1974=LINE('',#18263,#2233);
#1975=LINE('',#18323,#2234);
#1976=LINE('',#18383,#2235);
#1977=LINE('',#18443,#2236);
#1978=LINE('',#18503,#2237);
#1979=LINE('',#18563,#2238);
#1980=LINE('',#18623,#2239);
#1981=LINE('',#18683,#2240);
#1982=LINE('',#18743,#2241);
#1983=LINE('',#18803,#2242);
#1984=LINE('',#18863,#2243);
#1985=LINE('',#18923,#2244);
#1986=LINE('',#18983,#2245);
#1987=LINE('',#19043,#2246);
#1988=LINE('',#19103,#2247);
#1989=LINE('',#19163,#2248);
#1990=LINE('',#19223,#2249);
#1991=LINE('',#19283,#2250);
#1992=LINE('',#19402,#2251);
#2218=VECTOR('',#8485,2.175);
#2219=VECTOR('',#8490,2.05);
#2220=VECTOR('',#8493,2.175);
#2221=VECTOR('',#8498,2.05);
#2222=VECTOR('',#8503,6.275);
#2223=VECTOR('',#8514,6.025);
#2224=VECTOR('',#8515,6.025);
#2225=VECTOR('',#8560,6.275);
#2226=VECTOR('',#8569,9.75);
#2227=VECTOR('',#8576,10.);
#2228=VECTOR('',#8577,10.);
#2229=VECTOR('',#8660,14.5);
#2230=VECTOR('',#8665,10.5);
#2231=VECTOR('',#8672,8.74592262443523);
#2232=VECTOR('',#8673,8.74592262443523);
#2233=VECTOR('',#8674,8.74592262443523);
#2234=VECTOR('',#8675,8.74592262443523);
#2235=VECTOR('',#8676,8.74592262443523);
#2236=VECTOR('',#8677,8.74592262443523);
#2237=VECTOR('',#8678,8.74592262443523);
#2238=VECTOR('',#8679,8.74592262443523);
#2239=VECTOR('',#8680,8.74592262443523);
#2240=VECTOR('',#8681,8.74592262443523);
#2241=VECTOR('',#8682,8.74592262443523);
#2242=VECTOR('',#8683,8.74592262443523);
#2243=VECTOR('',#8684,8.74592262443523);
#2244=VECTOR('',#8685,8.74592262443523);
#2245=VECTOR('',#8686,8.74592262443523);
#2246=VECTOR('',#8687,8.74592262443523);
#2247=VECTOR('',#8688,8.74592262443523);
#2248=VECTOR('',#8689,8.74592262443523);
#2249=VECTOR('',#8690,8.74592262443523);
#2250=VECTOR('',#8691,8.74592262443523);
#2251=VECTOR('',#8698,12.1473403730037);
#2496=CIRCLE('',#7414,2.05);
#2497=CIRCLE('',#7417,2.05);
#2498=CIRCLE('',#7420,6.525);
#2499=CIRCLE('',#7421,6.025);
#2500=CIRCLE('',#7422,6.025);
#2501=CIRCLE('',#7424,6.025);
#2502=CIRCLE('',#7425,6.025);
#2503=CIRCLE('',#7427,9.16192731696939);
#2504=CIRCLE('',#7428,9.16192731696939);
#2505=CIRCLE('',#7429,9.16192731696939);
#2506=CIRCLE('',#7430,9.16192731696939);
#2507=CIRCLE('',#7431,9.16192731696939);
#2508=CIRCLE('',#7432,9.16192731696939);
#2509=CIRCLE('',#7433,9.16192731696939);
#2510=CIRCLE('',#7434,9.16192731696939);
#2511=CIRCLE('',#7435,9.16192731696939);
#2512=CIRCLE('',#7436,9.16192731696939);
#2513=CIRCLE('',#7437,9.16192731696939);
#2514=CIRCLE('',#7438,9.16192731696939);
#2515=CIRCLE('',#7439,9.16192731696939);
#2516=CIRCLE('',#7440,9.16192731696939);
#2517=CIRCLE('',#7441,9.16192731696939);
#2518=CIRCLE('',#7442,9.16192731696939);
#2519=CIRCLE('',#7443,9.16192731696939);
#2520=CIRCLE('',#7444,9.16192731696939);
#2521=CIRCLE('',#7445,9.16192731696939);
#2522=CIRCLE('',#7446,9.16192731696939);
#2523=CIRCLE('',#7448,6.525);
#2524=CIRCLE('',#7450,9.5);
#2525=CIRCLE('',#7452,10.);
#2526=CIRCLE('',#7453,10.);
#2527=CIRCLE('',#7455,10.);
#2528=CIRCLE('',#7457,14.4466666666667);
#2529=CIRCLE('',#7459,14.4466666666667);
#2530=CIRCLE('',#7461,14.4466666666667);
#2531=CIRCLE('',#7463,14.4466666666667);
#2532=CIRCLE('',#7465,14.4466666666667);
#2533=CIRCLE('',#7467,14.4466666666667);
#2534=CIRCLE('',#7469,14.4466666666667);
#2535=CIRCLE('',#7471,14.4466666666667);
#2536=CIRCLE('',#7473,14.4466666666667);
#2537=CIRCLE('',#7475,14.4466666666667);
#2538=CIRCLE('',#7477,14.4466666666667);
#2539=CIRCLE('',#7479,14.4466666666667);
#2540=CIRCLE('',#7481,14.4466666666667);
#2541=CIRCLE('',#7483,14.4466666666667);
#2542=CIRCLE('',#7485,14.4466666666667);
#2543=CIRCLE('',#7487,14.4466666666667);
#2544=CIRCLE('',#7489,14.4466666666667);
#2545=CIRCLE('',#7491,14.4466666666667);
#2546=CIRCLE('',#7493,14.4466666666667);
#2547=CIRCLE('',#7495,14.4233723052509);
#2548=CIRCLE('',#7496,10.5);
#2549=CIRCLE('',#7498,10.5);
#2550=CIRCLE('',#7500,14.4466666666667);
#2551=CIRCLE('',#7502,14.4034641071566);
#2552=CIRCLE('',#7504,14.4034641071566);
#2553=CIRCLE('',#7505,14.4034641071566);
#2554=CIRCLE('',#7506,14.4034641071566);
#2555=CIRCLE('',#7507,14.4034641071566);
#2556=CIRCLE('',#7508,14.4034641071566);
#2557=CIRCLE('',#7509,14.4034641071566);
#2558=CIRCLE('',#7510,14.4034641071566);
#2559=CIRCLE('',#7511,14.4034641071566);
#2560=CIRCLE('',#7512,14.4034641071566);
#2561=CIRCLE('',#7513,14.4034641071566);
#2562=CIRCLE('',#7514,14.4034641071566);
#2563=CIRCLE('',#7515,14.4034641071566);
#2564=CIRCLE('',#7516,14.4034641071566);
#2565=CIRCLE('',#7517,14.4034641071566);
#2566=CIRCLE('',#7518,14.4034641071566);
#2567=CIRCLE('',#7519,14.4034641071566);
#2568=CIRCLE('',#7520,14.4034641071566);
#2569=CIRCLE('',#7521,14.4034641071566);
#2570=CIRCLE('',#7522,14.4034641071566);
#2571=CIRCLE('',#7523,14.4034641071566);
#2978=VERTEX_POINT('',#15844);
#2979=VERTEX_POINT('',#15845);
#2980=VERTEX_POINT('',#15856);
#2981=VERTEX_POINT('',#15886);
#2982=VERTEX_POINT('',#15890);
#2983=VERTEX_POINT('',#15892);
#2984=VERTEX_POINT('',#15903);
#2985=VERTEX_POINT('',#15933);
#2986=VERTEX_POINT('',#15934);
#2987=VERTEX_POINT('',#15953);
#2988=VERTEX_POINT('',#15976);
#2989=VERTEX_POINT('',#15978);
#2990=VERTEX_POINT('',#16016);
#2991=VERTEX_POINT('',#16018);
#2992=VERTEX_POINT('',#16020);
#2993=VERTEX_POINT('',#16024);
#2994=VERTEX_POINT('',#16025);
#2995=VERTEX_POINT('',#16031);
#2996=VERTEX_POINT('',#16032);
#2997=VERTEX_POINT('',#16034);
#2998=VERTEX_POINT('',#16070);
#2999=VERTEX_POINT('',#16106);
#3000=VERTEX_POINT('',#16108);
#3001=VERTEX_POINT('',#16144);
#3002=VERTEX_POINT('',#16180);
#3003=VERTEX_POINT('',#16182);
#3004=VERTEX_POINT('',#16218);
#3005=VERTEX_POINT('',#16254);
#3006=VERTEX_POINT('',#16256);
#3007=VERTEX_POINT('',#16292);
#3008=VERTEX_POINT('',#16328);
#3009=VERTEX_POINT('',#16330);
#3010=VERTEX_POINT('',#16366);
#3011=VERTEX_POINT('',#16402);
#3012=VERTEX_POINT('',#16404);
#3013=VERTEX_POINT('',#16440);
#3014=VERTEX_POINT('',#16476);
#3015=VERTEX_POINT('',#16478);
#3016=VERTEX_POINT('',#16514);
#3017=VERTEX_POINT('',#16550);
#3018=VERTEX_POINT('',#16552);
#3019=VERTEX_POINT('',#16588);
#3020=VERTEX_POINT('',#16624);
#3021=VERTEX_POINT('',#16626);
#3022=VERTEX_POINT('',#16662);
#3023=VERTEX_POINT('',#16698);
#3024=VERTEX_POINT('',#16700);
#3025=VERTEX_POINT('',#16736);
#3026=VERTEX_POINT('',#16772);
#3027=VERTEX_POINT('',#16774);
#3028=VERTEX_POINT('',#16810);
#3029=VERTEX_POINT('',#16846);
#3030=VERTEX_POINT('',#16848);
#3031=VERTEX_POINT('',#16884);
#3032=VERTEX_POINT('',#16920);
#3033=VERTEX_POINT('',#16922);
#3034=VERTEX_POINT('',#16958);
#3035=VERTEX_POINT('',#16994);
#3036=VERTEX_POINT('',#16996);
#3037=VERTEX_POINT('',#17032);
#3038=VERTEX_POINT('',#17068);
#3039=VERTEX_POINT('',#17070);
#3040=VERTEX_POINT('',#17106);
#3041=VERTEX_POINT('',#17142);
#3042=VERTEX_POINT('',#17144);
#3043=VERTEX_POINT('',#17180);
#3044=VERTEX_POINT('',#17216);
#3045=VERTEX_POINT('',#17218);
#3046=VERTEX_POINT('',#17254);
#3047=VERTEX_POINT('',#17290);
#3048=VERTEX_POINT('',#17292);
#3049=VERTEX_POINT('',#17328);
#3050=VERTEX_POINT('',#17364);
#3051=VERTEX_POINT('',#17366);
#3052=VERTEX_POINT('',#17402);
#3053=VERTEX_POINT('',#17438);
#3054=VERTEX_POINT('',#17440);
#3055=VERTEX_POINT('',#17512);
#3056=VERTEX_POINT('',#17516);
#3057=VERTEX_POINT('',#17519);
#3058=VERTEX_POINT('',#17521);
#3059=VERTEX_POINT('',#17526);
#3060=VERTEX_POINT('',#17530);
#3061=VERTEX_POINT('',#17531);
#3062=VERTEX_POINT('',#17546);
#3063=VERTEX_POINT('',#17559);
#3064=VERTEX_POINT('',#17560);
#3065=VERTEX_POINT('',#17575);
#3066=VERTEX_POINT('',#17588);
#3067=VERTEX_POINT('',#17589);
#3068=VERTEX_POINT('',#17604);
#3069=VERTEX_POINT('',#17617);
#3070=VERTEX_POINT('',#17618);
#3071=VERTEX_POINT('',#17633);
#3072=VERTEX_POINT('',#17646);
#3073=VERTEX_POINT('',#17647);
#3074=VERTEX_POINT('',#17662);
#3075=VERTEX_POINT('',#17675);
#3076=VERTEX_POINT('',#17676);
#3077=VERTEX_POINT('',#17691);
#3078=VERTEX_POINT('',#17704);
#3079=VERTEX_POINT('',#17705);
#3080=VERTEX_POINT('',#17720);
#3081=VERTEX_POINT('',#17733);
#3082=VERTEX_POINT('',#17734);
#3083=VERTEX_POINT('',#17749);
#3084=VERTEX_POINT('',#17762);
#3085=VERTEX_POINT('',#17763);
#3086=VERTEX_POINT('',#17778);
#3087=VERTEX_POINT('',#17791);
#3088=VERTEX_POINT('',#17792);
#3089=VERTEX_POINT('',#17807);
#3090=VERTEX_POINT('',#17820);
#3091=VERTEX_POINT('',#17821);
#3092=VERTEX_POINT('',#17836);
#3093=VERTEX_POINT('',#17849);
#3094=VERTEX_POINT('',#17850);
#3095=VERTEX_POINT('',#17865);
#3096=VERTEX_POINT('',#17878);
#3097=VERTEX_POINT('',#17879);
#3098=VERTEX_POINT('',#17894);
#3099=VERTEX_POINT('',#17907);
#3100=VERTEX_POINT('',#17908);
#3101=VERTEX_POINT('',#17923);
#3102=VERTEX_POINT('',#17936);
#3103=VERTEX_POINT('',#17937);
#3104=VERTEX_POINT('',#17952);
#3105=VERTEX_POINT('',#17965);
#3106=VERTEX_POINT('',#17966);
#3107=VERTEX_POINT('',#17981);
#3108=VERTEX_POINT('',#17994);
#3109=VERTEX_POINT('',#17995);
#3110=VERTEX_POINT('',#18010);
#3111=VERTEX_POINT('',#18023);
#3112=VERTEX_POINT('',#18024);
#3113=VERTEX_POINT('',#18039);
#3114=VERTEX_POINT('',#18052);
#3115=VERTEX_POINT('',#18053);
#3116=VERTEX_POINT('',#18068);
#3117=VERTEX_POINT('',#18081);
#3118=VERTEX_POINT('',#18083);
#3119=VERTEX_POINT('',#18087);
#3120=VERTEX_POINT('',#18091);
#3121=VERTEX_POINT('',#18092);
#3122=VERTEX_POINT('',#18107);
#3123=VERTEX_POINT('',#18144);
#3124=VERTEX_POINT('',#18204);
#3125=VERTEX_POINT('',#18264);
#3126=VERTEX_POINT('',#18324);
#3127=VERTEX_POINT('',#18384);
#3128=VERTEX_POINT('',#18444);
#3129=VERTEX_POINT('',#18504);
#3130=VERTEX_POINT('',#18564);
#3131=VERTEX_POINT('',#18624);
#3132=VERTEX_POINT('',#18684);
#3133=VERTEX_POINT('',#18744);
#3134=VERTEX_POINT('',#18804);
#3135=VERTEX_POINT('',#18864);
#3136=VERTEX_POINT('',#18924);
#3137=VERTEX_POINT('',#18984);
#3138=VERTEX_POINT('',#19044);
#3139=VERTEX_POINT('',#19104);
#3140=VERTEX_POINT('',#19164);
#3141=VERTEX_POINT('',#19224);
#3142=VERTEX_POINT('',#19284);
#3143=VERTEX_POINT('',#19363);
#3144=VERTEX_POINT('',#19401);
#3145=VERTEX_POINT('',#19404);
#3146=VERTEX_POINT('',#19434);
#3147=VERTEX_POINT('',#19464);
#3148=VERTEX_POINT('',#19494);
#3149=VERTEX_POINT('',#19524);
#3150=VERTEX_POINT('',#19554);
#3151=VERTEX_POINT('',#19584);
#3152=VERTEX_POINT('',#19614);
#3153=VERTEX_POINT('',#19644);
#3154=VERTEX_POINT('',#19674);
#3155=VERTEX_POINT('',#19704);
#3156=VERTEX_POINT('',#19734);
#3157=VERTEX_POINT('',#19764);
#3158=VERTEX_POINT('',#19794);
#3159=VERTEX_POINT('',#19824);
#3160=VERTEX_POINT('',#19854);
#3161=VERTEX_POINT('',#19884);
#3162=VERTEX_POINT('',#19914);
#3163=VERTEX_POINT('',#19944);
#3832=EDGE_CURVE('',#2978,#2979,#427,.T.);
#3833=EDGE_CURVE('',#2980,#2978,#428,.T.);
#3834=EDGE_CURVE('',#2979,#2980,#429,.T.);
#3835=EDGE_CURVE('',#2979,#2981,#1959,.T.);
#3836=EDGE_CURVE('',#2981,#2981,#2496,.T.);
#3837=EDGE_CURVE('',#2981,#2982,#1960,.T.);
#3838=EDGE_CURVE('',#2983,#2982,#430,.T.);
#3839=EDGE_CURVE('',#2984,#2983,#431,.T.);
#3840=EDGE_CURVE('',#2982,#2984,#432,.T.);
#3841=EDGE_CURVE('',#2985,#2986,#433,.T.);
#3842=EDGE_CURVE('',#2985,#2987,#1961,.T.);
#3843=EDGE_CURVE('',#2987,#2987,#2497,.T.);
#3844=EDGE_CURVE('',#2986,#2985,#434,.T.);
#3845=EDGE_CURVE('',#2987,#2988,#1962,.T.);
#3846=EDGE_CURVE('',#2989,#2988,#435,.T.);
#3847=EDGE_CURVE('',#2988,#2989,#436,.T.);
#3848=EDGE_CURVE('',#2990,#2990,#2498,.T.);
#3849=EDGE_CURVE('',#2990,#2991,#1963,.T.);
#3850=EDGE_CURVE('',#2991,#2992,#2499,.T.);
#3851=EDGE_CURVE('',#2992,#2991,#2500,.T.);
#3852=EDGE_CURVE('',#2993,#2994,#2501,.T.);
#3853=EDGE_CURVE('',#2994,#2993,#2502,.T.);
#3854=EDGE_CURVE('',#2994,#2983,#1964,.T.);
#3855=EDGE_CURVE('',#2984,#2992,#1965,.T.);
#3856=EDGE_CURVE('',#2995,#2996,#2503,.T.);
#3857=EDGE_CURVE('',#2995,#2997,#255,.T.);
#3858=EDGE_CURVE('',#2997,#2998,#256,.T.);
#3859=EDGE_CURVE('',#2999,#2998,#2504,.T.);
#3860=EDGE_CURVE('',#2999,#3000,#257,.T.);
#3861=EDGE_CURVE('',#3000,#3001,#258,.T.);
#3862=EDGE_CURVE('',#3002,#3001,#2505,.T.);
#3863=EDGE_CURVE('',#3002,#3003,#259,.T.);
#3864=EDGE_CURVE('',#3003,#3004,#260,.T.);
#3865=EDGE_CURVE('',#3005,#3004,#2506,.T.);
#3866=EDGE_CURVE('',#3005,#3006,#261,.T.);
#3867=EDGE_CURVE('',#3006,#3007,#262,.T.);
#3868=EDGE_CURVE('',#3008,#3007,#2507,.T.);
#3869=EDGE_CURVE('',#3008,#3009,#263,.T.);
#3870=EDGE_CURVE('',#3009,#3010,#264,.T.);
#3871=EDGE_CURVE('',#3011,#3010,#2508,.T.);
#3872=EDGE_CURVE('',#3011,#3012,#265,.T.);
#3873=EDGE_CURVE('',#3012,#3013,#266,.T.);
#3874=EDGE_CURVE('',#3014,#3013,#2509,.T.);
#3875=EDGE_CURVE('',#3014,#3015,#267,.T.);
#3876=EDGE_CURVE('',#3015,#3016,#268,.T.);
#3877=EDGE_CURVE('',#3017,#3016,#2510,.T.);
#3878=EDGE_CURVE('',#3017,#3018,#269,.T.);
#3879=EDGE_CURVE('',#3018,#3019,#270,.T.);
#3880=EDGE_CURVE('',#3020,#3019,#2511,.T.);
#3881=EDGE_CURVE('',#3020,#3021,#271,.T.);
#3882=EDGE_CURVE('',#3021,#3022,#272,.T.);
#3883=EDGE_CURVE('',#3023,#3022,#2512,.T.);
#3884=EDGE_CURVE('',#3023,#3024,#273,.T.);
#3885=EDGE_CURVE('',#3024,#3025,#274,.T.);
#3886=EDGE_CURVE('',#3026,#3025,#2513,.T.);
#3887=EDGE_CURVE('',#3026,#3027,#275,.T.);
#3888=EDGE_CURVE('',#3027,#3028,#276,.T.);
#3889=EDGE_CURVE('',#3029,#3028,#2514,.T.);
#3890=EDGE_CURVE('',#3029,#3030,#277,.T.);
#3891=EDGE_CURVE('',#3030,#3031,#278,.T.);
#3892=EDGE_CURVE('',#3032,#3031,#2515,.T.);
#3893=EDGE_CURVE('',#3032,#3033,#279,.T.);
#3894=EDGE_CURVE('',#3033,#3034,#280,.T.);
#3895=EDGE_CURVE('',#3035,#3034,#2516,.T.);
#3896=EDGE_CURVE('',#3035,#3036,#281,.T.);
#3897=EDGE_CURVE('',#3036,#3037,#282,.T.);
#3898=EDGE_CURVE('',#3038,#3037,#2517,.T.);
#3899=EDGE_CURVE('',#3038,#3039,#283,.T.);
#3900=EDGE_CURVE('',#3039,#3040,#284,.T.);
#3901=EDGE_CURVE('',#3041,#3040,#2518,.T.);
#3902=EDGE_CURVE('',#3041,#3042,#285,.T.);
#3903=EDGE_CURVE('',#3042,#3043,#286,.T.);
#3904=EDGE_CURVE('',#3044,#3043,#2519,.T.);
#3905=EDGE_CURVE('',#3044,#3045,#287,.T.);
#3906=EDGE_CURVE('',#3045,#3046,#288,.T.);
#3907=EDGE_CURVE('',#3047,#3046,#2520,.T.);
#3908=EDGE_CURVE('',#3047,#3048,#289,.T.);
#3909=EDGE_CURVE('',#3048,#3049,#290,.T.);
#3910=EDGE_CURVE('',#3050,#3049,#2521,.T.);
#3911=EDGE_CURVE('',#3050,#3051,#291,.T.);
#3912=EDGE_CURVE('',#3051,#3052,#292,.T.);
#3913=EDGE_CURVE('',#3053,#3052,#2522,.T.);
#3914=EDGE_CURVE('',#3053,#3054,#293,.T.);
#3915=EDGE_CURVE('',#3054,#2996,#294,.T.);
#3916=EDGE_CURVE('',#2993,#3055,#1966,.T.);
#3917=EDGE_CURVE('',#3055,#3055,#2523,.T.);
#3918=EDGE_CURVE('',#3056,#3056,#2524,.T.);
#3919=EDGE_CURVE('',#3056,#3057,#1967,.T.);
#3920=EDGE_CURVE('',#3057,#3058,#2525,.T.);
#3921=EDGE_CURVE('',#3058,#3057,#2526,.T.);
#3922=EDGE_CURVE('',#3058,#2980,#1968,.T.);
#3923=EDGE_CURVE('',#2978,#3059,#1969,.T.);
#3924=EDGE_CURVE('',#3059,#3059,#2527,.T.);
#3925=EDGE_CURVE('',#3060,#3061,#437,.T.);
#3926=EDGE_CURVE('',#3062,#3060,#438,.T.);
#3927=EDGE_CURVE('',#3061,#3062,#2528,.T.);
#3928=EDGE_CURVE('',#3063,#3064,#439,.T.);
#3929=EDGE_CURVE('',#3065,#3063,#440,.T.);
#3930=EDGE_CURVE('',#3064,#3065,#2529,.T.);
#3931=EDGE_CURVE('',#3066,#3067,#441,.T.);
#3932=EDGE_CURVE('',#3068,#3066,#442,.T.);
#3933=EDGE_CURVE('',#3067,#3068,#2530,.T.);
#3934=EDGE_CURVE('',#3069,#3070,#443,.T.);
#3935=EDGE_CURVE('',#3071,#3069,#444,.T.);
#3936=EDGE_CURVE('',#3070,#3071,#2531,.T.);
#3937=EDGE_CURVE('',#3072,#3073,#445,.T.);
#3938=EDGE_CURVE('',#3074,#3072,#446,.T.);
#3939=EDGE_CURVE('',#3073,#3074,#2532,.T.);
#3940=EDGE_CURVE('',#3075,#3076,#447,.T.);
#3941=EDGE_CURVE('',#3077,#3075,#448,.T.);
#3942=EDGE_CURVE('',#3076,#3077,#2533,.T.);
#3943=EDGE_CURVE('',#3078,#3079,#449,.T.);
#3944=EDGE_CURVE('',#3080,#3078,#450,.T.);
#3945=EDGE_CURVE('',#3079,#3080,#2534,.T.);
#3946=EDGE_CURVE('',#3081,#3082,#451,.T.);
#3947=EDGE_CURVE('',#3083,#3081,#452,.T.);
#3948=EDGE_CURVE('',#3082,#3083,#2535,.T.);
#3949=EDGE_CURVE('',#3084,#3085,#453,.T.);
#3950=EDGE_CURVE('',#3086,#3084,#454,.T.);
#3951=EDGE_CURVE('',#3085,#3086,#2536,.T.);
#3952=EDGE_CURVE('',#3087,#3088,#455,.T.);
#3953=EDGE_CURVE('',#3089,#3087,#456,.T.);
#3954=EDGE_CURVE('',#3088,#3089,#2537,.T.);
#3955=EDGE_CURVE('',#3090,#3091,#457,.T.);
#3956=EDGE_CURVE('',#3092,#3090,#458,.T.);
#3957=EDGE_CURVE('',#3091,#3092,#2538,.T.);
#3958=EDGE_CURVE('',#3093,#3094,#459,.T.);
#3959=EDGE_CURVE('',#3095,#3093,#460,.T.);
#3960=EDGE_CURVE('',#3094,#3095,#2539,.T.);
#3961=EDGE_CURVE('',#3096,#3097,#461,.T.);
#3962=EDGE_CURVE('',#3098,#3096,#462,.T.);
#3963=EDGE_CURVE('',#3097,#3098,#2540,.T.);
#3964=EDGE_CURVE('',#3099,#3100,#463,.T.);
#3965=EDGE_CURVE('',#3101,#3099,#464,.T.);
#3966=EDGE_CURVE('',#3100,#3101,#2541,.T.);
#3967=EDGE_CURVE('',#3102,#3103,#465,.T.);
#3968=EDGE_CURVE('',#3104,#3102,#466,.T.);
#3969=EDGE_CURVE('',#3103,#3104,#2542,.T.);
#3970=EDGE_CURVE('',#3105,#3106,#467,.T.);
#3971=EDGE_CURVE('',#3107,#3105,#468,.T.);
#3972=EDGE_CURVE('',#3106,#3107,#2543,.T.);
#3973=EDGE_CURVE('',#3108,#3109,#469,.T.);
#3974=EDGE_CURVE('',#3110,#3108,#470,.T.);
#3975=EDGE_CURVE('',#3109,#3110,#2544,.T.);
#3976=EDGE_CURVE('',#3111,#3112,#471,.T.);
#3977=EDGE_CURVE('',#3113,#3111,#472,.T.);
#3978=EDGE_CURVE('',#3112,#3113,#2545,.T.);
#3979=EDGE_CURVE('',#3114,#3115,#473,.T.);
#3980=EDGE_CURVE('',#3116,#3114,#474,.T.);
#3981=EDGE_CURVE('',#3115,#3116,#2546,.T.);
#3982=EDGE_CURVE('',#3117,#3117,#2547,.T.);
#3983=EDGE_CURVE('',#3117,#3118,#1970,.T.);
#3984=EDGE_CURVE('',#3118,#3118,#2548,.T.);
#3985=EDGE_CURVE('',#3118,#3119,#1971,.T.);
#3986=EDGE_CURVE('',#3119,#3119,#2549,.T.);
#3987=EDGE_CURVE('',#3120,#3121,#475,.T.);
#3988=EDGE_CURVE('',#3122,#3120,#476,.T.);
#3989=EDGE_CURVE('',#3121,#3122,#2550,.T.);
#3990=EDGE_CURVE('',#3054,#3120,#1972,.T.);
#3991=EDGE_CURVE('',#3123,#3053,#477,.T.);
#3992=EDGE_CURVE('',#3123,#3122,#295,.T.);
#3993=EDGE_CURVE('',#2997,#3114,#1973,.T.);
#3994=EDGE_CURVE('',#3124,#2995,#478,.T.);
#3995=EDGE_CURVE('',#3124,#3116,#296,.T.);
#3996=EDGE_CURVE('',#3000,#3111,#1974,.T.);
#3997=EDGE_CURVE('',#3125,#2999,#479,.T.);
#3998=EDGE_CURVE('',#3125,#3113,#297,.T.);
#3999=EDGE_CURVE('',#3003,#3108,#1975,.T.);
#4000=EDGE_CURVE('',#3126,#3002,#480,.T.);
#4001=EDGE_CURVE('',#3126,#3110,#298,.T.);
#4002=EDGE_CURVE('',#3006,#3105,#1976,.T.);
#4003=EDGE_CURVE('',#3127,#3005,#481,.T.);
#4004=EDGE_CURVE('',#3127,#3107,#299,.T.);
#4005=EDGE_CURVE('',#3009,#3102,#1977,.T.);
#4006=EDGE_CURVE('',#3128,#3008,#482,.T.);
#4007=EDGE_CURVE('',#3128,#3104,#300,.T.);
#4008=EDGE_CURVE('',#3012,#3099,#1978,.T.);
#4009=EDGE_CURVE('',#3129,#3011,#483,.T.);
#4010=EDGE_CURVE('',#3129,#3101,#301,.T.);
#4011=EDGE_CURVE('',#3015,#3096,#1979,.T.);
#4012=EDGE_CURVE('',#3130,#3014,#484,.T.);
#4013=EDGE_CURVE('',#3130,#3098,#302,.T.);
#4014=EDGE_CURVE('',#3018,#3093,#1980,.T.);
#4015=EDGE_CURVE('',#3131,#3017,#485,.T.);
#4016=EDGE_CURVE('',#3131,#3095,#303,.T.);
#4017=EDGE_CURVE('',#3021,#3090,#1981,.T.);
#4018=EDGE_CURVE('',#3132,#3020,#486,.T.);
#4019=EDGE_CURVE('',#3132,#3092,#304,.T.);
#4020=EDGE_CURVE('',#3024,#3087,#1982,.T.);
#4021=EDGE_CURVE('',#3133,#3023,#487,.T.);
#4022=EDGE_CURVE('',#3133,#3089,#305,.T.);
#4023=EDGE_CURVE('',#3027,#3084,#1983,.T.);
#4024=EDGE_CURVE('',#3134,#3026,#488,.T.);
#4025=EDGE_CURVE('',#3134,#3086,#306,.T.);
#4026=EDGE_CURVE('',#3030,#3081,#1984,.T.);
#4027=EDGE_CURVE('',#3135,#3029,#489,.T.);
#4028=EDGE_CURVE('',#3135,#3083,#307,.T.);
#4029=EDGE_CURVE('',#3033,#3078,#1985,.T.);
#4030=EDGE_CURVE('',#3136,#3032,#490,.T.);
#4031=EDGE_CURVE('',#3136,#3080,#308,.T.);
#4032=EDGE_CURVE('',#3036,#3075,#1986,.T.);
#4033=EDGE_CURVE('',#3137,#3035,#491,.T.);
#4034=EDGE_CURVE('',#3137,#3077,#309,.T.);
#4035=EDGE_CURVE('',#3039,#3072,#1987,.T.);
#4036=EDGE_CURVE('',#3138,#3038,#492,.T.);
#4037=EDGE_CURVE('',#3138,#3074,#310,.T.);
#4038=EDGE_CURVE('',#3042,#3069,#1988,.T.);
#4039=EDGE_CURVE('',#3139,#3041,#493,.T.);
#4040=EDGE_CURVE('',#3139,#3071,#311,.T.);
#4041=EDGE_CURVE('',#3045,#3066,#1989,.T.);
#4042=EDGE_CURVE('',#3140,#3044,#494,.T.);
#4043=EDGE_CURVE('',#3140,#3068,#312,.T.);
#4044=EDGE_CURVE('',#3048,#3063,#1990,.T.);
#4045=EDGE_CURVE('',#3141,#3047,#495,.T.);
#4046=EDGE_CURVE('',#3141,#3065,#313,.T.);
#4047=EDGE_CURVE('',#3051,#3060,#1991,.T.);
#4048=EDGE_CURVE('',#3142,#3050,#496,.T.);
#4049=EDGE_CURVE('',#3142,#3062,#314,.T.);
#4050=EDGE_CURVE('',#3121,#3143,#315,.T.);
#4051=EDGE_CURVE('',#2996,#3143,#497,.T.);
#4052=EDGE_CURVE('',#3143,#3123,#2551,.T.);
#4053=EDGE_CURVE('',#3117,#3144,#1992,.T.);
#4054=EDGE_CURVE('',#3144,#3132,#2552,.T.);
#4055=EDGE_CURVE('',#3019,#3145,#498,.T.);
#4056=EDGE_CURVE('',#3145,#3131,#2553,.T.);
#4057=EDGE_CURVE('',#3016,#3146,#499,.T.);
#4058=EDGE_CURVE('',#3146,#3130,#2554,.T.);
#4059=EDGE_CURVE('',#3013,#3147,#500,.T.);
#4060=EDGE_CURVE('',#3147,#3129,#2555,.T.);
#4061=EDGE_CURVE('',#3010,#3148,#501,.T.);
#4062=EDGE_CURVE('',#3148,#3128,#2556,.T.);
#4063=EDGE_CURVE('',#3007,#3149,#502,.T.);
#4064=EDGE_CURVE('',#3149,#3127,#2557,.T.);
#4065=EDGE_CURVE('',#3004,#3150,#503,.T.);
#4066=EDGE_CURVE('',#3150,#3126,#2558,.T.);
#4067=EDGE_CURVE('',#3001,#3151,#504,.T.);
#4068=EDGE_CURVE('',#3151,#3125,#2559,.T.);
#4069=EDGE_CURVE('',#2998,#3152,#505,.T.);
#4070=EDGE_CURVE('',#3152,#3124,#2560,.T.);
#4071=EDGE_CURVE('',#3052,#3153,#506,.T.);
#4072=EDGE_CURVE('',#3153,#3142,#2561,.T.);
#4073=EDGE_CURVE('',#3049,#3154,#507,.T.);
#4074=EDGE_CURVE('',#3154,#3141,#2562,.T.);
#4075=EDGE_CURVE('',#3046,#3155,#508,.T.);
#4076=EDGE_CURVE('',#3155,#3140,#2563,.T.);
#4077=EDGE_CURVE('',#3043,#3156,#509,.T.);
#4078=EDGE_CURVE('',#3156,#3139,#2564,.T.);
#4079=EDGE_CURVE('',#3040,#3157,#510,.T.);
#4080=EDGE_CURVE('',#3157,#3138,#2565,.T.);
#4081=EDGE_CURVE('',#3037,#3158,#511,.T.);
#4082=EDGE_CURVE('',#3158,#3137,#2566,.T.);
#4083=EDGE_CURVE('',#3034,#3159,#512,.T.);
#4084=EDGE_CURVE('',#3159,#3136,#2567,.T.);
#4085=EDGE_CURVE('',#3031,#3160,#513,.T.);
#4086=EDGE_CURVE('',#3160,#3135,#2568,.T.);
#4087=EDGE_CURVE('',#3028,#3161,#514,.T.);
#4088=EDGE_CURVE('',#3161,#3134,#2569,.T.);
#4089=EDGE_CURVE('',#3025,#3162,#515,.T.);
#4090=EDGE_CURVE('',#3162,#3133,#2570,.T.);
#4091=EDGE_CURVE('',#3022,#3163,#516,.T.);
#4092=EDGE_CURVE('',#3163,#3144,#2571,.T.);
#4093=EDGE_CURVE('',#3115,#3152,#316,.T.);
#4094=EDGE_CURVE('',#3112,#3151,#317,.T.);
#4095=EDGE_CURVE('',#3109,#3150,#318,.T.);
#4096=EDGE_CURVE('',#3106,#3149,#319,.T.);
#4097=EDGE_CURVE('',#3103,#3148,#320,.T.);
#4098=EDGE_CURVE('',#3100,#3147,#321,.T.);
#4099=EDGE_CURVE('',#3097,#3146,#322,.T.);
#4100=EDGE_CURVE('',#3094,#3145,#323,.T.);
#4101=EDGE_CURVE('',#3091,#3163,#324,.T.);
#4102=EDGE_CURVE('',#3088,#3162,#325,.T.);
#4103=EDGE_CURVE('',#3085,#3161,#326,.T.);
#4104=EDGE_CURVE('',#3082,#3160,#327,.T.);
#4105=EDGE_CURVE('',#3079,#3159,#328,.T.);
#4106=EDGE_CURVE('',#3076,#3158,#329,.T.);
#4107=EDGE_CURVE('',#3073,#3157,#330,.T.);
#4108=EDGE_CURVE('',#3070,#3156,#331,.T.);
#4109=EDGE_CURVE('',#3067,#3155,#332,.T.);
#4110=EDGE_CURVE('',#3064,#3154,#333,.T.);
#4111=EDGE_CURVE('',#3061,#3153,#334,.T.);
#5313=ORIENTED_EDGE('',*,*,#3832,.F.);
#5314=ORIENTED_EDGE('',*,*,#3833,.F.);
#5315=ORIENTED_EDGE('',*,*,#3834,.F.);
#5316=ORIENTED_EDGE('',*,*,#3835,.T.);
#5317=ORIENTED_EDGE('',*,*,#3836,.T.);
#5318=ORIENTED_EDGE('',*,*,#3835,.F.);
#5319=ORIENTED_EDGE('',*,*,#3836,.F.);
#5320=ORIENTED_EDGE('',*,*,#3837,.T.);
#5321=ORIENTED_EDGE('',*,*,#3838,.F.);
#5322=ORIENTED_EDGE('',*,*,#3839,.F.);
#5323=ORIENTED_EDGE('',*,*,#3840,.F.);
#5324=ORIENTED_EDGE('',*,*,#3837,.F.);
#5325=ORIENTED_EDGE('',*,*,#3841,.F.);
#5326=ORIENTED_EDGE('',*,*,#3842,.T.);
#5327=ORIENTED_EDGE('',*,*,#3843,.T.);
#5328=ORIENTED_EDGE('',*,*,#3842,.F.);
#5329=ORIENTED_EDGE('',*,*,#3844,.F.);
#5330=ORIENTED_EDGE('',*,*,#3843,.F.);
#5331=ORIENTED_EDGE('',*,*,#3845,.T.);
#5332=ORIENTED_EDGE('',*,*,#3846,.F.);
#5333=ORIENTED_EDGE('',*,*,#3847,.F.);
#5334=ORIENTED_EDGE('',*,*,#3845,.F.);
#5335=ORIENTED_EDGE('',*,*,#3848,.T.);
#5336=ORIENTED_EDGE('',*,*,#3849,.T.);
#5337=ORIENTED_EDGE('',*,*,#3850,.T.);
#5338=ORIENTED_EDGE('',*,*,#3851,.T.);
#5339=ORIENTED_EDGE('',*,*,#3849,.F.);
#5340=ORIENTED_EDGE('',*,*,#3852,.F.);
#5341=ORIENTED_EDGE('',*,*,#3853,.F.);
#5342=ORIENTED_EDGE('',*,*,#3854,.T.);
#5343=ORIENTED_EDGE('',*,*,#3838,.T.);
#5344=ORIENTED_EDGE('',*,*,#3840,.T.);
#5345=ORIENTED_EDGE('',*,*,#3855,.T.);
#5346=ORIENTED_EDGE('',*,*,#3850,.F.);
#5347=ORIENTED_EDGE('',*,*,#3851,.F.);
#5348=ORIENTED_EDGE('',*,*,#3855,.F.);
#5349=ORIENTED_EDGE('',*,*,#3839,.T.);
#5350=ORIENTED_EDGE('',*,*,#3854,.F.);
#5351=ORIENTED_EDGE('',*,*,#3846,.T.);
#5352=ORIENTED_EDGE('',*,*,#3847,.T.);
#5353=ORIENTED_EDGE('',*,*,#3856,.F.);
#5354=ORIENTED_EDGE('',*,*,#3857,.T.);
#5355=ORIENTED_EDGE('',*,*,#3858,.T.);
#5356=ORIENTED_EDGE('',*,*,#3859,.F.);
#5357=ORIENTED_EDGE('',*,*,#3860,.T.);
#5358=ORIENTED_EDGE('',*,*,#3861,.T.);
#5359=ORIENTED_EDGE('',*,*,#3862,.F.);
#5360=ORIENTED_EDGE('',*,*,#3863,.T.);
#5361=ORIENTED_EDGE('',*,*,#3864,.T.);
#5362=ORIENTED_EDGE('',*,*,#3865,.F.);
#5363=ORIENTED_EDGE('',*,*,#3866,.T.);
#5364=ORIENTED_EDGE('',*,*,#3867,.T.);
#5365=ORIENTED_EDGE('',*,*,#3868,.F.);
#5366=ORIENTED_EDGE('',*,*,#3869,.T.);
#5367=ORIENTED_EDGE('',*,*,#3870,.T.);
#5368=ORIENTED_EDGE('',*,*,#3871,.F.);
#5369=ORIENTED_EDGE('',*,*,#3872,.T.);
#5370=ORIENTED_EDGE('',*,*,#3873,.T.);
#5371=ORIENTED_EDGE('',*,*,#3874,.F.);
#5372=ORIENTED_EDGE('',*,*,#3875,.T.);
#5373=ORIENTED_EDGE('',*,*,#3876,.T.);
#5374=ORIENTED_EDGE('',*,*,#3877,.F.);
#5375=ORIENTED_EDGE('',*,*,#3878,.T.);
#5376=ORIENTED_EDGE('',*,*,#3879,.T.);
#5377=ORIENTED_EDGE('',*,*,#3880,.F.);
#5378=ORIENTED_EDGE('',*,*,#3881,.T.);
#5379=ORIENTED_EDGE('',*,*,#3882,.T.);
#5380=ORIENTED_EDGE('',*,*,#3883,.F.);
#5381=ORIENTED_EDGE('',*,*,#3884,.T.);
#5382=ORIENTED_EDGE('',*,*,#3885,.T.);
#5383=ORIENTED_EDGE('',*,*,#3886,.F.);
#5384=ORIENTED_EDGE('',*,*,#3887,.T.);
#5385=ORIENTED_EDGE('',*,*,#3888,.T.);
#5386=ORIENTED_EDGE('',*,*,#3889,.F.);
#5387=ORIENTED_EDGE('',*,*,#3890,.T.);
#5388=ORIENTED_EDGE('',*,*,#3891,.T.);
#5389=ORIENTED_EDGE('',*,*,#3892,.F.);
#5390=ORIENTED_EDGE('',*,*,#3893,.T.);
#5391=ORIENTED_EDGE('',*,*,#3894,.T.);
#5392=ORIENTED_EDGE('',*,*,#3895,.F.);
#5393=ORIENTED_EDGE('',*,*,#3896,.T.);
#5394=ORIENTED_EDGE('',*,*,#3897,.T.);
#5395=ORIENTED_EDGE('',*,*,#3898,.F.);
#5396=ORIENTED_EDGE('',*,*,#3899,.T.);
#5397=ORIENTED_EDGE('',*,*,#3900,.T.);
#5398=ORIENTED_EDGE('',*,*,#3901,.F.);
#5399=ORIENTED_EDGE('',*,*,#3902,.T.);
#5400=ORIENTED_EDGE('',*,*,#3903,.T.);
#5401=ORIENTED_EDGE('',*,*,#3904,.F.);
#5402=ORIENTED_EDGE('',*,*,#3905,.T.);
#5403=ORIENTED_EDGE('',*,*,#3906,.T.);
#5404=ORIENTED_EDGE('',*,*,#3907,.F.);
#5405=ORIENTED_EDGE('',*,*,#3908,.T.);
#5406=ORIENTED_EDGE('',*,*,#3909,.T.);
#5407=ORIENTED_EDGE('',*,*,#3910,.F.);
#5408=ORIENTED_EDGE('',*,*,#3911,.T.);
#5409=ORIENTED_EDGE('',*,*,#3912,.T.);
#5410=ORIENTED_EDGE('',*,*,#3913,.F.);
#5411=ORIENTED_EDGE('',*,*,#3914,.T.);
#5412=ORIENTED_EDGE('',*,*,#3915,.T.);
#5413=ORIENTED_EDGE('',*,*,#3848,.F.);
#5414=ORIENTED_EDGE('',*,*,#3852,.T.);
#5415=ORIENTED_EDGE('',*,*,#3853,.T.);
#5416=ORIENTED_EDGE('',*,*,#3916,.T.);
#5417=ORIENTED_EDGE('',*,*,#3917,.T.);
#5418=ORIENTED_EDGE('',*,*,#3916,.F.);
#5419=ORIENTED_EDGE('',*,*,#3918,.F.);
#5420=ORIENTED_EDGE('',*,*,#3917,.F.);
#5421=ORIENTED_EDGE('',*,*,#3918,.T.);
#5422=ORIENTED_EDGE('',*,*,#3919,.T.);
#5423=ORIENTED_EDGE('',*,*,#3920,.T.);
#5424=ORIENTED_EDGE('',*,*,#3921,.T.);
#5425=ORIENTED_EDGE('',*,*,#3919,.F.);
#5426=ORIENTED_EDGE('',*,*,#3920,.F.);
#5427=ORIENTED_EDGE('',*,*,#3921,.F.);
#5428=ORIENTED_EDGE('',*,*,#3922,.T.);
#5429=ORIENTED_EDGE('',*,*,#3833,.T.);
#5430=ORIENTED_EDGE('',*,*,#3923,.T.);
#5431=ORIENTED_EDGE('',*,*,#3924,.T.);
#5432=ORIENTED_EDGE('',*,*,#3923,.F.);
#5433=ORIENTED_EDGE('',*,*,#3832,.T.);
#5434=ORIENTED_EDGE('',*,*,#3834,.T.);
#5435=ORIENTED_EDGE('',*,*,#3922,.F.);
#5436=ORIENTED_EDGE('',*,*,#3841,.T.);
#5437=ORIENTED_EDGE('',*,*,#3844,.T.);
#5438=ORIENTED_EDGE('',*,*,#3925,.F.);
#5439=ORIENTED_EDGE('',*,*,#3926,.F.);
#5440=ORIENTED_EDGE('',*,*,#3927,.F.);
#5441=ORIENTED_EDGE('',*,*,#3928,.F.);
#5442=ORIENTED_EDGE('',*,*,#3929,.F.);
#5443=ORIENTED_EDGE('',*,*,#3930,.F.);
#5444=ORIENTED_EDGE('',*,*,#3931,.F.);
#5445=ORIENTED_EDGE('',*,*,#3932,.F.);
#5446=ORIENTED_EDGE('',*,*,#3933,.F.);
#5447=ORIENTED_EDGE('',*,*,#3934,.F.);
#5448=ORIENTED_EDGE('',*,*,#3935,.F.);
#5449=ORIENTED_EDGE('',*,*,#3936,.F.);
#5450=ORIENTED_EDGE('',*,*,#3937,.F.);
#5451=ORIENTED_EDGE('',*,*,#3938,.F.);
#5452=ORIENTED_EDGE('',*,*,#3939,.F.);
#5453=ORIENTED_EDGE('',*,*,#3940,.F.);
#5454=ORIENTED_EDGE('',*,*,#3941,.F.);
#5455=ORIENTED_EDGE('',*,*,#3942,.F.);
#5456=ORIENTED_EDGE('',*,*,#3943,.F.);
#5457=ORIENTED_EDGE('',*,*,#3944,.F.);
#5458=ORIENTED_EDGE('',*,*,#3945,.F.);
#5459=ORIENTED_EDGE('',*,*,#3946,.F.);
#5460=ORIENTED_EDGE('',*,*,#3947,.F.);
#5461=ORIENTED_EDGE('',*,*,#3948,.F.);
#5462=ORIENTED_EDGE('',*,*,#3949,.F.);
#5463=ORIENTED_EDGE('',*,*,#3950,.F.);
#5464=ORIENTED_EDGE('',*,*,#3951,.F.);
#5465=ORIENTED_EDGE('',*,*,#3952,.F.);
#5466=ORIENTED_EDGE('',*,*,#3953,.F.);
#5467=ORIENTED_EDGE('',*,*,#3954,.F.);
#5468=ORIENTED_EDGE('',*,*,#3955,.F.);
#5469=ORIENTED_EDGE('',*,*,#3956,.F.);
#5470=ORIENTED_EDGE('',*,*,#3957,.F.);
#5471=ORIENTED_EDGE('',*,*,#3958,.F.);
#5472=ORIENTED_EDGE('',*,*,#3959,.F.);
#5473=ORIENTED_EDGE('',*,*,#3960,.F.);
#5474=ORIENTED_EDGE('',*,*,#3961,.F.);
#5475=ORIENTED_EDGE('',*,*,#3962,.F.);
#5476=ORIENTED_EDGE('',*,*,#3963,.F.);
#5477=ORIENTED_EDGE('',*,*,#3964,.F.);
#5478=ORIENTED_EDGE('',*,*,#3965,.F.);
#5479=ORIENTED_EDGE('',*,*,#3966,.F.);
#5480=ORIENTED_EDGE('',*,*,#3967,.F.);
#5481=ORIENTED_EDGE('',*,*,#3968,.F.);
#5482=ORIENTED_EDGE('',*,*,#3969,.F.);
#5483=ORIENTED_EDGE('',*,*,#3970,.F.);
#5484=ORIENTED_EDGE('',*,*,#3971,.F.);
#5485=ORIENTED_EDGE('',*,*,#3972,.F.);
#5486=ORIENTED_EDGE('',*,*,#3973,.F.);
#5487=ORIENTED_EDGE('',*,*,#3974,.F.);
#5488=ORIENTED_EDGE('',*,*,#3975,.F.);
#5489=ORIENTED_EDGE('',*,*,#3976,.F.);
#5490=ORIENTED_EDGE('',*,*,#3977,.F.);
#5491=ORIENTED_EDGE('',*,*,#3978,.F.);
#5492=ORIENTED_EDGE('',*,*,#3979,.F.);
#5493=ORIENTED_EDGE('',*,*,#3980,.F.);
#5494=ORIENTED_EDGE('',*,*,#3981,.F.);
#5495=ORIENTED_EDGE('',*,*,#3982,.F.);
#5496=ORIENTED_EDGE('',*,*,#3983,.T.);
#5497=ORIENTED_EDGE('',*,*,#3984,.F.);
#5498=ORIENTED_EDGE('',*,*,#3983,.F.);
#5499=ORIENTED_EDGE('',*,*,#3984,.T.);
#5500=ORIENTED_EDGE('',*,*,#3985,.T.);
#5501=ORIENTED_EDGE('',*,*,#3986,.F.);
#5502=ORIENTED_EDGE('',*,*,#3985,.F.);
#5503=ORIENTED_EDGE('',*,*,#3987,.F.);
#5504=ORIENTED_EDGE('',*,*,#3988,.F.);
#5505=ORIENTED_EDGE('',*,*,#3989,.F.);
#5506=ORIENTED_EDGE('',*,*,#3988,.T.);
#5507=ORIENTED_EDGE('',*,*,#3990,.F.);
#5508=ORIENTED_EDGE('',*,*,#3914,.F.);
#5509=ORIENTED_EDGE('',*,*,#3991,.F.);
#5510=ORIENTED_EDGE('',*,*,#3992,.T.);
#5511=ORIENTED_EDGE('',*,*,#3980,.T.);
#5512=ORIENTED_EDGE('',*,*,#3993,.F.);
#5513=ORIENTED_EDGE('',*,*,#3857,.F.);
#5514=ORIENTED_EDGE('',*,*,#3994,.F.);
#5515=ORIENTED_EDGE('',*,*,#3995,.T.);
#5516=ORIENTED_EDGE('',*,*,#3977,.T.);
#5517=ORIENTED_EDGE('',*,*,#3996,.F.);
#5518=ORIENTED_EDGE('',*,*,#3860,.F.);
#5519=ORIENTED_EDGE('',*,*,#3997,.F.);
#5520=ORIENTED_EDGE('',*,*,#3998,.T.);
#5521=ORIENTED_EDGE('',*,*,#3974,.T.);
#5522=ORIENTED_EDGE('',*,*,#3999,.F.);
#5523=ORIENTED_EDGE('',*,*,#3863,.F.);
#5524=ORIENTED_EDGE('',*,*,#4000,.F.);
#5525=ORIENTED_EDGE('',*,*,#4001,.T.);
#5526=ORIENTED_EDGE('',*,*,#3971,.T.);
#5527=ORIENTED_EDGE('',*,*,#4002,.F.);
#5528=ORIENTED_EDGE('',*,*,#3866,.F.);
#5529=ORIENTED_EDGE('',*,*,#4003,.F.);
#5530=ORIENTED_EDGE('',*,*,#4004,.T.);
#5531=ORIENTED_EDGE('',*,*,#3968,.T.);
#5532=ORIENTED_EDGE('',*,*,#4005,.F.);
#5533=ORIENTED_EDGE('',*,*,#3869,.F.);
#5534=ORIENTED_EDGE('',*,*,#4006,.F.);
#5535=ORIENTED_EDGE('',*,*,#4007,.T.);
#5536=ORIENTED_EDGE('',*,*,#3965,.T.);
#5537=ORIENTED_EDGE('',*,*,#4008,.F.);
#5538=ORIENTED_EDGE('',*,*,#3872,.F.);
#5539=ORIENTED_EDGE('',*,*,#4009,.F.);
#5540=ORIENTED_EDGE('',*,*,#4010,.T.);
#5541=ORIENTED_EDGE('',*,*,#3962,.T.);
#5542=ORIENTED_EDGE('',*,*,#4011,.F.);
#5543=ORIENTED_EDGE('',*,*,#3875,.F.);
#5544=ORIENTED_EDGE('',*,*,#4012,.F.);
#5545=ORIENTED_EDGE('',*,*,#4013,.T.);
#5546=ORIENTED_EDGE('',*,*,#3959,.T.);
#5547=ORIENTED_EDGE('',*,*,#4014,.F.);
#5548=ORIENTED_EDGE('',*,*,#3878,.F.);
#5549=ORIENTED_EDGE('',*,*,#4015,.F.);
#5550=ORIENTED_EDGE('',*,*,#4016,.T.);
#5551=ORIENTED_EDGE('',*,*,#3956,.T.);
#5552=ORIENTED_EDGE('',*,*,#4017,.F.);
#5553=ORIENTED_EDGE('',*,*,#3881,.F.);
#5554=ORIENTED_EDGE('',*,*,#4018,.F.);
#5555=ORIENTED_EDGE('',*,*,#4019,.T.);
#5556=ORIENTED_EDGE('',*,*,#3953,.T.);
#5557=ORIENTED_EDGE('',*,*,#4020,.F.);
#5558=ORIENTED_EDGE('',*,*,#3884,.F.);
#5559=ORIENTED_EDGE('',*,*,#4021,.F.);
#5560=ORIENTED_EDGE('',*,*,#4022,.T.);
#5561=ORIENTED_EDGE('',*,*,#3950,.T.);
#5562=ORIENTED_EDGE('',*,*,#4023,.F.);
#5563=ORIENTED_EDGE('',*,*,#3887,.F.);
#5564=ORIENTED_EDGE('',*,*,#4024,.F.);
#5565=ORIENTED_EDGE('',*,*,#4025,.T.);
#5566=ORIENTED_EDGE('',*,*,#3947,.T.);
#5567=ORIENTED_EDGE('',*,*,#4026,.F.);
#5568=ORIENTED_EDGE('',*,*,#3890,.F.);
#5569=ORIENTED_EDGE('',*,*,#4027,.F.);
#5570=ORIENTED_EDGE('',*,*,#4028,.T.);
#5571=ORIENTED_EDGE('',*,*,#3944,.T.);
#5572=ORIENTED_EDGE('',*,*,#4029,.F.);
#5573=ORIENTED_EDGE('',*,*,#3893,.F.);
#5574=ORIENTED_EDGE('',*,*,#4030,.F.);
#5575=ORIENTED_EDGE('',*,*,#4031,.T.);
#5576=ORIENTED_EDGE('',*,*,#3941,.T.);
#5577=ORIENTED_EDGE('',*,*,#4032,.F.);
#5578=ORIENTED_EDGE('',*,*,#3896,.F.);
#5579=ORIENTED_EDGE('',*,*,#4033,.F.);
#5580=ORIENTED_EDGE('',*,*,#4034,.T.);
#5581=ORIENTED_EDGE('',*,*,#3938,.T.);
#5582=ORIENTED_EDGE('',*,*,#4035,.F.);
#5583=ORIENTED_EDGE('',*,*,#3899,.F.);
#5584=ORIENTED_EDGE('',*,*,#4036,.F.);
#5585=ORIENTED_EDGE('',*,*,#4037,.T.);
#5586=ORIENTED_EDGE('',*,*,#3935,.T.);
#5587=ORIENTED_EDGE('',*,*,#4038,.F.);
#5588=ORIENTED_EDGE('',*,*,#3902,.F.);
#5589=ORIENTED_EDGE('',*,*,#4039,.F.);
#5590=ORIENTED_EDGE('',*,*,#4040,.T.);
#5591=ORIENTED_EDGE('',*,*,#3932,.T.);
#5592=ORIENTED_EDGE('',*,*,#4041,.F.);
#5593=ORIENTED_EDGE('',*,*,#3905,.F.);
#5594=ORIENTED_EDGE('',*,*,#4042,.F.);
#5595=ORIENTED_EDGE('',*,*,#4043,.T.);
#5596=ORIENTED_EDGE('',*,*,#3929,.T.);
#5597=ORIENTED_EDGE('',*,*,#4044,.F.);
#5598=ORIENTED_EDGE('',*,*,#3908,.F.);
#5599=ORIENTED_EDGE('',*,*,#4045,.F.);
#5600=ORIENTED_EDGE('',*,*,#4046,.T.);
#5601=ORIENTED_EDGE('',*,*,#3926,.T.);
#5602=ORIENTED_EDGE('',*,*,#4047,.F.);
#5603=ORIENTED_EDGE('',*,*,#3911,.F.);
#5604=ORIENTED_EDGE('',*,*,#4048,.F.);
#5605=ORIENTED_EDGE('',*,*,#4049,.T.);
#5606=ORIENTED_EDGE('',*,*,#3987,.T.);
#5607=ORIENTED_EDGE('',*,*,#4050,.T.);
#5608=ORIENTED_EDGE('',*,*,#4051,.F.);
#5609=ORIENTED_EDGE('',*,*,#3915,.F.);
#5610=ORIENTED_EDGE('',*,*,#3990,.T.);
#5611=ORIENTED_EDGE('',*,*,#3989,.T.);
#5612=ORIENTED_EDGE('',*,*,#3992,.F.);
#5613=ORIENTED_EDGE('',*,*,#4052,.F.);
#5614=ORIENTED_EDGE('',*,*,#4050,.F.);
#5615=ORIENTED_EDGE('',*,*,#3982,.T.);
#5616=ORIENTED_EDGE('',*,*,#4053,.T.);
#5617=ORIENTED_EDGE('',*,*,#4054,.T.);
#5618=ORIENTED_EDGE('',*,*,#4018,.T.);
#5619=ORIENTED_EDGE('',*,*,#3880,.T.);
#5620=ORIENTED_EDGE('',*,*,#4055,.T.);
#5621=ORIENTED_EDGE('',*,*,#4056,.T.);
#5622=ORIENTED_EDGE('',*,*,#4015,.T.);
#5623=ORIENTED_EDGE('',*,*,#3877,.T.);
#5624=ORIENTED_EDGE('',*,*,#4057,.T.);
#5625=ORIENTED_EDGE('',*,*,#4058,.T.);
#5626=ORIENTED_EDGE('',*,*,#4012,.T.);
#5627=ORIENTED_EDGE('',*,*,#3874,.T.);
#5628=ORIENTED_EDGE('',*,*,#4059,.T.);
#5629=ORIENTED_EDGE('',*,*,#4060,.T.);
#5630=ORIENTED_EDGE('',*,*,#4009,.T.);
#5631=ORIENTED_EDGE('',*,*,#3871,.T.);
#5632=ORIENTED_EDGE('',*,*,#4061,.T.);
#5633=ORIENTED_EDGE('',*,*,#4062,.T.);
#5634=ORIENTED_EDGE('',*,*,#4006,.T.);
#5635=ORIENTED_EDGE('',*,*,#3868,.T.);
#5636=ORIENTED_EDGE('',*,*,#4063,.T.);
#5637=ORIENTED_EDGE('',*,*,#4064,.T.);
#5638=ORIENTED_EDGE('',*,*,#4003,.T.);
#5639=ORIENTED_EDGE('',*,*,#3865,.T.);
#5640=ORIENTED_EDGE('',*,*,#4065,.T.);
#5641=ORIENTED_EDGE('',*,*,#4066,.T.);
#5642=ORIENTED_EDGE('',*,*,#4000,.T.);
#5643=ORIENTED_EDGE('',*,*,#3862,.T.);
#5644=ORIENTED_EDGE('',*,*,#4067,.T.);
#5645=ORIENTED_EDGE('',*,*,#4068,.T.);
#5646=ORIENTED_EDGE('',*,*,#3997,.T.);
#5647=ORIENTED_EDGE('',*,*,#3859,.T.);
#5648=ORIENTED_EDGE('',*,*,#4069,.T.);
#5649=ORIENTED_EDGE('',*,*,#4070,.T.);
#5650=ORIENTED_EDGE('',*,*,#3994,.T.);
#5651=ORIENTED_EDGE('',*,*,#3856,.T.);
#5652=ORIENTED_EDGE('',*,*,#4051,.T.);
#5653=ORIENTED_EDGE('',*,*,#4052,.T.);
#5654=ORIENTED_EDGE('',*,*,#3991,.T.);
#5655=ORIENTED_EDGE('',*,*,#3913,.T.);
#5656=ORIENTED_EDGE('',*,*,#4071,.T.);
#5657=ORIENTED_EDGE('',*,*,#4072,.T.);
#5658=ORIENTED_EDGE('',*,*,#4048,.T.);
#5659=ORIENTED_EDGE('',*,*,#3910,.T.);
#5660=ORIENTED_EDGE('',*,*,#4073,.T.);
#5661=ORIENTED_EDGE('',*,*,#4074,.T.);
#5662=ORIENTED_EDGE('',*,*,#4045,.T.);
#5663=ORIENTED_EDGE('',*,*,#3907,.T.);
#5664=ORIENTED_EDGE('',*,*,#4075,.T.);
#5665=ORIENTED_EDGE('',*,*,#4076,.T.);
#5666=ORIENTED_EDGE('',*,*,#4042,.T.);
#5667=ORIENTED_EDGE('',*,*,#3904,.T.);
#5668=ORIENTED_EDGE('',*,*,#4077,.T.);
#5669=ORIENTED_EDGE('',*,*,#4078,.T.);
#5670=ORIENTED_EDGE('',*,*,#4039,.T.);
#5671=ORIENTED_EDGE('',*,*,#3901,.T.);
#5672=ORIENTED_EDGE('',*,*,#4079,.T.);
#5673=ORIENTED_EDGE('',*,*,#4080,.T.);
#5674=ORIENTED_EDGE('',*,*,#4036,.T.);
#5675=ORIENTED_EDGE('',*,*,#3898,.T.);
#5676=ORIENTED_EDGE('',*,*,#4081,.T.);
#5677=ORIENTED_EDGE('',*,*,#4082,.T.);
#5678=ORIENTED_EDGE('',*,*,#4033,.T.);
#5679=ORIENTED_EDGE('',*,*,#3895,.T.);
#5680=ORIENTED_EDGE('',*,*,#4083,.T.);
#5681=ORIENTED_EDGE('',*,*,#4084,.T.);
#5682=ORIENTED_EDGE('',*,*,#4030,.T.);
#5683=ORIENTED_EDGE('',*,*,#3892,.T.);
#5684=ORIENTED_EDGE('',*,*,#4085,.T.);
#5685=ORIENTED_EDGE('',*,*,#4086,.T.);
#5686=ORIENTED_EDGE('',*,*,#4027,.T.);
#5687=ORIENTED_EDGE('',*,*,#3889,.T.);
#5688=ORIENTED_EDGE('',*,*,#4087,.T.);
#5689=ORIENTED_EDGE('',*,*,#4088,.T.);
#5690=ORIENTED_EDGE('',*,*,#4024,.T.);
#5691=ORIENTED_EDGE('',*,*,#3886,.T.);
#5692=ORIENTED_EDGE('',*,*,#4089,.T.);
#5693=ORIENTED_EDGE('',*,*,#4090,.T.);
#5694=ORIENTED_EDGE('',*,*,#4021,.T.);
#5695=ORIENTED_EDGE('',*,*,#3883,.T.);
#5696=ORIENTED_EDGE('',*,*,#4091,.T.);
#5697=ORIENTED_EDGE('',*,*,#4092,.T.);
#5698=ORIENTED_EDGE('',*,*,#4053,.F.);
#5699=ORIENTED_EDGE('',*,*,#3979,.T.);
#5700=ORIENTED_EDGE('',*,*,#4093,.T.);
#5701=ORIENTED_EDGE('',*,*,#4069,.F.);
#5702=ORIENTED_EDGE('',*,*,#3858,.F.);
#5703=ORIENTED_EDGE('',*,*,#3993,.T.);
#5704=ORIENTED_EDGE('',*,*,#3981,.T.);
#5705=ORIENTED_EDGE('',*,*,#3995,.F.);
#5706=ORIENTED_EDGE('',*,*,#4070,.F.);
#5707=ORIENTED_EDGE('',*,*,#4093,.F.);
#5708=ORIENTED_EDGE('',*,*,#3976,.T.);
#5709=ORIENTED_EDGE('',*,*,#4094,.T.);
#5710=ORIENTED_EDGE('',*,*,#4067,.F.);
#5711=ORIENTED_EDGE('',*,*,#3861,.F.);
#5712=ORIENTED_EDGE('',*,*,#3996,.T.);
#5713=ORIENTED_EDGE('',*,*,#3978,.T.);
#5714=ORIENTED_EDGE('',*,*,#3998,.F.);
#5715=ORIENTED_EDGE('',*,*,#4068,.F.);
#5716=ORIENTED_EDGE('',*,*,#4094,.F.);
#5717=ORIENTED_EDGE('',*,*,#3973,.T.);
#5718=ORIENTED_EDGE('',*,*,#4095,.T.);
#5719=ORIENTED_EDGE('',*,*,#4065,.F.);
#5720=ORIENTED_EDGE('',*,*,#3864,.F.);
#5721=ORIENTED_EDGE('',*,*,#3999,.T.);
#5722=ORIENTED_EDGE('',*,*,#3975,.T.);
#5723=ORIENTED_EDGE('',*,*,#4001,.F.);
#5724=ORIENTED_EDGE('',*,*,#4066,.F.);
#5725=ORIENTED_EDGE('',*,*,#4095,.F.);
#5726=ORIENTED_EDGE('',*,*,#3970,.T.);
#5727=ORIENTED_EDGE('',*,*,#4096,.T.);
#5728=ORIENTED_EDGE('',*,*,#4063,.F.);
#5729=ORIENTED_EDGE('',*,*,#3867,.F.);
#5730=ORIENTED_EDGE('',*,*,#4002,.T.);
#5731=ORIENTED_EDGE('',*,*,#3972,.T.);
#5732=ORIENTED_EDGE('',*,*,#4004,.F.);
#5733=ORIENTED_EDGE('',*,*,#4064,.F.);
#5734=ORIENTED_EDGE('',*,*,#4096,.F.);
#5735=ORIENTED_EDGE('',*,*,#3967,.T.);
#5736=ORIENTED_EDGE('',*,*,#4097,.T.);
#5737=ORIENTED_EDGE('',*,*,#4061,.F.);
#5738=ORIENTED_EDGE('',*,*,#3870,.F.);
#5739=ORIENTED_EDGE('',*,*,#4005,.T.);
#5740=ORIENTED_EDGE('',*,*,#3969,.T.);
#5741=ORIENTED_EDGE('',*,*,#4007,.F.);
#5742=ORIENTED_EDGE('',*,*,#4062,.F.);
#5743=ORIENTED_EDGE('',*,*,#4097,.F.);
#5744=ORIENTED_EDGE('',*,*,#3964,.T.);
#5745=ORIENTED_EDGE('',*,*,#4098,.T.);
#5746=ORIENTED_EDGE('',*,*,#4059,.F.);
#5747=ORIENTED_EDGE('',*,*,#3873,.F.);
#5748=ORIENTED_EDGE('',*,*,#4008,.T.);
#5749=ORIENTED_EDGE('',*,*,#3966,.T.);
#5750=ORIENTED_EDGE('',*,*,#4010,.F.);
#5751=ORIENTED_EDGE('',*,*,#4060,.F.);
#5752=ORIENTED_EDGE('',*,*,#4098,.F.);
#5753=ORIENTED_EDGE('',*,*,#3961,.T.);
#5754=ORIENTED_EDGE('',*,*,#4099,.T.);
#5755=ORIENTED_EDGE('',*,*,#4057,.F.);
#5756=ORIENTED_EDGE('',*,*,#3876,.F.);
#5757=ORIENTED_EDGE('',*,*,#4011,.T.);
#5758=ORIENTED_EDGE('',*,*,#3963,.T.);
#5759=ORIENTED_EDGE('',*,*,#4013,.F.);
#5760=ORIENTED_EDGE('',*,*,#4058,.F.);
#5761=ORIENTED_EDGE('',*,*,#4099,.F.);
#5762=ORIENTED_EDGE('',*,*,#3958,.T.);
#5763=ORIENTED_EDGE('',*,*,#4100,.T.);
#5764=ORIENTED_EDGE('',*,*,#4055,.F.);
#5765=ORIENTED_EDGE('',*,*,#3879,.F.);
#5766=ORIENTED_EDGE('',*,*,#4014,.T.);
#5767=ORIENTED_EDGE('',*,*,#3960,.T.);
#5768=ORIENTED_EDGE('',*,*,#4016,.F.);
#5769=ORIENTED_EDGE('',*,*,#4056,.F.);
#5770=ORIENTED_EDGE('',*,*,#4100,.F.);
#5771=ORIENTED_EDGE('',*,*,#3955,.T.);
#5772=ORIENTED_EDGE('',*,*,#4101,.T.);
#5773=ORIENTED_EDGE('',*,*,#4091,.F.);
#5774=ORIENTED_EDGE('',*,*,#3882,.F.);
#5775=ORIENTED_EDGE('',*,*,#4017,.T.);
#5776=ORIENTED_EDGE('',*,*,#3957,.T.);
#5777=ORIENTED_EDGE('',*,*,#4019,.F.);
#5778=ORIENTED_EDGE('',*,*,#4054,.F.);
#5779=ORIENTED_EDGE('',*,*,#4092,.F.);
#5780=ORIENTED_EDGE('',*,*,#4101,.F.);
#5781=ORIENTED_EDGE('',*,*,#3952,.T.);
#5782=ORIENTED_EDGE('',*,*,#4102,.T.);
#5783=ORIENTED_EDGE('',*,*,#4089,.F.);
#5784=ORIENTED_EDGE('',*,*,#3885,.F.);
#5785=ORIENTED_EDGE('',*,*,#4020,.T.);
#5786=ORIENTED_EDGE('',*,*,#3954,.T.);
#5787=ORIENTED_EDGE('',*,*,#4022,.F.);
#5788=ORIENTED_EDGE('',*,*,#4090,.F.);
#5789=ORIENTED_EDGE('',*,*,#4102,.F.);
#5790=ORIENTED_EDGE('',*,*,#3949,.T.);
#5791=ORIENTED_EDGE('',*,*,#4103,.T.);
#5792=ORIENTED_EDGE('',*,*,#4087,.F.);
#5793=ORIENTED_EDGE('',*,*,#3888,.F.);
#5794=ORIENTED_EDGE('',*,*,#4023,.T.);
#5795=ORIENTED_EDGE('',*,*,#3951,.T.);
#5796=ORIENTED_EDGE('',*,*,#4025,.F.);
#5797=ORIENTED_EDGE('',*,*,#4088,.F.);
#5798=ORIENTED_EDGE('',*,*,#4103,.F.);
#5799=ORIENTED_EDGE('',*,*,#3946,.T.);
#5800=ORIENTED_EDGE('',*,*,#4104,.T.);
#5801=ORIENTED_EDGE('',*,*,#4085,.F.);
#5802=ORIENTED_EDGE('',*,*,#3891,.F.);
#5803=ORIENTED_EDGE('',*,*,#4026,.T.);
#5804=ORIENTED_EDGE('',*,*,#3948,.T.);
#5805=ORIENTED_EDGE('',*,*,#4028,.F.);
#5806=ORIENTED_EDGE('',*,*,#4086,.F.);
#5807=ORIENTED_EDGE('',*,*,#4104,.F.);
#5808=ORIENTED_EDGE('',*,*,#3943,.T.);
#5809=ORIENTED_EDGE('',*,*,#4105,.T.);
#5810=ORIENTED_EDGE('',*,*,#4083,.F.);
#5811=ORIENTED_EDGE('',*,*,#3894,.F.);
#5812=ORIENTED_EDGE('',*,*,#4029,.T.);
#5813=ORIENTED_EDGE('',*,*,#3945,.T.);
#5814=ORIENTED_EDGE('',*,*,#4031,.F.);
#5815=ORIENTED_EDGE('',*,*,#4084,.F.);
#5816=ORIENTED_EDGE('',*,*,#4105,.F.);
#5817=ORIENTED_EDGE('',*,*,#3940,.T.);
#5818=ORIENTED_EDGE('',*,*,#4106,.T.);
#5819=ORIENTED_EDGE('',*,*,#4081,.F.);
#5820=ORIENTED_EDGE('',*,*,#3897,.F.);
#5821=ORIENTED_EDGE('',*,*,#4032,.T.);
#5822=ORIENTED_EDGE('',*,*,#3942,.T.);
#5823=ORIENTED_EDGE('',*,*,#4034,.F.);
#5824=ORIENTED_EDGE('',*,*,#4082,.F.);
#5825=ORIENTED_EDGE('',*,*,#4106,.F.);
#5826=ORIENTED_EDGE('',*,*,#3937,.T.);
#5827=ORIENTED_EDGE('',*,*,#4107,.T.);
#5828=ORIENTED_EDGE('',*,*,#4079,.F.);
#5829=ORIENTED_EDGE('',*,*,#3900,.F.);
#5830=ORIENTED_EDGE('',*,*,#4035,.T.);
#5831=ORIENTED_EDGE('',*,*,#3939,.T.);
#5832=ORIENTED_EDGE('',*,*,#4037,.F.);
#5833=ORIENTED_EDGE('',*,*,#4080,.F.);
#5834=ORIENTED_EDGE('',*,*,#4107,.F.);
#5835=ORIENTED_EDGE('',*,*,#3934,.T.);
#5836=ORIENTED_EDGE('',*,*,#4108,.T.);
#5837=ORIENTED_EDGE('',*,*,#4077,.F.);
#5838=ORIENTED_EDGE('',*,*,#3903,.F.);
#5839=ORIENTED_EDGE('',*,*,#4038,.T.);
#5840=ORIENTED_EDGE('',*,*,#3936,.T.);
#5841=ORIENTED_EDGE('',*,*,#4040,.F.);
#5842=ORIENTED_EDGE('',*,*,#4078,.F.);
#5843=ORIENTED_EDGE('',*,*,#4108,.F.);
#5844=ORIENTED_EDGE('',*,*,#3931,.T.);
#5845=ORIENTED_EDGE('',*,*,#4109,.T.);
#5846=ORIENTED_EDGE('',*,*,#4075,.F.);
#5847=ORIENTED_EDGE('',*,*,#3906,.F.);
#5848=ORIENTED_EDGE('',*,*,#4041,.T.);
#5849=ORIENTED_EDGE('',*,*,#3933,.T.);
#5850=ORIENTED_EDGE('',*,*,#4043,.F.);
#5851=ORIENTED_EDGE('',*,*,#4076,.F.);
#5852=ORIENTED_EDGE('',*,*,#4109,.F.);
#5853=ORIENTED_EDGE('',*,*,#3928,.T.);
#5854=ORIENTED_EDGE('',*,*,#4110,.T.);
#5855=ORIENTED_EDGE('',*,*,#4073,.F.);
#5856=ORIENTED_EDGE('',*,*,#3909,.F.);
#5857=ORIENTED_EDGE('',*,*,#4044,.T.);
#5858=ORIENTED_EDGE('',*,*,#3930,.T.);
#5859=ORIENTED_EDGE('',*,*,#4046,.F.);
#5860=ORIENTED_EDGE('',*,*,#4074,.F.);
#5861=ORIENTED_EDGE('',*,*,#4110,.F.);
#5862=ORIENTED_EDGE('',*,*,#3925,.T.);
#5863=ORIENTED_EDGE('',*,*,#4111,.T.);
#5864=ORIENTED_EDGE('',*,*,#4071,.F.);
#5865=ORIENTED_EDGE('',*,*,#3912,.F.);
#5866=ORIENTED_EDGE('',*,*,#4047,.T.);
#5867=ORIENTED_EDGE('',*,*,#3927,.T.);
#5868=ORIENTED_EDGE('',*,*,#4049,.F.);
#5869=ORIENTED_EDGE('',*,*,#4072,.F.);
#5870=ORIENTED_EDGE('',*,*,#4111,.F.);
#5871=ORIENTED_EDGE('',*,*,#3986,.T.);
#5872=ORIENTED_EDGE('',*,*,#3924,.F.);
#6594=CYLINDRICAL_SURFACE('',#7415,2.05);
#6595=CYLINDRICAL_SURFACE('',#7418,2.05);
#6596=CYLINDRICAL_SURFACE('',#7423,6.025);
#6597=CYLINDRICAL_SURFACE('',#7454,10.);
#6598=CYLINDRICAL_SURFACE('',#7497,10.5);
#6796=ADVANCED_FACE('',(#1145),#708,.F.);
#6797=ADVANCED_FACE('',(#1146),#6594,.F.);
#6798=ADVANCED_FACE('',(#1147),#709,.F.);
#6799=ADVANCED_FACE('',(#1148),#6595,.F.);
#6800=ADVANCED_FACE('',(#1149),#710,.F.);
#6801=ADVANCED_FACE('',(#1150,#803),#6596,.F.);
#6802=ADVANCED_FACE('',(#1151,#804),#909,.T.);
#6803=ADVANCED_FACE('',(#1152),#711,.F.);
#6804=ADVANCED_FACE('',(#1153,#805),#910,.T.);
#6805=ADVANCED_FACE('',(#1154),#712,.T.);
#6806=ADVANCED_FACE('',(#1155,#806),#6597,.T.);
#6807=ADVANCED_FACE('',(#1156),#713,.T.);
#6808=ADVANCED_FACE('',(#1157),#714,.T.);
#6809=ADVANCED_FACE('',(#1158),#715,.T.);
#6810=ADVANCED_FACE('',(#1159),#716,.T.);
#6811=ADVANCED_FACE('',(#1160),#717,.T.);
#6812=ADVANCED_FACE('',(#1161),#718,.T.);
#6813=ADVANCED_FACE('',(#1162),#719,.T.);
#6814=ADVANCED_FACE('',(#1163),#720,.T.);
#6815=ADVANCED_FACE('',(#1164),#721,.T.);
#6816=ADVANCED_FACE('',(#1165),#722,.T.);
#6817=ADVANCED_FACE('',(#1166),#723,.T.);
#6818=ADVANCED_FACE('',(#1167),#724,.T.);
#6819=ADVANCED_FACE('',(#1168),#725,.T.);
#6820=ADVANCED_FACE('',(#1169),#726,.T.);
#6821=ADVANCED_FACE('',(#1170),#727,.T.);
#6822=ADVANCED_FACE('',(#1171),#728,.T.);
#6823=ADVANCED_FACE('',(#1172),#729,.T.);
#6824=ADVANCED_FACE('',(#1173),#730,.T.);
#6825=ADVANCED_FACE('',(#1174),#731,.T.);
#6826=ADVANCED_FACE('',(#1175),#732,.T.);
#6827=ADVANCED_FACE('',(#1176),#6598,.T.);
#6828=ADVANCED_FACE('',(#1177),#733,.T.);
#6829=ADVANCED_FACE('',(#1178),#133,.F.);
#6830=ADVANCED_FACE('',(#1179),#134,.F.);
#6831=ADVANCED_FACE('',(#1180),#135,.F.);
#6832=ADVANCED_FACE('',(#1181),#136,.F.);
#6833=ADVANCED_FACE('',(#1182),#137,.F.);
#6834=ADVANCED_FACE('',(#1183),#138,.F.);
#6835=ADVANCED_FACE('',(#1184),#139,.F.);
#6836=ADVANCED_FACE('',(#1185),#140,.F.);
#6837=ADVANCED_FACE('',(#1186),#141,.F.);
#6838=ADVANCED_FACE('',(#1187),#142,.F.);
#6839=ADVANCED_FACE('',(#1188),#143,.F.);
#6840=ADVANCED_FACE('',(#1189),#144,.F.);
#6841=ADVANCED_FACE('',(#1190),#145,.F.);
#6842=ADVANCED_FACE('',(#1191),#146,.F.);
#6843=ADVANCED_FACE('',(#1192),#147,.F.);
#6844=ADVANCED_FACE('',(#1193),#148,.F.);
#6845=ADVANCED_FACE('',(#1194),#149,.F.);
#6846=ADVANCED_FACE('',(#1195),#150,.F.);
#6847=ADVANCED_FACE('',(#1196),#151,.F.);
#6848=ADVANCED_FACE('',(#1197),#152,.F.);
#6849=ADVANCED_FACE('',(#1198),#153,.F.);
#6850=ADVANCED_FACE('',(#1199),#911,.T.);
#6851=ADVANCED_FACE('',(#1200),#734,.T.);
#6852=ADVANCED_FACE('',(#1201),#154,.F.);
#6853=ADVANCED_FACE('',(#1202),#912,.T.);
#6854=ADVANCED_FACE('',(#1203),#155,.F.);
#6855=ADVANCED_FACE('',(#1204),#913,.T.);
#6856=ADVANCED_FACE('',(#1205),#156,.F.);
#6857=ADVANCED_FACE('',(#1206),#914,.T.);
#6858=ADVANCED_FACE('',(#1207),#157,.F.);
#6859=ADVANCED_FACE('',(#1208),#915,.T.);
#6860=ADVANCED_FACE('',(#1209),#158,.F.);
#6861=ADVANCED_FACE('',(#1210),#916,.T.);
#6862=ADVANCED_FACE('',(#1211),#159,.F.);
#6863=ADVANCED_FACE('',(#1212),#917,.T.);
#6864=ADVANCED_FACE('',(#1213),#160,.F.);
#6865=ADVANCED_FACE('',(#1214),#918,.T.);
#6866=ADVANCED_FACE('',(#1215),#161,.F.);
#6867=ADVANCED_FACE('',(#1216),#919,.T.);
#6868=ADVANCED_FACE('',(#1217),#162,.F.);
#6869=ADVANCED_FACE('',(#1218),#920,.T.);
#6870=ADVANCED_FACE('',(#1219),#163,.F.);
#6871=ADVANCED_FACE('',(#1220),#921,.T.);
#6872=ADVANCED_FACE('',(#1221),#164,.F.);
#6873=ADVANCED_FACE('',(#1222),#922,.T.);
#6874=ADVANCED_FACE('',(#1223),#165,.F.);
#6875=ADVANCED_FACE('',(#1224),#923,.T.);
#6876=ADVANCED_FACE('',(#1225),#166,.F.);
#6877=ADVANCED_FACE('',(#1226),#924,.T.);
#6878=ADVANCED_FACE('',(#1227),#167,.F.);
#6879=ADVANCED_FACE('',(#1228),#925,.T.);
#6880=ADVANCED_FACE('',(#1229),#168,.F.);
#6881=ADVANCED_FACE('',(#1230),#926,.T.);
#6882=ADVANCED_FACE('',(#1231),#169,.F.);
#6883=ADVANCED_FACE('',(#1232),#927,.T.);
#6884=ADVANCED_FACE('',(#1233),#170,.F.);
#6885=ADVANCED_FACE('',(#1234),#928,.T.);
#6886=ADVANCED_FACE('',(#1235),#171,.F.);
#6887=ADVANCED_FACE('',(#1236),#929,.T.);
#6888=ADVANCED_FACE('',(#1237),#172,.F.);
#6889=ADVANCED_FACE('',(#1238),#930,.T.);
#6890=ADVANCED_FACE('',(#1239,#807),#931,.T.);
#7027=CLOSED_SHELL('',(#6796,#6797,#6798,#6799,#6800,#6801,#6802,#6803,
#6804,#6805,#6806,#6807,#6808,#6809,#6810,#6811,#6812,#6813,#6814,#6815,
#6816,#6817,#6818,#6819,#6820,#6821,#6822,#6823,#6824,#6825,#6826,#6827,
#6828,#6829,#6830,#6831,#6832,#6833,#6834,#6835,#6836,#6837,#6838,#6839,
#6840,#6841,#6842,#6843,#6844,#6845,#6846,#6847,#6848,#6849,#6850,#6851,
#6852,#6853,#6854,#6855,#6856,#6857,#6858,#6859,#6860,#6861,#6862,#6863,
#6864,#6865,#6866,#6867,#6868,#6869,#6870,#6871,#6872,#6873,#6874,#6875,
#6876,#6877,#6878,#6879,#6880,#6881,#6882,#6883,#6884,#6885,#6886,#6887,
#6888,#6889,#6890));
#7412=AXIS2_PLACEMENT_3D('',#15842,#8481,#8482);
#7413=AXIS2_PLACEMENT_3D('',#15843,#8483,#8484);
#7414=AXIS2_PLACEMENT_3D('',#15888,#8486,#8487);
#7415=AXIS2_PLACEMENT_3D('',#15889,#8488,#8489);
#7416=AXIS2_PLACEMENT_3D('',#15932,#8491,#8492);
#7417=AXIS2_PLACEMENT_3D('',#15955,#8494,#8495);
#7418=AXIS2_PLACEMENT_3D('',#15975,#8496,#8497);
#7419=AXIS2_PLACEMENT_3D('',#16015,#8499,#8500);
#7420=AXIS2_PLACEMENT_3D('',#16017,#8501,#8502);
#7421=AXIS2_PLACEMENT_3D('',#16021,#8504,#8505);
#7422=AXIS2_PLACEMENT_3D('',#16022,#8506,#8507);
#7423=AXIS2_PLACEMENT_3D('',#16023,#8508,#8509);
#7424=AXIS2_PLACEMENT_3D('',#16026,#8510,#8511);
#7425=AXIS2_PLACEMENT_3D('',#16027,#8512,#8513);
#7426=AXIS2_PLACEMENT_3D('',#16030,#8516,#8517);
#7427=AXIS2_PLACEMENT_3D('',#16033,#8518,#8519);
#7428=AXIS2_PLACEMENT_3D('',#16107,#8520,#8521);
#7429=AXIS2_PLACEMENT_3D('',#16181,#8522,#8523);
#7430=AXIS2_PLACEMENT_3D('',#16255,#8524,#8525);
#7431=AXIS2_PLACEMENT_3D('',#16329,#8526,#8527);
#7432=AXIS2_PLACEMENT_3D('',#16403,#8528,#8529);
#7433=AXIS2_PLACEMENT_3D('',#16477,#8530,#8531);
#7434=AXIS2_PLACEMENT_3D('',#16551,#8532,#8533);
#7435=AXIS2_PLACEMENT_3D('',#16625,#8534,#8535);
#7436=AXIS2_PLACEMENT_3D('',#16699,#8536,#8537);
#7437=AXIS2_PLACEMENT_3D('',#16773,#8538,#8539);
#7438=AXIS2_PLACEMENT_3D('',#16847,#8540,#8541);
#7439=AXIS2_PLACEMENT_3D('',#16921,#8542,#8543);
#7440=AXIS2_PLACEMENT_3D('',#16995,#8544,#8545);
#7441=AXIS2_PLACEMENT_3D('',#17069,#8546,#8547);
#7442=AXIS2_PLACEMENT_3D('',#17143,#8548,#8549);
#7443=AXIS2_PLACEMENT_3D('',#17217,#8550,#8551);
#7444=AXIS2_PLACEMENT_3D('',#17291,#8552,#8553);
#7445=AXIS2_PLACEMENT_3D('',#17365,#8554,#8555);
#7446=AXIS2_PLACEMENT_3D('',#17439,#8556,#8557);
#7447=AXIS2_PLACEMENT_3D('',#17511,#8558,#8559);
#7448=AXIS2_PLACEMENT_3D('',#17514,#8561,#8562);
#7449=AXIS2_PLACEMENT_3D('',#17515,#8563,#8564);
#7450=AXIS2_PLACEMENT_3D('',#17517,#8565,#8566);
#7451=AXIS2_PLACEMENT_3D('',#17518,#8567,#8568);
#7452=AXIS2_PLACEMENT_3D('',#17522,#8570,#8571);
#7453=AXIS2_PLACEMENT_3D('',#17523,#8572,#8573);
#7454=AXIS2_PLACEMENT_3D('',#17524,#8574,#8575);
#7455=AXIS2_PLACEMENT_3D('',#17528,#8578,#8579);
#7456=AXIS2_PLACEMENT_3D('',#17529,#8580,#8581);
#7457=AXIS2_PLACEMENT_3D('',#17557,#8582,#8583);
#7458=AXIS2_PLACEMENT_3D('',#17558,#8584,#8585);
#7459=AXIS2_PLACEMENT_3D('',#17586,#8586,#8587);
#7460=AXIS2_PLACEMENT_3D('',#17587,#8588,#8589);
#7461=AXIS2_PLACEMENT_3D('',#17615,#8590,#8591);
#7462=AXIS2_PLACEMENT_3D('',#17616,#8592,#8593);
#7463=AXIS2_PLACEMENT_3D('',#17644,#8594,#8595);
#7464=AXIS2_PLACEMENT_3D('',#17645,#8596,#8597);
#7465=AXIS2_PLACEMENT_3D('',#17673,#8598,#8599);
#7466=AXIS2_PLACEMENT_3D('',#17674,#8600,#8601);
#7467=AXIS2_PLACEMENT_3D('',#17702,#8602,#8603);
#7468=AXIS2_PLACEMENT_3D('',#17703,#8604,#8605);
#7469=AXIS2_PLACEMENT_3D('',#17731,#8606,#8607);
#7470=AXIS2_PLACEMENT_3D('',#17732,#8608,#8609);
#7471=AXIS2_PLACEMENT_3D('',#17760,#8610,#8611);
#7472=AXIS2_PLACEMENT_3D('',#17761,#8612,#8613);
#7473=AXIS2_PLACEMENT_3D('',#17789,#8614,#8615);
#7474=AXIS2_PLACEMENT_3D('',#17790,#8616,#8617);
#7475=AXIS2_PLACEMENT_3D('',#17818,#8618,#8619);
#7476=AXIS2_PLACEMENT_3D('',#17819,#8620,#8621);
#7477=AXIS2_PLACEMENT_3D('',#17847,#8622,#8623);
#7478=AXIS2_PLACEMENT_3D('',#17848,#8624,#8625);
#7479=AXIS2_PLACEMENT_3D('',#17876,#8626,#8627);
#7480=AXIS2_PLACEMENT_3D('',#17877,#8628,#8629);
#7481=AXIS2_PLACEMENT_3D('',#17905,#8630,#8631);
#7482=AXIS2_PLACEMENT_3D('',#17906,#8632,#8633);
#7483=AXIS2_PLACEMENT_3D('',#17934,#8634,#8635);
#7484=AXIS2_PLACEMENT_3D('',#17935,#8636,#8637);
#7485=AXIS2_PLACEMENT_3D('',#17963,#8638,#8639);
#7486=AXIS2_PLACEMENT_3D('',#17964,#8640,#8641);
#7487=AXIS2_PLACEMENT_3D('',#17992,#8642,#8643);
#7488=AXIS2_PLACEMENT_3D('',#17993,#8644,#8645);
#7489=AXIS2_PLACEMENT_3D('',#18021,#8646,#8647);
#7490=AXIS2_PLACEMENT_3D('',#18022,#8648,#8649);
#7491=AXIS2_PLACEMENT_3D('',#18050,#8650,#8651);
#7492=AXIS2_PLACEMENT_3D('',#18051,#8652,#8653);
#7493=AXIS2_PLACEMENT_3D('',#18079,#8654,#8655);
#7494=AXIS2_PLACEMENT_3D('',#18080,#8656,#8657);
#7495=AXIS2_PLACEMENT_3D('',#18082,#8658,#8659);
#7496=AXIS2_PLACEMENT_3D('',#18085,#8661,#8662);
#7497=AXIS2_PLACEMENT_3D('',#18086,#8663,#8664);
#7498=AXIS2_PLACEMENT_3D('',#18089,#8666,#8667);
#7499=AXIS2_PLACEMENT_3D('',#18090,#8668,#8669);
#7500=AXIS2_PLACEMENT_3D('',#18118,#8670,#8671);
#7501=AXIS2_PLACEMENT_3D('',#19398,#8692,#8693);
#7502=AXIS2_PLACEMENT_3D('',#19399,#8694,#8695);
#7503=AXIS2_PLACEMENT_3D('',#19400,#8696,#8697);
#7504=AXIS2_PLACEMENT_3D('',#19403,#8699,#8700);
#7505=AXIS2_PLACEMENT_3D('',#19433,#8701,#8702);
#7506=AXIS2_PLACEMENT_3D('',#19463,#8703,#8704);
#7507=AXIS2_PLACEMENT_3D('',#19493,#8705,#8706);
#7508=AXIS2_PLACEMENT_3D('',#19523,#8707,#8708);
#7509=AXIS2_PLACEMENT_3D('',#19553,#8709,#8710);
#7510=AXIS2_PLACEMENT_3D('',#19583,#8711,#8712);
#7511=AXIS2_PLACEMENT_3D('',#19613,#8713,#8714);
#7512=AXIS2_PLACEMENT_3D('',#19643,#8715,#8716);
#7513=AXIS2_PLACEMENT_3D('',#19673,#8717,#8718);
#7514=AXIS2_PLACEMENT_3D('',#19703,#8719,#8720);
#7515=AXIS2_PLACEMENT_3D('',#19733,#8721,#8722);
#7516=AXIS2_PLACEMENT_3D('',#19763,#8723,#8724);
#7517=AXIS2_PLACEMENT_3D('',#19793,#8725,#8726);
#7518=AXIS2_PLACEMENT_3D('',#19823,#8727,#8728);
#7519=AXIS2_PLACEMENT_3D('',#19853,#8729,#8730);
#7520=AXIS2_PLACEMENT_3D('',#19883,#8731,#8732);
#7521=AXIS2_PLACEMENT_3D('',#19913,#8733,#8734);
#7522=AXIS2_PLACEMENT_3D('',#19943,#8735,#8736);
#7523=AXIS2_PLACEMENT_3D('',#19973,#8737,#8738);
#7524=AXIS2_PLACEMENT_3D('',#20024,#8739,#8740);
#7525=AXIS2_PLACEMENT_3D('',#20079,#8741,#8742);
#7526=AXIS2_PLACEMENT_3D('',#20134,#8743,#8744);
#7527=AXIS2_PLACEMENT_3D('',#20185,#8745,#8746);
#7528=AXIS2_PLACEMENT_3D('',#20236,#8747,#8748);
#7529=AXIS2_PLACEMENT_3D('',#20287,#8749,#8750);
#7530=AXIS2_PLACEMENT_3D('',#20342,#8751,#8752);
#7531=AXIS2_PLACEMENT_3D('',#20397,#8753,#8754);
#7532=AXIS2_PLACEMENT_3D('',#20448,#8755,#8756);
#7533=AXIS2_PLACEMENT_3D('',#20499,#8757,#8758);
#7534=AXIS2_PLACEMENT_3D('',#20550,#8759,#8760);
#7535=AXIS2_PLACEMENT_3D('',#20605,#8761,#8762);
#7536=AXIS2_PLACEMENT_3D('',#20660,#8763,#8764);
#7537=AXIS2_PLACEMENT_3D('',#20711,#8765,#8766);
#7538=AXIS2_PLACEMENT_3D('',#20762,#8767,#8768);
#7539=AXIS2_PLACEMENT_3D('',#20813,#8769,#8770);
#7540=AXIS2_PLACEMENT_3D('',#20868,#8771,#8772);
#7541=AXIS2_PLACEMENT_3D('',#20923,#8773,#8774);
#7542=AXIS2_PLACEMENT_3D('',#20974,#8775,#8776);
#7543=AXIS2_PLACEMENT_3D('',#20975,#8777,#8778);
#8481=DIRECTION('axis',(0.,0.,1.));
#8482=DIRECTION('refdir',(1.,0.,0.));
#8483=DIRECTION('center_axis',(0.,-1.,0.));
#8484=DIRECTION('ref_axis',(0.,0.,-1.));
#8485=DIRECTION('',(-8.65956056235493E-17,0.707106781186548,-0.707106781186547));
#8486=DIRECTION('center_axis',(0.,1.,0.));
#8487=DIRECTION('ref_axis',(0.,0.,-1.));
#8488=DIRECTION('center_axis',(0.,1.,0.));
#8489=DIRECTION('ref_axis',(0.,0.,-1.));
#8490=DIRECTION('',(0.,1.,0.));
#8491=DIRECTION('center_axis',(0.,0.,1.));
#8492=DIRECTION('ref_axis',(1.,0.,0.));
#8493=DIRECTION('',(0.707106781186547,-8.65956056235493E-17,-0.707106781186548));
#8494=DIRECTION('center_axis',(0.,0.,-1.));
#8495=DIRECTION('ref_axis',(1.,0.,0.));
#8496=DIRECTION('center_axis',(0.,0.,-1.));
#8497=DIRECTION('ref_axis',(1.,0.,0.));
#8498=DIRECTION('',(0.,0.,-1.));
#8499=DIRECTION('center_axis',(-1.,0.,0.));
#8500=DIRECTION('ref_axis',(0.,-1.,0.));
#8501=DIRECTION('center_axis',(-1.,0.,0.));
#8502=DIRECTION('ref_axis',(0.,-1.,0.));
#8503=DIRECTION('',(0.707106781186547,-0.707106781186547,8.65956056235493E-17));
#8504=DIRECTION('center_axis',(1.,0.,0.));
#8505=DIRECTION('ref_axis',(0.,-1.,0.));
#8506=DIRECTION('center_axis',(1.,0.,0.));
#8507=DIRECTION('ref_axis',(0.,-1.,0.));
#8508=DIRECTION('center_axis',(1.,0.,0.));
#8509=DIRECTION('ref_axis',(0.,1.,0.));
#8510=DIRECTION('center_axis',(-1.,0.,0.));
#8511=DIRECTION('ref_axis',(0.,-1.,0.));
#8512=DIRECTION('center_axis',(-1.,0.,0.));
#8513=DIRECTION('ref_axis',(0.,-1.,0.));
#8514=DIRECTION('',(-1.,0.,0.));
#8515=DIRECTION('',(-1.,0.,0.));
#8516=DIRECTION('center_axis',(-1.,0.,0.));
#8517=DIRECTION('ref_axis',(0.,0.,1.));
#8518=DIRECTION('center_axis',(1.,0.,0.));
#8519=DIRECTION('ref_axis',(0.,0.,-1.));
#8520=DIRECTION('center_axis',(1.,0.,0.));
#8521=DIRECTION('ref_axis',(0.,0.,-1.));
#8522=DIRECTION('center_axis',(1.,0.,0.));
#8523=DIRECTION('ref_axis',(0.,0.,-1.));
#8524=DIRECTION('center_axis',(1.,0.,0.));
#8525=DIRECTION('ref_axis',(0.,0.,-1.));
#8526=DIRECTION('center_axis',(1.,0.,0.));
#8527=DIRECTION('ref_axis',(0.,0.,-1.));
#8528=DIRECTION('center_axis',(1.,0.,0.));
#8529=DIRECTION('ref_axis',(0.,0.,-1.));
#8530=DIRECTION('center_axis',(1.,0.,0.));
#8531=DIRECTION('ref_axis',(0.,0.,-1.));
#8532=DIRECTION('center_axis',(1.,0.,0.));
#8533=DIRECTION('ref_axis',(0.,0.,-1.));
#8534=DIRECTION('center_axis',(1.,0.,0.));
#8535=DIRECTION('ref_axis',(0.,0.,-1.));
#8536=DIRECTION('center_axis',(1.,0.,0.));
#8537=DIRECTION('ref_axis',(0.,0.,-1.));
#8538=DIRECTION('center_axis',(1.,0.,0.));
#8539=DIRECTION('ref_axis',(0.,0.,-1.));
#8540=DIRECTION('center_axis',(1.,0.,0.));
#8541=DIRECTION('ref_axis',(0.,0.,-1.));
#8542=DIRECTION('center_axis',(1.,0.,0.));
#8543=DIRECTION('ref_axis',(0.,0.,-1.));
#8544=DIRECTION('center_axis',(1.,0.,0.));
#8545=DIRECTION('ref_axis',(0.,0.,-1.));
#8546=DIRECTION('center_axis',(1.,0.,0.));
#8547=DIRECTION('ref_axis',(0.,0.,-1.));
#8548=DIRECTION('center_axis',(1.,0.,0.));
#8549=DIRECTION('ref_axis',(0.,0.,-1.));
#8550=DIRECTION('center_axis',(1.,0.,0.));
#8551=DIRECTION('ref_axis',(0.,0.,-1.));
#8552=DIRECTION('center_axis',(1.,0.,0.));
#8553=DIRECTION('ref_axis',(0.,0.,-1.));
#8554=DIRECTION('center_axis',(1.,0.,0.));
#8555=DIRECTION('ref_axis',(0.,0.,-1.));
#8556=DIRECTION('center_axis',(1.,0.,0.));
#8557=DIRECTION('ref_axis',(0.,0.,-1.));
#8558=DIRECTION('center_axis',(1.,0.,0.));
#8559=DIRECTION('ref_axis',(0.,-1.,0.));
#8560=DIRECTION('',(0.707106781186546,0.707106781186549,-8.65956056235495E-17));
#8561=DIRECTION('center_axis',(1.,0.,0.));
#8562=DIRECTION('ref_axis',(0.,-1.,0.));
#8563=DIRECTION('center_axis',(1.,0.,0.));
#8564=DIRECTION('ref_axis',(0.,0.,-1.));
#8565=DIRECTION('center_axis',(-1.,0.,0.));
#8566=DIRECTION('ref_axis',(0.,-1.,0.));
#8567=DIRECTION('center_axis',(-1.,0.,0.));
#8568=DIRECTION('ref_axis',(0.,-1.,0.));
#8569=DIRECTION('',(-0.707106781186546,0.707106781186549,8.65956056235495E-17));
#8570=DIRECTION('center_axis',(1.,0.,0.));
#8571=DIRECTION('ref_axis',(0.,-1.,0.));
#8572=DIRECTION('center_axis',(1.,0.,0.));
#8573=DIRECTION('ref_axis',(0.,-1.,0.));
#8574=DIRECTION('center_axis',(1.,0.,0.));
#8575=DIRECTION('ref_axis',(0.,1.,0.));
#8576=DIRECTION('',(-1.,0.,0.));
#8577=DIRECTION('',(-1.,0.,0.));
#8578=DIRECTION('center_axis',(1.,0.,0.));
#8579=DIRECTION('ref_axis',(0.,0.,-1.));
#8580=DIRECTION('center_axis',(-1.,0.,0.));
#8581=DIRECTION('ref_axis',(0.,1.,0.));
#8582=DIRECTION('center_axis',(1.,-9.89384015765324E-17,1.11713723763385E-17));
#8583=DIRECTION('ref_axis',(0.,1.,0.));
#8584=DIRECTION('center_axis',(-1.,0.,0.));
#8585=DIRECTION('ref_axis',(0.,1.,0.));
#8586=DIRECTION('center_axis',(1.,-9.75481554459673E-17,-1.99490409889652E-17));
#8587=DIRECTION('ref_axis',(0.,1.,0.));
#8588=DIRECTION('center_axis',(-1.,0.,0.));
#8589=DIRECTION('ref_axis',(0.,1.,0.));
#8590=DIRECTION('center_axis',(1.,-8.66092162023871E-17,-4.91167032291274E-17));
#8591=DIRECTION('ref_axis',(0.,1.,0.));
#8592=DIRECTION('center_axis',(-1.,0.,0.));
#8593=DIRECTION('ref_axis',(0.,1.,0.));
#8594=DIRECTION('center_axis',(1.,-6.71923634350248E-17,-7.34764803410285E-17));
#8595=DIRECTION('ref_axis',(0.,1.,0.));
#8596=DIRECTION('center_axis',(-1.,0.,0.));
#8597=DIRECTION('ref_axis',(0.,1.,0.));
#8598=DIRECTION('center_axis',(1.,-4.1198253977918E-17,-9.06438676164084E-17));
#8599=DIRECTION('ref_axis',(0.,1.,0.));
#8600=DIRECTION('center_axis',(-1.,0.,0.));
#8601=DIRECTION('ref_axis',(0.,1.,0.));
#8602=DIRECTION('center_axis',(1.,-1.11713723763385E-17,-9.89384015765324E-17));
#8603=DIRECTION('ref_axis',(0.,1.,0.));
#8604=DIRECTION('center_axis',(-1.,0.,0.));
#8605=DIRECTION('ref_axis',(0.,1.,0.));
#8606=DIRECTION('center_axis',(1.,1.99490409889652E-17,-9.75481554459673E-17));
#8607=DIRECTION('ref_axis',(0.,1.,0.));
#8608=DIRECTION('center_axis',(-1.,0.,0.));
#8609=DIRECTION('ref_axis',(0.,1.,0.));
#8610=DIRECTION('center_axis',(1.,4.91167032291274E-17,-8.66092162023871E-17));
#8611=DIRECTION('ref_axis',(0.,1.,0.));
#8612=DIRECTION('center_axis',(-1.,0.,0.));
#8613=DIRECTION('ref_axis',(0.,1.,0.));
#8614=DIRECTION('center_axis',(1.,7.34764803410285E-17,-6.71923634350248E-17));
#8615=DIRECTION('ref_axis',(0.,1.,0.));
#8616=DIRECTION('center_axis',(-1.,0.,0.));
#8617=DIRECTION('ref_axis',(0.,1.,0.));
#8618=DIRECTION('center_axis',(1.,9.06438676164084E-17,-4.1198253977918E-17));
#8619=DIRECTION('ref_axis',(0.,1.,0.));
#8620=DIRECTION('center_axis',(-1.,0.,0.));
#8621=DIRECTION('ref_axis',(0.,-0.996349796141496,0.0853644172287271));
#8622=DIRECTION('center_axis',(1.,9.89384015765324E-17,-1.11713723763385E-17));
#8623=DIRECTION('ref_axis',(0.,1.,0.));
#8624=DIRECTION('center_axis',(-1.,0.,0.));
#8625=DIRECTION('ref_axis',(0.,1.,0.));
#8626=DIRECTION('center_axis',(1.,9.75481554459673E-17,1.99490409889651E-17));
#8627=DIRECTION('ref_axis',(0.,1.,0.));
#8628=DIRECTION('center_axis',(-1.,0.,0.));
#8629=DIRECTION('ref_axis',(0.,1.,0.));
#8630=DIRECTION('center_axis',(1.,8.66092162023871E-17,4.91167032291274E-17));
#8631=DIRECTION('ref_axis',(0.,1.,0.));
#8632=DIRECTION('center_axis',(-1.,0.,0.));
#8633=DIRECTION('ref_axis',(0.,1.,0.));
#8634=DIRECTION('center_axis',(1.,6.71923634350248E-17,7.34764803410285E-17));
#8635=DIRECTION('ref_axis',(0.,1.,0.));
#8636=DIRECTION('center_axis',(-1.,0.,0.));
#8637=DIRECTION('ref_axis',(0.,1.,0.));
#8638=DIRECTION('center_axis',(1.,4.1198253977918E-17,9.06438676164084E-17));
#8639=DIRECTION('ref_axis',(0.,1.,0.));
#8640=DIRECTION('center_axis',(-1.,0.,0.));
#8641=DIRECTION('ref_axis',(0.,1.,0.));
#8642=DIRECTION('center_axis',(1.,1.11713723763385E-17,9.89384015765324E-17));
#8643=DIRECTION('ref_axis',(0.,1.,0.));
#8644=DIRECTION('center_axis',(-1.,0.,0.));
#8645=DIRECTION('ref_axis',(0.,1.,0.));
#8646=DIRECTION('center_axis',(1.,-1.99490409889651E-17,9.75481554459673E-17));
#8647=DIRECTION('ref_axis',(0.,1.,0.));
#8648=DIRECTION('center_axis',(-1.,0.,0.));
#8649=DIRECTION('ref_axis',(0.,1.,0.));
#8650=DIRECTION('center_axis',(1.,-4.91167032291274E-17,8.66092162023871E-17));
#8651=DIRECTION('ref_axis',(0.,1.,0.));
#8652=DIRECTION('center_axis',(-1.,0.,0.));
#8653=DIRECTION('ref_axis',(0.,1.,0.));
#8654=DIRECTION('center_axis',(1.,-7.34764803410285E-17,6.71923634350248E-17));
#8655=DIRECTION('ref_axis',(0.,1.,0.));
#8656=DIRECTION('center_axis',(-1.,0.,0.));
#8657=DIRECTION('ref_axis',(0.,1.,0.));
#8658=DIRECTION('center_axis',(-1.,0.,0.));
#8659=DIRECTION('ref_axis',(0.,1.,0.));
#8660=DIRECTION('',(0.68394112888133,0.729537204140085,8.93425401909064E-17));
#8661=DIRECTION('center_axis',(1.,0.,0.));
#8662=DIRECTION('ref_axis',(0.,0.,-1.));
#8663=DIRECTION('center_axis',(1.,0.,0.));
#8664=DIRECTION('ref_axis',(0.,1.,0.));
#8665=DIRECTION('',(1.,0.,0.));
#8666=DIRECTION('center_axis',(1.,0.,0.));
#8667=DIRECTION('ref_axis',(0.,1.,0.));
#8668=DIRECTION('center_axis',(-1.,0.,0.));
#8669=DIRECTION('ref_axis',(0.,1.,0.));
#8670=DIRECTION('center_axis',(1.,-9.06438676164084E-17,4.11982539779181E-17));
#8671=DIRECTION('ref_axis',(0.,1.,0.));
#8672=DIRECTION('',(0.657420344909251,0.594324098593915,-0.46322495175663));
#8673=DIRECTION('',(0.657420344909251,0.422091424447672,-0.624209355510742));
#8674=DIRECTION('',(0.657420344909251,0.20854150079261,-0.724091798425149));
#8675=DIRECTION('',(0.657420344909251,-0.0254219179541074,-0.753095091065488));
#8676=DIRECTION('',(0.657420344909251,-0.256896862246559,-0.7083801890703));
#8677=DIRECTION('',(0.657420344909251,-0.463224951756629,-0.594324098593915));
#8678=DIRECTION('',(0.657420344909251,-0.624209355510742,-0.422091424447672));
#8679=DIRECTION('',(0.657420344909251,-0.724091798425149,-0.20854150079261));
#8680=DIRECTION('',(0.657420344909251,-0.753095091065488,0.0254219179541074));
#8681=DIRECTION('',(0.657420344909251,-0.7083801890703,0.256896862246559));
#8682=DIRECTION('',(0.657420344909251,-0.594324098593915,0.463224951756629));
#8683=DIRECTION('',(0.657420344909251,-0.422091424447672,0.624209355510742));
#8684=DIRECTION('',(0.657420344909251,-0.20854150079261,0.724091798425149));
#8685=DIRECTION('',(0.657420344909251,0.0254219179541074,0.753095091065488));
#8686=DIRECTION('',(0.657420344909251,0.256896862246559,0.7083801890703));
#8687=DIRECTION('',(0.657420344909251,0.463224951756629,0.594324098593915));
#8688=DIRECTION('',(0.657420344909251,0.624209355510742,0.422091424447673));
#8689=DIRECTION('',(0.657420344909251,0.724091798425149,0.20854150079261));
#8690=DIRECTION('',(0.657420344909251,0.753095091065488,-0.0254219179541073));
#8691=DIRECTION('',(0.657420344909251,0.7083801890703,-0.256896862246559));
#8692=DIRECTION('center_axis',(1.,-9.06438676164084E-17,4.11982539779181E-17));
#8693=DIRECTION('ref_axis',(1.11713723763385E-17,-0.309016994374948,-0.951056516295153));
#8694=DIRECTION('center_axis',(1.,-9.06438676164084E-17,4.11982539779181E-17));
#8695=DIRECTION('ref_axis',(0.,1.,0.));
#8696=DIRECTION('center_axis',(1.,0.,0.));
#8697=DIRECTION('ref_axis',(0.,1.,0.));
#8698=DIRECTION('',(-0.739012155113086,0.673692091830617,8.2503486387125E-17));
#8699=DIRECTION('center_axis',(1.,9.89384015765324E-17,-1.11713723763385E-17));
#8700=DIRECTION('ref_axis',(0.,1.,0.));
#8701=DIRECTION('center_axis',(1.,9.75481554459673E-17,1.99490409889651E-17));
#8702=DIRECTION('ref_axis',(0.,1.,0.));
#8703=DIRECTION('center_axis',(1.,8.66092162023871E-17,4.91167032291274E-17));
#8704=DIRECTION('ref_axis',(0.,1.,0.));
#8705=DIRECTION('center_axis',(1.,6.71923634350248E-17,7.34764803410285E-17));
#8706=DIRECTION('ref_axis',(0.,1.,0.));
#8707=DIRECTION('center_axis',(1.,4.1198253977918E-17,9.06438676164084E-17));
#8708=DIRECTION('ref_axis',(0.,1.,0.));
#8709=DIRECTION('center_axis',(1.,1.11713723763385E-17,9.89384015765324E-17));
#8710=DIRECTION('ref_axis',(0.,1.,0.));
#8711=DIRECTION('center_axis',(1.,-1.99490409889651E-17,9.75481554459673E-17));
#8712=DIRECTION('ref_axis',(0.,1.,0.));
#8713=DIRECTION('center_axis',(1.,-4.91167032291274E-17,8.66092162023871E-17));
#8714=DIRECTION('ref_axis',(0.,1.,0.));
#8715=DIRECTION('center_axis',(1.,-7.34764803410285E-17,6.71923634350248E-17));
#8716=DIRECTION('ref_axis',(0.,1.,0.));
#8717=DIRECTION('center_axis',(1.,-9.89384015765324E-17,1.11713723763385E-17));
#8718=DIRECTION('ref_axis',(0.,1.,0.));
#8719=DIRECTION('center_axis',(1.,-9.75481554459673E-17,-1.99490409889652E-17));
#8720=DIRECTION('ref_axis',(0.,1.,0.));
#8721=DIRECTION('center_axis',(1.,-8.66092162023871E-17,-4.91167032291274E-17));
#8722=DIRECTION('ref_axis',(0.,1.,0.));
#8723=DIRECTION('center_axis',(1.,-6.71923634350248E-17,-7.34764803410285E-17));
#8724=DIRECTION('ref_axis',(0.,1.,0.));
#8725=DIRECTION('center_axis',(1.,-4.1198253977918E-17,-9.06438676164084E-17));
#8726=DIRECTION('ref_axis',(0.,1.,0.));
#8727=DIRECTION('center_axis',(1.,-1.11713723763385E-17,-9.89384015765324E-17));
#8728=DIRECTION('ref_axis',(0.,1.,0.));
#8729=DIRECTION('center_axis',(1.,1.99490409889652E-17,-9.75481554459673E-17));
#8730=DIRECTION('ref_axis',(0.,1.,0.));
#8731=DIRECTION('center_axis',(1.,4.91167032291274E-17,-8.66092162023871E-17));
#8732=DIRECTION('ref_axis',(0.,1.,0.));
#8733=DIRECTION('center_axis',(1.,7.34764803410285E-17,-6.71923634350248E-17));
#8734=DIRECTION('ref_axis',(0.,1.,0.));
#8735=DIRECTION('center_axis',(1.,9.06438676164084E-17,-4.1198253977918E-17));
#8736=DIRECTION('ref_axis',(0.,1.,0.));
#8737=DIRECTION('center_axis',(1.,9.89384015765324E-17,-1.11713723763385E-17));
#8738=DIRECTION('ref_axis',(0.,1.,0.));
#8739=DIRECTION('center_axis',(1.,-7.34764803410285E-17,6.71923634350248E-17));
#8740=DIRECTION('ref_axis',(1.11713723763385E-17,-0.587785252292473,-0.809016994374947));
#8741=DIRECTION('center_axis',(1.,-4.91167032291274E-17,8.66092162023871E-17));
#8742=DIRECTION('ref_axis',(1.11713723763385E-17,-0.809016994374948,-0.587785252292473));
#8743=DIRECTION('center_axis',(1.,-1.99490409889651E-17,9.75481554459673E-17));
#8744=DIRECTION('ref_axis',(1.11713723763385E-17,-0.951056516295154,-0.309016994374947));
#8745=DIRECTION('center_axis',(1.,1.11713723763385E-17,9.89384015765324E-17));
#8746=DIRECTION('ref_axis',(1.11713723763385E-17,-1.,1.83697019872103E-16));
#8747=DIRECTION('center_axis',(1.,4.1198253977918E-17,9.06438676164084E-17));
#8748=DIRECTION('ref_axis',(1.11713723763385E-17,-0.951056516295153,0.309016994374948));
#8749=DIRECTION('center_axis',(1.,6.71923634350248E-17,7.34764803410285E-17));
#8750=DIRECTION('ref_axis',(1.11713723763385E-17,-0.809016994374947,0.587785252292473));
#8751=DIRECTION('center_axis',(1.,8.66092162023871E-17,4.91167032291274E-17));
#8752=DIRECTION('ref_axis',(1.11713723763385E-17,-0.587785252292473,0.809016994374947));
#8753=DIRECTION('center_axis',(1.,9.75481554459673E-17,1.99490409889651E-17));
#8754=DIRECTION('ref_axis',(1.11713723763385E-17,-0.309016994374947,0.951056516295154));
#8755=DIRECTION('center_axis',(1.,9.89384015765324E-17,-1.11713723763385E-17));
#8756=DIRECTION('ref_axis',(1.11713723763385E-17,1.22464679914735E-16,1.));
#8757=DIRECTION('center_axis',(1.,9.06438676164084E-17,-4.1198253977918E-17));
#8758=DIRECTION('ref_axis',(1.11713723763385E-17,0.309016994374948,0.951056516295153));
#8759=DIRECTION('center_axis',(1.,7.34764803410285E-17,-6.71923634350248E-17));
#8760=DIRECTION('ref_axis',(1.11713723763385E-17,0.587785252292473,0.809016994374947));
#8761=DIRECTION('center_axis',(1.,4.91167032291274E-17,-8.66092162023871E-17));
#8762=DIRECTION('ref_axis',(1.11713723763385E-17,0.809016994374947,0.587785252292473));
#8763=DIRECTION('center_axis',(1.,1.99490409889652E-17,-9.75481554459673E-17));
#8764=DIRECTION('ref_axis',(1.11713723763385E-17,0.951056516295154,0.309016994374947));
#8765=DIRECTION('center_axis',(1.,-1.11713723763385E-17,-9.89384015765324E-17));
#8766=DIRECTION('ref_axis',(1.11713723763385E-17,1.,-6.12323399573677E-17));
#8767=DIRECTION('center_axis',(1.,-4.1198253977918E-17,-9.06438676164084E-17));
#8768=DIRECTION('ref_axis',(1.11713723763385E-17,0.951056516295154,-0.309016994374948));
#8769=DIRECTION('center_axis',(1.,-6.71923634350248E-17,-7.34764803410285E-17));
#8770=DIRECTION('ref_axis',(1.11713723763385E-17,0.809016994374947,-0.587785252292473));
#8771=DIRECTION('center_axis',(1.,-8.66092162023871E-17,-4.91167032291274E-17));
#8772=DIRECTION('ref_axis',(1.11713723763385E-17,0.587785252292473,-0.809016994374947));
#8773=DIRECTION('center_axis',(1.,-9.75481554459673E-17,-1.99490409889652E-17));
#8774=DIRECTION('ref_axis',(1.11713723763385E-17,0.309016994374947,-0.951056516295154));
#8775=DIRECTION('center_axis',(1.,-9.89384015765324E-17,1.11713723763385E-17));
#8776=DIRECTION('ref_axis',(1.11713723763385E-17,0.,-1.));
#8777=DIRECTION('center_axis',(1.,0.,0.));
#8778=DIRECTION('ref_axis',(0.,0.,-1.));
#15842=CARTESIAN_POINT('',(0.,0.,0.));
#15843=CARTESIAN_POINT('Origin',(24.5,-9.875,0.));
#15844=CARTESIAN_POINT('',(22.2,-10.,0.));
#15845=CARTESIAN_POINT('',(24.5,-9.78106229945361,2.08106229945361));
#15846=CARTESIAN_POINT('Ctrl Pts',(22.2,-10.,-3.46944695195361E-17));
#15847=CARTESIAN_POINT('Ctrl Pts',(22.2,-10.,0.279281663145492));
#15848=CARTESIAN_POINT('Ctrl Pts',(22.2664319537276,-9.98711221417022,0.57235161892421));
#15849=CARTESIAN_POINT('Ctrl Pts',(22.5234308581959,-9.94287664809831,1.09963640431428));
#15850=CARTESIAN_POINT('Ctrl Pts',(22.7136761128309,-9.91228969341567,1.33407151029786));
#15851=CARTESIAN_POINT('Ctrl Pts',(23.1318392128932,-9.8577299734025,1.69022028358443));
#15852=CARTESIAN_POINT('Ctrl Pts',(23.3865793433932,-9.82998540360157,1.83883276387722));
#15853=CARTESIAN_POINT('Ctrl Pts',(23.9342975404997,-9.79141246827269,2.03424683169264));
#15854=CARTESIAN_POINT('Ctrl Pts',(24.2273042269987,-9.78106229945361,2.08106229945361));
#15855=CARTESIAN_POINT('Ctrl Pts',(24.5,-9.78106229945361,2.08106229945361));
#15856=CARTESIAN_POINT('',(26.8,-10.,0.));
#15857=CARTESIAN_POINT('Ctrl Pts',(26.8,-10.,1.04083408558608E-15));
#15858=CARTESIAN_POINT('Ctrl Pts',(26.8,-10.,-0.279281663145491));
#15859=CARTESIAN_POINT('Ctrl Pts',(26.7335680462724,-9.98711221417022,-0.57235161892421));
#15860=CARTESIAN_POINT('Ctrl Pts',(26.4765691418041,-9.94287664809831,-1.09963640431428));
#15861=CARTESIAN_POINT('Ctrl Pts',(26.2863238871692,-9.91228969341567,-1.33407151029786));
#15862=CARTESIAN_POINT('Ctrl Pts',(25.8681607871068,-9.8577299734025,-1.69022028358443));
#15863=CARTESIAN_POINT('Ctrl Pts',(25.6134206566068,-9.82998540360157,-1.83883276387722));
#15864=CARTESIAN_POINT('Ctrl Pts',(25.0657024595003,-9.79141246827269,-2.03424683169264));
#15865=CARTESIAN_POINT('Ctrl Pts',(24.7726957730013,-9.78106229945362,-2.08106229945361));
#15866=CARTESIAN_POINT('Ctrl Pts',(24.5,-9.78106229945362,-2.08106229945361));
#15867=CARTESIAN_POINT('Ctrl Pts',(24.2273042269987,-9.78106229945362,-2.08106229945361));
#15868=CARTESIAN_POINT('Ctrl Pts',(23.9342975404997,-9.79141246827269,-2.03424683169264));
#15869=CARTESIAN_POINT('Ctrl Pts',(23.3865793433932,-9.82998540360157,-1.83883276387722));
#15870=CARTESIAN_POINT('Ctrl Pts',(23.1318392128932,-9.8577299734025,-1.69022028358443));
#15871=CARTESIAN_POINT('Ctrl Pts',(22.7136761128309,-9.91228969341567,-1.33407151029786));
#15872=CARTESIAN_POINT('Ctrl Pts',(22.5234308581959,-9.94287664809831,-1.09963640431428));
#15873=CARTESIAN_POINT('Ctrl Pts',(22.2664319537276,-9.98711221417022,-0.572351618924211));
#15874=CARTESIAN_POINT('Ctrl Pts',(22.2,-10.,-0.279281663145492));
#15875=CARTESIAN_POINT('Ctrl Pts',(22.2,-10.,4.85722573273506E-16));
#15876=CARTESIAN_POINT('Ctrl Pts',(24.5,-9.78106229945361,2.08106229945361));
#15877=CARTESIAN_POINT('Ctrl Pts',(24.7726957730013,-9.78106229945361,2.08106229945361));
#15878=CARTESIAN_POINT('Ctrl Pts',(25.0657024595003,-9.79141246827269,2.03424683169264));
#15879=CARTESIAN_POINT('Ctrl Pts',(25.6134206566068,-9.82998540360157,1.83883276387722));
#15880=CARTESIAN_POINT('Ctrl Pts',(25.8681607871068,-9.8577299734025,1.69022028358443));
#15881=CARTESIAN_POINT('Ctrl Pts',(26.2863238871692,-9.91228969341567,1.33407151029786));
#15882=CARTESIAN_POINT('Ctrl Pts',(26.4765691418041,-9.94287664809831,1.09963640431428));
#15883=CARTESIAN_POINT('Ctrl Pts',(26.7335680462724,-9.98711221417022,0.572351618924211));
#15884=CARTESIAN_POINT('Ctrl Pts',(26.8,-10.,0.279281663145492));
#15885=CARTESIAN_POINT('Ctrl Pts',(26.8,-10.,-2.08166817117217E-16));
#15886=CARTESIAN_POINT('',(24.5,-9.75,2.05));
#15887=CARTESIAN_POINT('',(24.5,-9.875,2.175));
#15888=CARTESIAN_POINT('Origin',(24.5,-9.75,0.));
#15889=CARTESIAN_POINT('Origin',(24.5,-7.75,0.));
#15890=CARTESIAN_POINT('',(24.5,-5.66552071746278,2.05));
#15891=CARTESIAN_POINT('',(24.5,-7.75,2.05));
#15892=CARTESIAN_POINT('',(26.55,-6.025,-3.34230378723604E-16));
#15893=CARTESIAN_POINT('Ctrl Pts',(26.55,-6.025,1.38777878078145E-16));
#15894=CARTESIAN_POINT('Ctrl Pts',(26.55,-6.025,0.259594733817565));
#15895=CARTESIAN_POINT('Ctrl Pts',(26.4976983668916,-6.00658123724956,0.535111320788412));
#15896=CARTESIAN_POINT('Ctrl Pts',(26.287830413716,-5.94008056213222,1.03961781502895));
#15897=CARTESIAN_POINT('Ctrl Pts',(26.13037388806,-5.8928399020443,1.26876391480488));
#15898=CARTESIAN_POINT('Ctrl Pts',(25.7686724003374,-5.80318375449856,1.63046540252745));
#15899=CARTESIAN_POINT('Ctrl Pts',(25.5395625840329,-5.75468697285078,1.78785157007388));
#15900=CARTESIAN_POINT('Ctrl Pts',(25.035191264494,-5.68525838031662,1.99766693028397));
#15901=CARTESIAN_POINT('Ctrl Pts',(24.7597261277258,-5.66552071746278,2.05));
#15902=CARTESIAN_POINT('Ctrl Pts',(24.5,-5.66552071746278,2.05));
#15903=CARTESIAN_POINT('',(22.45,-6.025,-6.81175073918965E-16));
#15904=CARTESIAN_POINT('Ctrl Pts',(22.45,-6.025,-6.24500451351651E-16));
#15905=CARTESIAN_POINT('Ctrl Pts',(22.45,-6.025,-0.259594733817566));
#15906=CARTESIAN_POINT('Ctrl Pts',(22.5023016331084,-6.00658123724956,-0.535111320788414));
#15907=CARTESIAN_POINT('Ctrl Pts',(22.712169586284,-5.94008056213222,-1.03961781502895));
#15908=CARTESIAN_POINT('Ctrl Pts',(22.86962611194,-5.8928399020443,-1.26876391480488));
#15909=CARTESIAN_POINT('Ctrl Pts',(23.2313275996626,-5.80318375449856,-1.63046540252745));
#15910=CARTESIAN_POINT('Ctrl Pts',(23.4604374159671,-5.75468697285078,-1.78785157007388));
#15911=CARTESIAN_POINT('Ctrl Pts',(23.964808735506,-5.68525838031662,-1.99766693028397));
#15912=CARTESIAN_POINT('Ctrl Pts',(24.2402738722742,-5.66552071746278,-2.05));
#15913=CARTESIAN_POINT('Ctrl Pts',(24.7597261277258,-5.66552071746278,-2.05));
#15914=CARTESIAN_POINT('Ctrl Pts',(25.035191264494,-5.68525838031662,-1.99766693028397));
#15915=CARTESIAN_POINT('Ctrl Pts',(25.5395625840329,-5.75468697285078,-1.78785157007388));
#15916=CARTESIAN_POINT('Ctrl Pts',(25.7686724003374,-5.80318375449856,-1.63046540252745));
#15917=CARTESIAN_POINT('Ctrl Pts',(26.13037388806,-5.8928399020443,-1.26876391480488));
#15918=CARTESIAN_POINT('Ctrl Pts',(26.287830413716,-5.94008056213222,-1.03961781502895));
#15919=CARTESIAN_POINT('Ctrl Pts',(26.4976983668916,-6.00658123724956,-0.535111320788414));
#15920=CARTESIAN_POINT('Ctrl Pts',(26.55,-6.025,-0.259594733817566));
#15921=CARTESIAN_POINT('Ctrl Pts',(26.55,-6.025,-6.24500451351651E-16));
#15922=CARTESIAN_POINT('Ctrl Pts',(24.5,-5.66552071746278,2.05));
#15923=CARTESIAN_POINT('Ctrl Pts',(24.2402738722742,-5.66552071746278,2.05));
#15924=CARTESIAN_POINT('Ctrl Pts',(23.964808735506,-5.68525838031662,1.99766693028397));
#15925=CARTESIAN_POINT('Ctrl Pts',(23.4604374159671,-5.75468697285078,1.78785157007388));
#15926=CARTESIAN_POINT('Ctrl Pts',(23.2313275996626,-5.80318375449856,1.63046540252745));
#15927=CARTESIAN_POINT('Ctrl Pts',(22.86962611194,-5.8928399020443,1.26876391480488));
#15928=CARTESIAN_POINT('Ctrl Pts',(22.712169586284,-5.94008056213222,1.03961781502895));
#15929=CARTESIAN_POINT('Ctrl Pts',(22.5023016331084,-6.00658123724956,0.535111320788414));
#15930=CARTESIAN_POINT('Ctrl Pts',(22.45,-6.025,0.259594733817566));
#15931=CARTESIAN_POINT('Ctrl Pts',(22.45,-6.025,0.));
#15932=CARTESIAN_POINT('Origin',(24.5,0.,9.875));
#15933=CARTESIAN_POINT('',(22.2,0.,10.));
#15934=CARTESIAN_POINT('',(26.8,0.,10.));
#15935=CARTESIAN_POINT('Ctrl Pts',(22.2,-2.77555756156289E-16,10.));
#15936=CARTESIAN_POINT('Ctrl Pts',(22.2,0.279281663145492,10.));
#15937=CARTESIAN_POINT('Ctrl Pts',(22.2664319537276,0.57235161892421,9.98711221417022));
#15938=CARTESIAN_POINT('Ctrl Pts',(22.5234308581959,1.09963640431428,9.94287664809831));
#15939=CARTESIAN_POINT('Ctrl Pts',(22.7136761128309,1.33407151029786,9.91228969341567));
#15940=CARTESIAN_POINT('Ctrl Pts',(23.1318392128932,1.69022028358443,9.8577299734025));
#15941=CARTESIAN_POINT('Ctrl Pts',(23.3865793433932,1.83883276387722,9.82998540360157));
#15942=CARTESIAN_POINT('Ctrl Pts',(23.9342975404997,2.03424683169264,9.79141246827269));
#15943=CARTESIAN_POINT('Ctrl Pts',(24.2273042269987,2.08106229945361,9.78106229945362));
#15944=CARTESIAN_POINT('Ctrl Pts',(24.7726957730013,2.08106229945361,9.78106229945362));
#15945=CARTESIAN_POINT('Ctrl Pts',(25.0657024595003,2.03424683169264,9.79141246827269));
#15946=CARTESIAN_POINT('Ctrl Pts',(25.6134206566068,1.83883276387722,9.82998540360157));
#15947=CARTESIAN_POINT('Ctrl Pts',(25.8681607871068,1.69022028358443,9.8577299734025));
#15948=CARTESIAN_POINT('Ctrl Pts',(26.2863238871692,1.33407151029786,9.91228969341567));
#15949=CARTESIAN_POINT('Ctrl Pts',(26.4765691418041,1.09963640431428,9.94287664809831));
#15950=CARTESIAN_POINT('Ctrl Pts',(26.7335680462724,0.572351618924211,9.98711221417022));
#15951=CARTESIAN_POINT('Ctrl Pts',(26.8,0.279281663145492,10.));
#15952=CARTESIAN_POINT('Ctrl Pts',(26.8,0.,10.));
#15953=CARTESIAN_POINT('',(22.45,2.51052593825207E-16,9.75));
#15954=CARTESIAN_POINT('',(22.325,2.66360678814549E-16,9.875));
#15955=CARTESIAN_POINT('Origin',(24.5,0.,9.75));
#15956=CARTESIAN_POINT('Ctrl Pts',(26.8,1.31838984174237E-15,10.));
#15957=CARTESIAN_POINT('Ctrl Pts',(26.8,-0.279281663145491,10.));
#15958=CARTESIAN_POINT('Ctrl Pts',(26.7335680462724,-0.572351618924209,
9.98711221417022));
#15959=CARTESIAN_POINT('Ctrl Pts',(26.4765691418041,-1.09963640431428,9.94287664809831));
#15960=CARTESIAN_POINT('Ctrl Pts',(26.2863238871692,-1.33407151029786,9.91228969341567));
#15961=CARTESIAN_POINT('Ctrl Pts',(25.8681607871068,-1.69022028358443,9.8577299734025));
#15962=CARTESIAN_POINT('Ctrl Pts',(25.6134206566068,-1.83883276387722,9.82998540360157));
#15963=CARTESIAN_POINT('Ctrl Pts',(25.0657024595003,-2.03424683169264,9.79141246827269));
#15964=CARTESIAN_POINT('Ctrl Pts',(24.7726957730013,-2.08106229945361,9.78106229945362));
#15965=CARTESIAN_POINT('Ctrl Pts',(24.5,-2.08106229945361,9.78106229945362));
#15966=CARTESIAN_POINT('Ctrl Pts',(24.2273042269987,-2.08106229945361,9.78106229945362));
#15967=CARTESIAN_POINT('Ctrl Pts',(23.9342975404997,-2.03424683169264,9.79141246827269));
#15968=CARTESIAN_POINT('Ctrl Pts',(23.3865793433932,-1.83883276387722,9.82998540360157));
#15969=CARTESIAN_POINT('Ctrl Pts',(23.1318392128932,-1.69022028358443,9.8577299734025));
#15970=CARTESIAN_POINT('Ctrl Pts',(22.7136761128309,-1.33407151029786,9.91228969341567));
#15971=CARTESIAN_POINT('Ctrl Pts',(22.5234308581959,-1.09963640431428,9.94287664809831));
#15972=CARTESIAN_POINT('Ctrl Pts',(22.2664319537276,-0.572351618924211,
9.98711221417022));
#15973=CARTESIAN_POINT('Ctrl Pts',(22.2,-0.279281663145492,10.));
#15974=CARTESIAN_POINT('Ctrl Pts',(22.2,3.46944695195361E-16,10.));
#15975=CARTESIAN_POINT('Origin',(24.5,0.,7.75));
#15976=CARTESIAN_POINT('',(22.45,1.94915235951676E-16,6.025));
#15977=CARTESIAN_POINT('',(22.45,2.51052593825207E-16,7.75));
#15978=CARTESIAN_POINT('',(24.5,2.05,5.66552071746278));
#15979=CARTESIAN_POINT('Ctrl Pts',(24.5,2.05,5.66552071746278));
#15980=CARTESIAN_POINT('Ctrl Pts',(24.2402738722742,2.05,5.66552071746278));
#15981=CARTESIAN_POINT('Ctrl Pts',(23.964808735506,1.99766693028397,5.68525838031662));
#15982=CARTESIAN_POINT('Ctrl Pts',(23.4604374159671,1.78785157007388,5.75468697285078));
#15983=CARTESIAN_POINT('Ctrl Pts',(23.2313275996626,1.63046540252745,5.80318375449856));
#15984=CARTESIAN_POINT('Ctrl Pts',(22.86962611194,1.26876391480488,5.8928399020443));
#15985=CARTESIAN_POINT('Ctrl Pts',(22.712169586284,1.03961781502895,5.94008056213222));
#15986=CARTESIAN_POINT('Ctrl Pts',(22.5023016331084,0.535111320788414,6.00658123724956));
#15987=CARTESIAN_POINT('Ctrl Pts',(22.45,0.259594733817566,6.025));
#15988=CARTESIAN_POINT('Ctrl Pts',(22.45,2.77555756156289E-16,6.025));
#15989=CARTESIAN_POINT('Ctrl Pts',(22.45,2.08166817117217E-16,6.025));
#15990=CARTESIAN_POINT('Ctrl Pts',(22.45,-0.259594733817565,6.025));
#15991=CARTESIAN_POINT('Ctrl Pts',(22.5023016331084,-0.535111320788413,
6.00658123724956));
#15992=CARTESIAN_POINT('Ctrl Pts',(22.712169586284,-1.03961781502895,5.94008056213222));
#15993=CARTESIAN_POINT('Ctrl Pts',(22.86962611194,-1.26876391480488,5.8928399020443));
#15994=CARTESIAN_POINT('Ctrl Pts',(23.2313275996626,-1.63046540252745,5.80318375449856));
#15995=CARTESIAN_POINT('Ctrl Pts',(23.4604374159671,-1.78785157007388,5.75468697285078));
#15996=CARTESIAN_POINT('Ctrl Pts',(23.964808735506,-1.99766693028397,5.68525838031662));
#15997=CARTESIAN_POINT('Ctrl Pts',(24.2402738722742,-2.05,5.66552071746278));
#15998=CARTESIAN_POINT('Ctrl Pts',(24.7597261277258,-2.05,5.66552071746278));
#15999=CARTESIAN_POINT('Ctrl Pts',(25.035191264494,-1.99766693028397,5.68525838031662));
#16000=CARTESIAN_POINT('Ctrl Pts',(25.5395625840329,-1.78785157007388,5.75468697285078));
#16001=CARTESIAN_POINT('Ctrl Pts',(25.7686724003374,-1.63046540252745,5.80318375449856));
#16002=CARTESIAN_POINT('Ctrl Pts',(26.13037388806,-1.26876391480488,5.8928399020443));
#16003=CARTESIAN_POINT('Ctrl Pts',(26.287830413716,-1.03961781502895,5.94008056213222));
#16004=CARTESIAN_POINT('Ctrl Pts',(26.4976983668916,-0.535111320788413,
6.00658123724956));
#16005=CARTESIAN_POINT('Ctrl Pts',(26.55,-0.259594733817566,6.025));
#16006=CARTESIAN_POINT('Ctrl Pts',(26.55,0.259594733817565,6.025));
#16007=CARTESIAN_POINT('Ctrl Pts',(26.4976983668916,0.535111320788412,6.00658123724956));
#16008=CARTESIAN_POINT('Ctrl Pts',(26.287830413716,1.03961781502895,5.94008056213222));
#16009=CARTESIAN_POINT('Ctrl Pts',(26.13037388806,1.26876391480488,5.8928399020443));
#16010=CARTESIAN_POINT('Ctrl Pts',(25.7686724003374,1.63046540252745,5.80318375449856));
#16011=CARTESIAN_POINT('Ctrl Pts',(25.5395625840329,1.78785157007388,5.75468697285078));
#16012=CARTESIAN_POINT('Ctrl Pts',(25.035191264494,1.99766693028397,5.68525838031662));
#16013=CARTESIAN_POINT('Ctrl Pts',(24.7597261277258,2.05,5.66552071746278));
#16014=CARTESIAN_POINT('Ctrl Pts',(24.5,2.05,5.66552071746278));
#16015=CARTESIAN_POINT('Origin',(10.3002525316942,0.,0.));
#16016=CARTESIAN_POINT('',(10.0502525316942,6.525,-7.99082036443648E-16));
#16017=CARTESIAN_POINT('Origin',(10.0502525316942,0.,0.));
#16018=CARTESIAN_POINT('',(10.5502525316942,6.025,7.3784969648628E-16));
#16019=CARTESIAN_POINT('',(10.3002525316942,6.275,-7.68465866464964E-16));
#16020=CARTESIAN_POINT('',(10.5502525316942,-6.025,-7.3784969648628E-16));
#16021=CARTESIAN_POINT('Origin',(10.5502525316942,0.,0.));
#16022=CARTESIAN_POINT('Origin',(10.5502525316942,0.,0.));
#16023=CARTESIAN_POINT('Origin',(19.7001262658471,0.,0.));
#16024=CARTESIAN_POINT('',(28.85,6.025,-7.3784969648628E-16));
#16025=CARTESIAN_POINT('',(28.85,-6.025,-7.3784969648628E-16));
#16026=CARTESIAN_POINT('Origin',(28.85,0.,0.));
#16027=CARTESIAN_POINT('Origin',(28.85,0.,0.));
#16028=CARTESIAN_POINT('',(19.7001262658471,-6.025,-7.3784969648628E-16));
#16029=CARTESIAN_POINT('',(19.7001262658471,-6.025,-7.3784969648628E-16));
#16030=CARTESIAN_POINT('Origin',(10.0502525316942,9.16192731696939,0.));
#16031=CARTESIAN_POINT('',(10.0502525316942,8.25473589028142,-3.97495252086484));
#16032=CARTESIAN_POINT('',(10.0502525316942,8.69919410795919,-2.87487982939776));
#16033=CARTESIAN_POINT('Origin',(10.0502525316942,0.,0.));
#16034=CARTESIAN_POINT('',(10.0502525316942,9.36936257048691,-5.29266352931554));
#16035=CARTESIAN_POINT('Ctrl Pts',(10.0502525316942,8.25473589028142,-3.97495252086484));
#16036=CARTESIAN_POINT('Ctrl Pts',(10.0502525316942,8.26501573550299,-3.9787354050507));
#16037=CARTESIAN_POINT('Ctrl Pts',(10.0502525316942,8.28548315894707,-3.98649262817573));
#16038=CARTESIAN_POINT('Ctrl Pts',(10.0502525316942,8.31590749387114,-3.9987028261882));
#16039=CARTESIAN_POINT('Ctrl Pts',(10.0502525316942,8.35591866443433,-4.01613390483614));
#16040=CARTESIAN_POINT('Ctrl Pts',(10.0502525316942,8.40499831559484,-4.03985675684261));
#16041=CARTESIAN_POINT('Ctrl Pts',(10.0502525316942,8.45312379306447,-4.06554061525075));
#16042=CARTESIAN_POINT('Ctrl Pts',(10.0502525316942,8.50026327435046,-4.09322319459339));
#16043=CARTESIAN_POINT('Ctrl Pts',(10.0502525316942,8.54637031220843,-4.12295311857557));
#16044=CARTESIAN_POINT('Ctrl Pts',(10.0502525316942,8.59138312702269,-4.1547878023559));
#16045=CARTESIAN_POINT('Ctrl Pts',(10.0502525316942,8.63523937649908,-4.18877458937294));
#16046=CARTESIAN_POINT('Ctrl Pts',(10.0502525316942,8.67789021323112,-4.22493224148239));
#16047=CARTESIAN_POINT('Ctrl Pts',(10.0502525316942,8.71931397871314,-4.26323309731516));
#16048=CARTESIAN_POINT('Ctrl Pts',(10.0502525316942,8.75953271831989,-4.30358079311506));
#16049=CARTESIAN_POINT('Ctrl Pts',(10.0502525316942,8.79862131584184,-4.34579910040493));
#16050=CARTESIAN_POINT('Ctrl Pts',(10.0502525316942,8.83668400083504,-4.38966981967219));
#16051=CARTESIAN_POINT('Ctrl Pts',(10.0502525316942,8.87383549938658,-4.43496376972659));
#16052=CARTESIAN_POINT('Ctrl Pts',(10.0502525316942,8.91018166484712,-4.48147234048105));
#16053=CARTESIAN_POINT('Ctrl Pts',(10.0502525316942,8.94579828347148,-4.52904236806123));
#16054=CARTESIAN_POINT('Ctrl Pts',(10.0502525316942,8.98071755670482,-4.57759789799494));
#16055=CARTESIAN_POINT('Ctrl Pts',(10.0502525316942,9.01494291264748,-4.62711375721922));
#16056=CARTESIAN_POINT('Ctrl Pts',(10.0502525316942,9.04845937030362,-4.67759669462988));
#16057=CARTESIAN_POINT('Ctrl Pts',(10.0502525316942,9.08124522426278,-4.72906440450668));
#16058=CARTESIAN_POINT('Ctrl Pts',(10.0502525316942,9.11328422214026,-4.78152352641848));
#16059=CARTESIAN_POINT('Ctrl Pts',(10.0502525316942,9.14457471976904,-4.83495345882569));
#16060=CARTESIAN_POINT('Ctrl Pts',(10.0502525316942,9.17512453503235,-4.88931713153334));
#16061=CARTESIAN_POINT('Ctrl Pts',(10.0502525316942,9.20494811701998,-4.9445675341018));
#16062=CARTESIAN_POINT('Ctrl Pts',(10.0502525316942,9.23406306612411,-5.00065547708482));
#16063=CARTESIAN_POINT('Ctrl Pts',(10.0502525316942,9.26248702510056,-5.05753691650348));
#16064=CARTESIAN_POINT('Ctrl Pts',(10.0502525316942,9.29023486488122,-5.11517936005741));
#16065=CARTESIAN_POINT('Ctrl Pts',(10.0502525316942,9.31731853484592,-5.17355993514958));
#16066=CARTESIAN_POINT('Ctrl Pts',(10.0502525316942,9.33846108530483,-5.22084339412737));
#16067=CARTESIAN_POINT('Ctrl Pts',(10.0502525316942,9.35402540755351,-5.25662833187234));
#16068=CARTESIAN_POINT('Ctrl Pts',(10.0502525316942,9.3642718170601,-5.28062796260048));
#16069=CARTESIAN_POINT('Ctrl Pts',(10.0502525316942,9.36936257048691,-5.29266352931554));
#16070=CARTESIAN_POINT('',(10.0502525316942,7.38503851882133,-5.42237201204004));
#16071=CARTESIAN_POINT('Ctrl Pts',(10.0502525316942,9.36936257048691,-5.29266352931554));
#16072=CARTESIAN_POINT('Ctrl Pts',(10.0502525316942,9.34434525366385,-5.32181765856171));
#16073=CARTESIAN_POINT('Ctrl Pts',(10.0502525316942,9.29515286061949,-5.37803958295792));
#16074=CARTESIAN_POINT('Ctrl Pts',(10.0502525316942,9.22389100140796,-5.45611344595659));
#16075=CARTESIAN_POINT('Ctrl Pts',(10.0502525316942,9.13393772674446,-5.54767139923329));
#16076=CARTESIAN_POINT('Ctrl Pts',(10.0502525316942,9.02993079896417,-5.64122622022819));
#16077=CARTESIAN_POINT('Ctrl Pts',(10.0502525316942,8.93425530662678,-5.71414742300118));
#16078=CARTESIAN_POINT('Ctrl Pts',(10.0502525316942,8.84663552299331,-5.76712457531372));
#16079=CARTESIAN_POINT('Ctrl Pts',(10.0502525316942,8.76653902495464,-5.80148760154655));
#16080=CARTESIAN_POINT('Ctrl Pts',(10.0502525316942,8.69311263972367,-5.81936638407584));
#16081=CARTESIAN_POINT('Ctrl Pts',(10.0502525316942,8.62505870129886,-5.82399901560002));
#16082=CARTESIAN_POINT('Ctrl Pts',(10.0502525316942,8.56077284249031,-5.81938869186267));
#16083=CARTESIAN_POINT('Ctrl Pts',(10.0502525316942,8.4986070414541,-5.80964873807682));
#16084=CARTESIAN_POINT('Ctrl Pts',(10.0502525316942,8.43709945169241,-5.79843016859412));
#16085=CARTESIAN_POINT('Ctrl Pts',(10.0502525316942,8.37520120352267,-5.78835717995633));
#16086=CARTESIAN_POINT('Ctrl Pts',(10.0502525316942,8.31255178250645,-5.78034060190006));
#16087=CARTESIAN_POINT('Ctrl Pts',(10.0502525316942,8.24933415385039,-5.77394633717213));
#16088=CARTESIAN_POINT('Ctrl Pts',(10.0502525316942,8.18604879427487,-5.76796747841793));
#16089=CARTESIAN_POINT('Ctrl Pts',(10.0502525316942,8.12332066784839,-5.76091367696946));
#16090=CARTESIAN_POINT('Ctrl Pts',(10.0502525316942,8.06168961610356,-5.75154264947447));
#16091=CARTESIAN_POINT('Ctrl Pts',(10.0502525316942,8.00141929583747,-5.73934420595248));
#16092=CARTESIAN_POINT('Ctrl Pts',(10.0502525316942,7.94258074919088,-5.72431483522833));
#16093=CARTESIAN_POINT('Ctrl Pts',(10.0502525316942,7.88512587067823,-5.70675814390461));
#16094=CARTESIAN_POINT('Ctrl Pts',(10.0502525316942,7.82895914189736,-5.68709020402104));
#16095=CARTESIAN_POINT('Ctrl Pts',(10.0502525316942,7.77401905533046,-5.66561822174726));
#16096=CARTESIAN_POINT('Ctrl Pts',(10.0502525316942,7.72032292706671,-5.64241804293469));
#16097=CARTESIAN_POINT('Ctrl Pts',(10.0502525316942,7.6679311867486,-5.61742944592276));
#16098=CARTESIAN_POINT('Ctrl Pts',(10.0502525316942,7.61692741952956,-5.59050809253397));
#16099=CARTESIAN_POINT('Ctrl Pts',(10.0502525316942,7.56739405041849,-5.56148971316608));
#16100=CARTESIAN_POINT('Ctrl Pts',(10.0502525316942,7.51938467268366,-5.53026090613148));
#16101=CARTESIAN_POINT('Ctrl Pts',(10.0502525316942,7.47292244003411,-5.4967684895078));
#16102=CARTESIAN_POINT('Ctrl Pts',(10.0502525316942,7.43699488267859,-5.46814894648693));
#16103=CARTESIAN_POINT('Ctrl Pts',(10.0502525316942,7.41074614986957,-5.44565864507534));
#16104=CARTESIAN_POINT('Ctrl Pts',(10.0502525316942,7.39355619607562,-5.43021006317766));
#16105=CARTESIAN_POINT('Ctrl Pts',(10.0502525316942,7.38503851882133,-5.42237201204004));
#16106=CARTESIAN_POINT('',(10.0502525316942,6.62239247796684,-6.33125817110613));
#16107=CARTESIAN_POINT('Origin',(10.0502525316942,0.,0.));
#16108=CARTESIAN_POINT('',(10.0502525316942,7.27527035012649,-7.92891439885425));
#16109=CARTESIAN_POINT('Ctrl Pts',(10.0502525316942,6.62239247796684,-6.33125817110613));
#16110=CARTESIAN_POINT('Ctrl Pts',(10.0502525316942,6.63100021625014,-6.33803255463449));
#16111=CARTESIAN_POINT('Ctrl Pts',(10.0502525316942,6.64806877891362,-6.35173489391119));
#16112=CARTESIAN_POINT('Ctrl Pts',(10.0502525316942,6.67323088220656,-6.37274911883029));
#16113=CARTESIAN_POINT('Ctrl Pts',(10.0502525316942,6.70589726716278,-6.40169119143333));
#16114=CARTESIAN_POINT('Ctrl Pts',(10.0502525316942,6.74524402479143,-6.43941941070578));
#16115=CARTESIAN_POINT('Ctrl Pts',(10.0502525316942,6.7830773250095,-6.47871780200897));
#16116=CARTESIAN_POINT('Ctrl Pts',(10.0502525316942,6.81935524839631,-6.51961240030403));
#16117=CARTESIAN_POINT('Ctrl Pts',(10.0502525316942,6.85401859544624,-6.56213509649465));
#16118=CARTESIAN_POINT('Ctrl Pts',(10.0502525316942,6.88699086799345,-6.60632140469039));
#16119=CARTESIAN_POINT('Ctrl Pts',(10.0502525316942,6.91819814506577,-6.65219708634863));
#16120=CARTESIAN_POINT('Ctrl Pts',(10.0502525316942,6.9475881722867,-6.69976489037577));
#16121=CARTESIAN_POINT('Ctrl Pts',(10.0502525316942,6.97514889902642,-6.74899181640015));
#16122=CARTESIAN_POINT('Ctrl Pts',(10.0502525316942,7.00093106972056,-6.79979302943897));
#16123=CARTESIAN_POINT('Ctrl Pts',(10.0502525316942,7.02506036068034,-6.85202406661451));
#16124=CARTESIAN_POINT('Ctrl Pts',(10.0502525316942,7.04770332746178,-6.90550961656264));
#16125=CARTESIAN_POINT('Ctrl Pts',(10.0502525316942,7.06903990194017,-6.96006716732954));
#16126=CARTESIAN_POINT('Ctrl Pts',(10.0502525316942,7.08923522069654,-7.01553102941681));
#16127=CARTESIAN_POINT('Ctrl Pts',(10.0502525316942,7.10840869098247,-7.07177895456439));
#16128=CARTESIAN_POINT('Ctrl Pts',(10.0502525316942,7.12661440941494,-7.12874865657033));
#16129=CARTESIAN_POINT('Ctrl Pts',(10.0502525316942,7.14386341521534,-7.18641725377035));
#16130=CARTESIAN_POINT('Ctrl Pts',(10.0502525316942,7.16013937508649,-7.24478653536347));
#16131=CARTESIAN_POINT('Ctrl Pts',(10.0502525316942,7.17541617812315,-7.30386662226907));
#16132=CARTESIAN_POINT('Ctrl Pts',(10.0502525316942,7.18967631564937,-7.36365880682929));
#16133=CARTESIAN_POINT('Ctrl Pts',(10.0502525316942,7.2029245901952,-7.42414298774012));
#16134=CARTESIAN_POINT('Ctrl Pts',(10.0502525316942,7.21517989232968,-7.48528632500984));
#16135=CARTESIAN_POINT('Ctrl Pts',(10.0502525316942,7.22647049097858,-7.54704857406782));
#16136=CARTESIAN_POINT('Ctrl Pts',(10.0502525316942,7.23682832548437,-7.60938839179095));
#16137=CARTESIAN_POINT('Ctrl Pts',(10.0502525316942,7.24628378544295,-7.67226934177745));
#16138=CARTESIAN_POINT('Ctrl Pts',(10.0502525316942,7.254861054624,-7.73566511738401));
#16139=CARTESIAN_POINT('Ctrl Pts',(10.0502525316942,7.26257856558425,-7.79955765803962));
#16140=CARTESIAN_POINT('Ctrl Pts',(10.0502525316942,7.26807493359233,-7.85106030720964));
#16141=CARTESIAN_POINT('Ctrl Pts',(10.0502525316942,7.27181932978281,-7.88990344551799));
#16142=CARTESIAN_POINT('Ctrl Pts',(10.0502525316942,7.27414795055896,-7.91589476537953));
#16143=CARTESIAN_POINT('Ctrl Pts',(10.0502525316942,7.27527035012649,-7.92891439885425));
#16144=CARTESIAN_POINT('',(10.0502525316942,5.34798390487229,-7.43908464225652));
#16145=CARTESIAN_POINT('Ctrl Pts',(10.0502525316942,7.27527035012649,-7.92891439885425));
#16146=CARTESIAN_POINT('Ctrl Pts',(10.0502525316942,7.24246834654844,-7.94891084739874));
#16147=CARTESIAN_POINT('Ctrl Pts',(10.0502525316942,7.17831007049655,-7.98717978950973));
#16148=CARTESIAN_POINT('Ctrl Pts',(10.0502525316942,7.08640986444703,-8.03941132011984));
#16149=CARTESIAN_POINT('Ctrl Pts',(10.0502525316942,6.97256625288353,-8.09869101763159));
#16150=CARTESIAN_POINT('Ctrl Pts',(10.0502525316942,6.84473975688511,-8.15552703155277));
#16151=CARTESIAN_POINT('Ctrl Pts',(10.0502525316942,6.73121306554077,-8.19531386354866));
#16152=CARTESIAN_POINT('Ctrl Pts',(10.0502525316942,6.63151085898163,-8.21862212728407));
#16153=CARTESIAN_POINT('Ctrl Pts',(10.0502525316942,6.54471580350543,-8.22655212821855));
#16154=CARTESIAN_POINT('Ctrl Pts',(10.0502525316942,6.46935831372323,-8.22086585997457));
#16155=CARTESIAN_POINT('Ctrl Pts',(10.0502525316942,6.40320361025513,-8.20424193086582));
#16156=CARTESIAN_POINT('Ctrl Pts',(10.0502525316942,6.34348879371403,-8.17999182956336));
#16157=CARTESIAN_POINT('Ctrl Pts',(10.0502525316942,6.28737541479209,-8.15151829405778));
#16158=CARTESIAN_POINT('Ctrl Pts',(10.0502525316942,6.23234494937036,-8.12184190992835));
#16159=CARTESIAN_POINT('Ctrl Pts',(10.0502525316942,6.1765889417745,-8.09313431783932));
#16160=CARTESIAN_POINT('Ctrl Pts',(10.0502525316942,6.11948306053102,-8.06615036325875));
#16161=CARTESIAN_POINT('Ctrl Pts',(10.0502525316942,6.06133545932041,-8.04053373452353));
#16162=CARTESIAN_POINT('Ctrl Pts',(10.0502525316942,6.00299507467204,-8.01529125034138));
#16163=CARTESIAN_POINT('Ctrl Pts',(10.0502525316942,5.94551682580168,-7.98919862941808));
#16164=CARTESIAN_POINT('Ctrl Pts',(10.0502525316942,5.88979801918434,-7.96124121028423));
#16165=CARTESIAN_POINT('Ctrl Pts',(10.0502525316942,5.8362470647093,-7.93101524786534));
#16166=CARTESIAN_POINT('Ctrl Pts',(10.0502525316942,5.78493261248025,-7.89853935606421));
#16167=CARTESIAN_POINT('Ctrl Pts',(10.0502525316942,5.73571509186187,-7.86408741650604));
#16168=CARTESIAN_POINT('Ctrl Pts',(10.0502525316942,5.68837508612421,-7.82802562040593));
#16169=CARTESIAN_POINT('Ctrl Pts',(10.0502525316942,5.64275916621446,-7.79062713132508));
#16170=CARTESIAN_POINT('Ctrl Pts',(10.0502525316942,5.59886036305501,-7.75196943392054));
#16171=CARTESIAN_POINT('Ctrl Pts',(10.0502525316942,5.5567547581677,-7.71201392777609));
#16172=CARTESIAN_POINT('Ctrl Pts',(10.0502525316942,5.51656644870714,-7.67064916836037));
#16173=CARTESIAN_POINT('Ctrl Pts',(10.0502525316942,5.47842458761391,-7.62774439672625));
#16174=CARTESIAN_POINT('Ctrl Pts',(10.0502525316942,5.44241518816367,-7.58320832269043));
#16175=CARTESIAN_POINT('Ctrl Pts',(10.0502525316942,5.4085767049601,-7.5369975221287));
#16176=CARTESIAN_POINT('Ctrl Pts',(10.0502525316942,5.38325149258725,-7.49867649345608));
#16177=CARTESIAN_POINT('Ctrl Pts',(10.0502525316942,5.36523734954954,-7.46917564122634));
#16178=CARTESIAN_POINT('Ctrl Pts',(10.0502525316942,5.35366260632437,-7.44917117889019));
#16179=CARTESIAN_POINT('Ctrl Pts',(10.0502525316942,5.34798390487229,-7.43908464225652));
#16180=CARTESIAN_POINT('',(10.0502525316942,4.34180314898733,-8.06781615908999));
#16181=CARTESIAN_POINT('Origin',(10.0502525316942,0.,0.));
#16182=CARTESIAN_POINT('',(10.0502525316942,4.46902397810654,-9.78902788303806));
#16183=CARTESIAN_POINT('Ctrl Pts',(10.0502525316942,4.34180314898733,-8.06781615908999));
#16184=CARTESIAN_POINT('Ctrl Pts',(10.0502525316942,4.34789619493555,-8.07691891810119));
#16185=CARTESIAN_POINT('Ctrl Pts',(10.0502525316942,4.35989510698125,-8.09522509309135));
#16186=CARTESIAN_POINT('Ctrl Pts',(10.0502525316942,4.37733193665808,-8.1229863261673));
#16187=CARTESIAN_POINT('Ctrl Pts',(10.0502525316942,4.39945592264772,-8.16060634100777));
#16188=CARTESIAN_POINT('Ctrl Pts',(10.0502525316942,4.42521825196284,-8.20864682657585));
#16189=CARTESIAN_POINT('Ctrl Pts',(10.0502525316942,4.44905598790391,-8.25771295042534));
#16190=CARTESIAN_POINT('Ctrl Pts',(10.0502525316942,4.47092121748728,-8.30781651946229));
#16191=CARTESIAN_POINT('Ctrl Pts',(10.0502525316942,4.49074778380617,-8.35896957008516));
#16192=CARTESIAN_POINT('Ctrl Pts',(10.0502525316942,4.50845195831808,-8.41118223898599));
#16193=CARTESIAN_POINT('Ctrl Pts',(10.0502525316942,4.52395547727261,-8.46445618393006));
#16194=CARTESIAN_POINT('Ctrl Pts',(10.0502525316942,4.53720779434568,-8.51877787179233));
#16195=CARTESIAN_POINT('Ctrl Pts',(10.0502525316942,4.54820764638295,-8.5741121935049));
#16196=CARTESIAN_POINT('Ctrl Pts',(10.0502525316942,4.55702950966199,-8.63039414709753));
#16197=CARTESIAN_POINT('Ctrl Pts',(10.0502525316942,4.56383755094179,-8.68752517632497));
#16198=CARTESIAN_POINT('Ctrl Pts',(10.0502525316942,4.56884434816008,-8.7453900186693));
#16199=CARTESIAN_POINT('Ctrl Pts',(10.0502525316942,4.57227742599473,-8.80387069695484));
#16200=CARTESIAN_POINT('Ctrl Pts',(10.0502525316942,4.57434503953799,-8.86286066111437));
#16201=CARTESIAN_POINT('Ctrl Pts',(10.0502525316942,4.57519852862449,-8.92228054501355));
#16202=CARTESIAN_POINT('Ctrl Pts',(10.0502525316942,4.57490858968921,-8.98208782772813));
#16203=CARTESIAN_POINT('Ctrl Pts',(10.0502525316942,4.57349279247872,-9.0422641588092));
#16204=CARTESIAN_POINT('Ctrl Pts',(10.0502525316942,4.57093505021141,-9.10280619261976));
#16205=CARTESIAN_POINT('Ctrl Pts',(10.0502525316942,4.5672074024046,-9.16371548601266));
#16206=CARTESIAN_POINT('Ctrl Pts',(10.0502525316942,4.56229279796226,-9.22498785759991));
#16207=CARTESIAN_POINT('Ctrl Pts',(10.0502525316942,4.55620201600645,-9.28660567396873));
#16208=CARTESIAN_POINT('Ctrl Pts',(10.0502525316942,4.54896317065147,-9.34854353993788));
#16209=CARTESIAN_POINT('Ctrl Pts',(10.0502525316942,4.54061558349964,-9.4107719162247));
#16210=CARTESIAN_POINT('Ctrl Pts',(10.0502525316942,4.53120240639841,-9.47326135298215));
#16211=CARTESIAN_POINT('Ctrl Pts',(10.0502525316942,4.52076380103831,-9.53598658803447));
#16212=CARTESIAN_POINT('Ctrl Pts',(10.0502525316942,4.50933089675096,-9.59893007547295));
#16213=CARTESIAN_POINT('Ctrl Pts',(10.0502525316942,4.4969268049629,-9.6620803346471));
#16214=CARTESIAN_POINT('Ctrl Pts',(10.0502525316942,4.48623896772408,-9.71276073586856));
#16215=CARTESIAN_POINT('Ctrl Pts',(10.0502525316942,4.47779691026848,-9.7508598377266));
#16216=CARTESIAN_POINT('Ctrl Pts',(10.0502525316942,4.47197980068818,-9.77629863524131));
#16217=CARTESIAN_POINT('Ctrl Pts',(10.0502525316942,4.46902397810654,-9.78902788303806));
#16218=CARTESIAN_POINT('',(10.0502525316942,2.78743136471945,-8.7276078365385));
#16219=CARTESIAN_POINT('Ctrl Pts',(10.0502525316942,4.46902397810654,-9.78902788303806));
#16220=CARTESIAN_POINT('Ctrl Pts',(10.0502525316942,4.4316481764287,-9.7979092591739));
#16221=CARTESIAN_POINT('Ctrl Pts',(10.0502525316942,4.35880427644625,-9.81447918831044));
#16222=CARTESIAN_POINT('Ctrl Pts',(10.0502525316942,4.25526155603324,-9.83575560039739));
#16223=CARTESIAN_POINT('Ctrl Pts',(10.0502525316942,4.12867141346466,-9.85695433232581));
#16224=CARTESIAN_POINT('Ctrl Pts',(10.0502525316942,3.98953789729602,-9.87150803413088));
#16225=CARTESIAN_POINT('Ctrl Pts',(10.0502525316942,3.86927279048049,-9.87426588302275));
#16226=CARTESIAN_POINT('Ctrl Pts',(10.0502525316942,3.76724770763979,-9.86562368292838));
#16227=CARTESIAN_POINT('Ctrl Pts',(10.0502525316942,3.68225019949279,-9.84634441482148));
#16228=CARTESIAN_POINT('Ctrl Pts',(10.0502525316942,3.61233812130575,-9.81764970735851));
#16229=CARTESIAN_POINT('Ctrl Pts',(10.0502525316942,3.55455833609672,-9.78139648362373));
#16230=CARTESIAN_POINT('Ctrl Pts',(10.0502525316942,3.50525986412372,-9.73988037363202));
#16231=CARTESIAN_POINT('Ctrl Pts',(10.0502525316942,3.46069167580983,-9.6954604444488));
#16232=CARTESIAN_POINT('Ctrl Pts',(10.0502525316942,3.41752510010333,-9.65023117691875));
#16233=CARTESIAN_POINT('Ctrl Pts',(10.0502525316942,3.37336911957977,-9.60569908050971));
#16234=CARTESIAN_POINT('Ctrl Pts',(10.0502525316942,3.32739669964522,-9.56238912688746));
#16235=CARTESIAN_POINT('Ctrl Pts',(10.0502525316942,3.28001101822472,-9.5200576682471));
#16236=CARTESIAN_POINT('Ctrl Pts',(10.0502525316942,3.23232637183425,-9.47802246886347));
#16237=CARTESIAN_POINT('Ctrl Pts',(10.0502525316942,3.18572437199394,-9.43544515599928));
#16238=CARTESIAN_POINT('Ctrl Pts',(10.0502525316942,3.14137195551156,-9.3916380122022));
#16239=CARTESIAN_POINT('Ctrl Pts',(10.0502525316942,3.09978230736302,-9.34634325868463));
#16240=CARTESIAN_POINT('Ctrl Pts',(10.0502525316942,3.06101496566449,-9.29959981236885));
#16241=CARTESIAN_POINT('Ctrl Pts',(10.0502525316942,3.02485255677714,-9.25162502046097));
#16242=CARTESIAN_POINT('Ctrl Pts',(10.0502525316942,2.99097324368151,-9.20269934800391));
#16243=CARTESIAN_POINT('Ctrl Pts',(10.0502525316942,2.95914669449447,-9.15303517679781));
#16244=CARTESIAN_POINT('Ctrl Pts',(10.0502525316942,2.92934233715353,-9.10270404556727));
#16245=CARTESIAN_POINT('Ctrl Pts',(10.0502525316942,2.9016444576704,-9.05169275361811));
#16246=CARTESIAN_POINT('Ctrl Pts',(10.0502525316942,2.87620551770673,-8.99993365903229));
#16247=CARTESIAN_POINT('Ctrl Pts',(10.0502525316942,2.85318875574511,-8.94734231311461));
#16248=CARTESIAN_POINT('Ctrl Pts',(10.0502525316942,2.83270418548989,-8.89385847330528));
#16249=CARTESIAN_POINT('Ctrl Pts',(10.0502525316942,2.81480179823484,-8.83945272393405));
#16250=CARTESIAN_POINT('Ctrl Pts',(10.0502525316942,2.80255793908285,-8.79518133889446));
#16251=CARTESIAN_POINT('Ctrl Pts',(10.0502525316942,2.7945417356489,-8.76155768480736));
#16252=CARTESIAN_POINT('Ctrl Pts',(10.0502525316942,2.78971521950536,-8.73895551818547));
#16253=CARTESIAN_POINT('Ctrl Pts',(10.0502525316942,2.78743136471945,-8.7276078365385));
#16254=CARTESIAN_POINT('',(10.0502525316942,1.6362078766636,-9.01464008964162));
#16255=CARTESIAN_POINT('Origin',(10.0502525316942,0.,0.));
#16256=CARTESIAN_POINT('',(10.0502525316942,1.22531840158854,-10.6909231138624));
#16257=CARTESIAN_POINT('Ctrl Pts',(10.0502525316942,1.6362078766636,-9.01464008964162));
#16258=CARTESIAN_POINT('Ctrl Pts',(10.0502525316942,1.63918980048658,-9.02518018266099));
#16259=CARTESIAN_POINT('Ctrl Pts',(10.0502525316942,1.64494452480213,-9.04629825740996));
#16260=CARTESIAN_POINT('Ctrl Pts',(10.0502525316942,1.65294924248453,-9.07808903572539));
#16261=CARTESIAN_POINT('Ctrl Pts',(10.0502525316942,1.66236517961207,-9.12070448363665));
#16262=CARTESIAN_POINT('Ctrl Pts',(10.0502525316942,1.67202128432359,-9.17435469805521));
#16263=CARTESIAN_POINT('Ctrl Pts',(10.0502525316942,1.67953005230647,-9.22838562038483));
#16264=CARTESIAN_POINT('Ctrl Pts',(10.0502525316942,1.68484226707077,-9.28279367373423));
#16265=CARTESIAN_POINT('Ctrl Pts',(10.0502525316942,1.68789129020751,-9.33756986179013));
#16266=CARTESIAN_POINT('Ctrl Pts',(10.0502525316942,1.68859435873067,-9.39269795157698));
#16267=CARTESIAN_POINT('Ctrl Pts',(10.0502525316942,1.68687652711276,-9.44815533489435));
#16268=CARTESIAN_POINT('Ctrl Pts',(10.0502525316942,1.68269390490855,-9.50391352130234));
#16269=CARTESIAN_POINT('Ctrl Pts',(10.0502525316942,1.67605614008548,-9.55993872975698));
#16270=CARTESIAN_POINT('Ctrl Pts',(10.0502525316942,1.66705415050613,-9.61619215414635));
#16271=CARTESIAN_POINT('Ctrl Pts',(10.0502525316942,1.65587452359108,-9.67263079222962));
#16272=CARTESIAN_POINT('Ctrl Pts',(10.0502525316942,1.64275505105007,-9.72921071303343));
#16273=CARTESIAN_POINT('Ctrl Pts',(10.0502525316942,1.62794857866286,-9.78589002258816));
#16274=CARTESIAN_POINT('Ctrl Pts',(10.0502525316942,1.6116860945735,-9.84263174012077));
#16275=CARTESIAN_POINT('Ctrl Pts',(10.0502525316942,1.59413605700216,-9.89940715053283));
#16276=CARTESIAN_POINT('Ctrl Pts',(10.0502525316942,1.57537884194225,-9.9561976604221));
#16277=CARTESIAN_POINT('Ctrl Pts',(10.0502525316942,1.55543682981627,-10.0129912468249));
#16278=CARTESIAN_POINT('Ctrl Pts',(10.0502525316942,1.53429575504446,-10.0697797567623));
#16279=CARTESIAN_POINT('Ctrl Pts',(10.0502525316942,1.51192854453357,-10.1265560306252));
#16280=CARTESIAN_POINT('Ctrl Pts',(10.0502525316942,1.48832027384755,-10.1833108225988));
#16281=CARTESIAN_POINT('Ctrl Pts',(10.0502525316942,1.4634866435649,-10.2400306932429));
#16282=CARTESIAN_POINT('Ctrl Pts',(10.0502525316942,1.43746223933981,-10.2967001780439));
#16283=CARTESIAN_POINT('Ctrl Pts',(10.0502525316942,1.41029358637873,-10.353303334518));
#16284=CARTESIAN_POINT('Ctrl Pts',(10.0502525316942,1.38203082503059,-10.4098254888505));
#16285=CARTESIAN_POINT('Ctrl Pts',(10.0502525316942,1.35271995777451,-10.4662550259293));
#16286=CARTESIAN_POINT('Ctrl Pts',(10.0502525316942,1.32239601234813,-10.5225848780961));
#16287=CARTESIAN_POINT('Ctrl Pts',(10.0502525316942,1.29108451674038,-10.5788112684272));
#16288=CARTESIAN_POINT('Ctrl Pts',(10.0502525316942,1.26525867423012,-10.6237084709174));
#16289=CARTESIAN_POINT('Ctrl Pts',(10.0502525316942,1.24545653053149,-10.6573341307832));
#16290=CARTESIAN_POINT('Ctrl Pts',(10.0502525316942,1.23206310981062,-10.6797302792078));
#16291=CARTESIAN_POINT('Ctrl Pts',(10.0502525316942,1.22531840158854,-10.6909231138624));
#16292=CARTESIAN_POINT('',(10.0502525316942,-0.0459743785884374,-9.16181196696065));
#16293=CARTESIAN_POINT('Ctrl Pts',(10.0502525316942,1.22531840158854,-10.6909231138624));
#16294=CARTESIAN_POINT('Ctrl Pts',(10.0502525316942,1.18702740569167,-10.6878200466132));
#16295=CARTESIAN_POINT('Ctrl Pts',(10.0502525316942,1.11262835024222,-10.6810689826619));
#16296=CARTESIAN_POINT('Ctrl Pts',(10.0502525316942,1.00757859836431,-10.6693075927691));
#16297=CARTESIAN_POINT('Ctrl Pts',(10.0502525316942,0.880633449950654,-10.6503502795328));
#16298=CARTESIAN_POINT('Ctrl Pts',(10.0502525316942,0.743812271574574,-10.6211970514875));
#16299=CARTESIAN_POINT('Ctrl Pts',(10.0502525316942,0.628581135879223,-10.5866559598108));
#16300=CARTESIAN_POINT('Ctrl Pts',(10.0502525316942,0.534220102715976,-10.5469092546456));
#16301=CARTESIAN_POINT('Ctrl Pts',(10.0502525316942,0.459340290208065,-10.5023079065862));
#16302=CARTESIAN_POINT('Ctrl Pts',(10.0502525316942,0.401717104935218,-10.4534135977985));
#16303=CARTESIAN_POINT('Ctrl Pts',(10.0502525316942,0.357968125936962,-10.4010797975679));
#16304=CARTESIAN_POINT('Ctrl Pts',(10.0502525316942,0.323911676451424,-10.3463615649927));
#16305=CARTESIAN_POINT('Ctrl Pts',(10.0502525316942,0.295251323542574,-10.2903433742921));
#16306=CARTESIAN_POINT('Ctrl Pts',(10.0502525316942,0.268174082740674,-10.2339885791981));
#16307=CARTESIAN_POINT('Ctrl Pts',(10.0502525316942,0.239940424315883,-10.1779910903389));
#16308=CARTESIAN_POINT('Ctrl Pts',(10.0502525316942,0.209601566462139,-10.1225946176937));
#16309=CARTESIAN_POINT('Ctrl Pts',(10.0502525316942,0.177616245484634,-10.0676920272606));
#16310=CARTESIAN_POINT('Ctrl Pts',(10.0502525316942,0.145255042779229,-10.0129788108676));
#16311=CARTESIAN_POINT('Ctrl Pts',(10.0502525316942,0.114091020408568,-9.95808457009925));
#16312=CARTESIAN_POINT('Ctrl Pts',(10.0502525316942,0.0854465176078889,
-9.90271585009609));
#16313=CARTESIAN_POINT('Ctrl Pts',(10.0502525316942,0.0598892603187484,
-9.84678607154126));
#16314=CARTESIAN_POINT('Ctrl Pts',(10.0502525316942,0.0374638466641554,
-9.79035064491696));
#16315=CARTESIAN_POINT('Ctrl Pts',(10.0502525316942,0.0178963780480492,
-9.73354910755133));
#16316=CARTESIAN_POINT('Ctrl Pts',(10.0502525316942,0.000794100811298054,
-9.67654874444263));
#16317=CARTESIAN_POINT('Ctrl Pts',(10.0502525316942,-0.014127673269992,
-9.61948036621956));
#16318=CARTESIAN_POINT('Ctrl Pts',(10.0502525316942,-0.0269201266367305,
-9.56240256296547));
#16319=CARTESIAN_POINT('Ctrl Pts',(10.0502525316942,-0.0374990192894134,
-9.50532882588415));
#16320=CARTESIAN_POINT('Ctrl Pts',(10.0502525316942,-0.0456984490690192,
-9.44824193693312));
#16321=CARTESIAN_POINT('Ctrl Pts',(10.0502525316942,-0.0513370708710194,
-9.39111202409575));
#16322=CARTESIAN_POINT('Ctrl Pts',(10.0502525316942,-0.0542916394702433,
-9.33391578939727));
#16323=CARTESIAN_POINT('Ctrl Pts',(10.0502525316942,-0.0545055203789832,
-9.27664070503215));
#16324=CARTESIAN_POINT('Ctrl Pts',(10.0502525316942,-0.0524695120683302,
-9.23075255525014));
#16325=CARTESIAN_POINT('Ctrl Pts',(10.0502525316942,-0.0497030940542395,
-9.19629741683749));
#16326=CARTESIAN_POINT('Ctrl Pts',(10.0502525316942,-0.0473089300877004,
-9.17331000347738));
#16327=CARTESIAN_POINT('Ctrl Pts',(10.0502525316942,-0.0459743785884374,
-9.16181196696065));
#16328=CARTESIAN_POINT('',(10.0502525316942,-1.22955082275859,-9.07904823952839));
#16329=CARTESIAN_POINT('Origin',(10.0502525316942,0.,0.));
#16330=CARTESIAN_POINT('',(10.0502525316942,-2.13832987737225,-10.5463163022605));
#16331=CARTESIAN_POINT('Ctrl Pts',(10.0502525316942,-1.22955082275859,-9.07904823952839));
#16332=CARTESIAN_POINT('Ctrl Pts',(10.0502525316942,-1.22997191254093,-9.08999392881405));
#16333=CARTESIAN_POINT('Ctrl Pts',(10.0502525316942,-1.23102468846705,-9.11185671902711));
#16334=CARTESIAN_POINT('Ctrl Pts',(10.0502525316942,-1.23323564031797,-9.14456513970113));
#16335=CARTESIAN_POINT('Ctrl Pts',(10.0502525316942,-1.23744944958329,-9.18800452372235));
#16336=CARTESIAN_POINT('Ctrl Pts',(10.0502525316942,-1.24484477628256,-9.24201281020108));
#16337=CARTESIAN_POINT('Ctrl Pts',(10.0502525316942,-1.2543999867847,-9.29571960787763));
#16338=CARTESIAN_POINT('Ctrl Pts',(10.0502525316942,-1.26616078343298,-9.34910630619445));
#16339=CARTESIAN_POINT('Ctrl Pts',(10.0502525316942,-1.28018776310679,-9.40214375674832));
#16340=CARTESIAN_POINT('Ctrl Pts',(10.0502525316942,-1.29655462181801,-9.45479094589287));
#16341=CARTESIAN_POINT('Ctrl Pts',(10.0502525316942,-1.31532565068075,-9.50700321251013));
#16342=CARTESIAN_POINT('Ctrl Pts',(10.0502525316942,-1.33653378795886,-9.55873989768809));
#16343=CARTESIAN_POINT('Ctrl Pts',(10.0502525316942,-1.36015941897336,-9.60997185513068));
#16344=CARTESIAN_POINT('Ctrl Pts',(10.0502525316942,-1.38610408395052,-9.6606902731969));
#16345=CARTESIAN_POINT('Ctrl Pts',(10.0502525316942,-1.41417703928493,-9.7109119130093));
#16346=CARTESIAN_POINT('Ctrl Pts',(10.0502525316942,-1.44413855620418,-9.76066847540881));
#16347=CARTESIAN_POINT('Ctrl Pts',(10.0502525316942,-1.47573521813323,-9.80999825050556));
#16348=CARTESIAN_POINT('Ctrl Pts',(10.0502525316942,-1.50873591460517,-9.85893744675637));
#16349=CARTESIAN_POINT('Ctrl Pts',(10.0502525316942,-1.54297155887855,-9.90751081093262));
#16350=CARTESIAN_POINT('Ctrl Pts',(10.0502525316942,-1.57835996316383,-9.95572549720588));
#16351=CARTESIAN_POINT('Ctrl Pts',(10.0502525316942,-1.61487612711423,-10.003576986989));
#16352=CARTESIAN_POINT('Ctrl Pts',(10.0502525316942,-1.65253109869336,-10.0510531180319));
#16353=CARTESIAN_POINT('Ctrl Pts',(10.0502525316942,-1.69134841350201,-10.0981387150956));
#16354=CARTESIAN_POINT('Ctrl Pts',(10.0502525316942,-1.73133940840847,-10.1448203729832));
#16355=CARTESIAN_POINT('Ctrl Pts',(10.0502525316942,-1.77248499825981,-10.1910901617733));
#16356=CARTESIAN_POINT('Ctrl Pts',(10.0502525316942,-1.81474751134677,-10.2369440613944));
#16357=CARTESIAN_POINT('Ctrl Pts',(10.0502525316942,-1.85807777307013,-10.2823812867227));
#16358=CARTESIAN_POINT('Ctrl Pts',(10.0502525316942,-1.90242356266618,-10.3274033763511));
#16359=CARTESIAN_POINT('Ctrl Pts',(10.0502525316942,-1.94773753991041,-10.3720134991994));
#16360=CARTESIAN_POINT('Ctrl Pts',(10.0502525316942,-1.99398420741813,-10.4162157576914));
#16361=CARTESIAN_POINT('Ctrl Pts',(10.0502525316942,-2.04113811949547,-10.4600144483414));
#16362=CARTESIAN_POINT('Ctrl Pts',(10.0502525316942,-2.07957395387303,-10.4947336011034));
#16363=CARTESIAN_POINT('Ctrl Pts',(10.0502525316942,-2.10879781201984,-10.5205943051056));
#16364=CARTESIAN_POINT('Ctrl Pts',(10.0502525316942,-2.12845650254365,-10.5377555133892));
#16365=CARTESIAN_POINT('Ctrl Pts',(10.0502525316942,-2.13832987737225,-10.5463163022605));
#16366=CARTESIAN_POINT('',(10.0502525316942,-2.87487982939776,-8.69919410795919));
#16367=CARTESIAN_POINT('Ctrl Pts',(10.0502525316942,-2.13832987737225,-10.5463163022605));
#16368=CARTESIAN_POINT('Ctrl Pts',(10.0502525316942,-2.17378787802072,-10.531532541469));
#16369=CARTESIAN_POINT('Ctrl Pts',(10.0502525316942,-2.24245939102107,-10.5021213256069));
#16370=CARTESIAN_POINT('Ctrl Pts',(10.0502525316942,-2.33873317272541,-10.4584734205235));
#16371=CARTESIAN_POINT('Ctrl Pts',(10.0502525316942,-2.45360705137856,-10.4012157360254));
#16372=CARTESIAN_POINT('Ctrl Pts',(10.0502525316942,-2.57472288173342,-10.3312092992132));
#16373=CARTESIAN_POINT('Ctrl Pts',(10.0502525316942,-2.6736404198842,-10.2627503896831));
#16374=CARTESIAN_POINT('Ctrl Pts',(10.0502525316942,-2.751100687992,-10.1957898638803));
#16375=CARTESIAN_POINT('Ctrl Pts',(10.0502525316942,-2.80853304709422,-10.1302323265723));
#16376=CARTESIAN_POINT('Ctrl Pts',(10.0502525316942,-2.84822678059402,-10.0659245320707));
#16377=CARTESIAN_POINT('Ctrl Pts',(10.0502525316942,-2.8736624985001,-10.0026329523419));
#16378=CARTESIAN_POINT('Ctrl Pts',(10.0502525316942,-2.88914324293729,-9.94006879903196));
#16379=CARTESIAN_POINT('Ctrl Pts',(10.0502525316942,-2.89909028540996,-9.8779357976215));
#16380=CARTESIAN_POINT('Ctrl Pts',(10.0502525316942,-2.90742768231934,-9.81597187495431));
#16381=CARTESIAN_POINT('Ctrl Pts',(10.0502525316942,-2.91697531144329,-9.753990418012));
#16382=CARTESIAN_POINT('Ctrl Pts',(10.0502525316942,-2.92871082842625,-9.69193001905628));
#16383=CARTESIAN_POINT('Ctrl Pts',(10.0502525316942,-2.94216484288864,-9.62983054491074));
#16384=CARTESIAN_POINT('Ctrl Pts',(10.0502525316942,-2.95603486191442,-9.56779502233835));
#16385=CARTESIAN_POINT('Ctrl Pts',(10.0502525316942,-2.96871035517328,-9.50595728442294));
#16386=CARTESIAN_POINT('Ctrl Pts',(10.0502525316942,-2.97884302078014,-9.44444686430419));
#16387=CARTESIAN_POINT('Ctrl Pts',(10.0502525316942,-2.98586616479853,-9.38335685712271));
#16388=CARTESIAN_POINT('Ctrl Pts',(10.0502525316942,-2.98975449467364,-9.32275374295661));
#16389=CARTESIAN_POINT('Ctrl Pts',(10.0502525316942,-2.99081162285579,-9.26268559037018));
#16390=CARTESIAN_POINT('Ctrl Pts',(10.0502525316942,-2.98946277417915,-9.20319012929579));
#16391=CARTESIAN_POINT('Ctrl Pts',(10.0502525316942,-2.9860191259415,-9.144303794535));
#16392=CARTESIAN_POINT('Ctrl Pts',(10.0502525316942,-2.98054746086824,-9.08606649232432));
#16393=CARTESIAN_POINT('Ctrl Pts',(10.0502525316942,-2.97297183097014,-9.02851708515246));
#16394=CARTESIAN_POINT('Ctrl Pts',(10.0502525316942,-2.96312913325008,-8.97169046427448));
#16395=CARTESIAN_POINT('Ctrl Pts',(10.0502525316942,-2.95083766730388,-8.91561425843345));
#16396=CARTESIAN_POINT('Ctrl Pts',(10.0502525316942,-2.93597302048693,-8.86030439480771));
#16397=CARTESIAN_POINT('Ctrl Pts',(10.0502525316942,-2.91847745889582,-8.80576645976534));
#16398=CARTESIAN_POINT('Ctrl Pts',(10.0502525316942,-2.90236088180168,-8.76275339706311));
#16399=CARTESIAN_POINT('Ctrl Pts',(10.0502525316942,-2.88908263860953,-8.7308394833358));
#16400=CARTESIAN_POINT('Ctrl Pts',(10.0502525316942,-2.87970215198308,-8.70971699141988));
#16401=CARTESIAN_POINT('Ctrl Pts',(10.0502525316942,-2.87487982939776,-8.69919410795919));
#16402=CARTESIAN_POINT('',(10.0502525316942,-3.97495252086484,-8.25473589028142));
#16403=CARTESIAN_POINT('Origin',(10.0502525316942,0.,0.));
#16404=CARTESIAN_POINT('',(10.0502525316942,-5.29266352931554,-9.36936257048691));
#16405=CARTESIAN_POINT('Ctrl Pts',(10.0502525316942,-3.97495252086484,-8.25473589028142));
#16406=CARTESIAN_POINT('Ctrl Pts',(10.0502525316942,-3.9787354050507,-8.26501573550299));
#16407=CARTESIAN_POINT('Ctrl Pts',(10.0502525316942,-3.98649262817573,-8.28548315894707));
#16408=CARTESIAN_POINT('Ctrl Pts',(10.0502525316942,-3.9987028261882,-8.31590749387114));
#16409=CARTESIAN_POINT('Ctrl Pts',(10.0502525316942,-4.01613390483614,-8.35591866443433));
#16410=CARTESIAN_POINT('Ctrl Pts',(10.0502525316942,-4.03985675684261,-8.40499831559484));
#16411=CARTESIAN_POINT('Ctrl Pts',(10.0502525316942,-4.06554061525075,-8.45312379306447));
#16412=CARTESIAN_POINT('Ctrl Pts',(10.0502525316942,-4.09322319459339,-8.50026327435046));
#16413=CARTESIAN_POINT('Ctrl Pts',(10.0502525316942,-4.12295311857557,-8.54637031220843));
#16414=CARTESIAN_POINT('Ctrl Pts',(10.0502525316942,-4.1547878023559,-8.59138312702269));
#16415=CARTESIAN_POINT('Ctrl Pts',(10.0502525316942,-4.18877458937294,-8.63523937649908));
#16416=CARTESIAN_POINT('Ctrl Pts',(10.0502525316942,-4.22493224148239,-8.67789021323112));
#16417=CARTESIAN_POINT('Ctrl Pts',(10.0502525316942,-4.26323309731516,-8.71931397871314));
#16418=CARTESIAN_POINT('Ctrl Pts',(10.0502525316942,-4.30358079311506,-8.75953271831989));
#16419=CARTESIAN_POINT('Ctrl Pts',(10.0502525316942,-4.34579910040493,-8.79862131584184));
#16420=CARTESIAN_POINT('Ctrl Pts',(10.0502525316942,-4.38966981967219,-8.83668400083504));
#16421=CARTESIAN_POINT('Ctrl Pts',(10.0502525316942,-4.43496376972658,-8.87383549938658));
#16422=CARTESIAN_POINT('Ctrl Pts',(10.0502525316942,-4.48147234048105,-8.91018166484712));
#16423=CARTESIAN_POINT('Ctrl Pts',(10.0502525316942,-4.52904236806123,-8.94579828347148));
#16424=CARTESIAN_POINT('Ctrl Pts',(10.0502525316942,-4.57759789799493,-8.98071755670482));
#16425=CARTESIAN_POINT('Ctrl Pts',(10.0502525316942,-4.62711375721922,-9.01494291264748));
#16426=CARTESIAN_POINT('Ctrl Pts',(10.0502525316942,-4.67759669462988,-9.04845937030362));
#16427=CARTESIAN_POINT('Ctrl Pts',(10.0502525316942,-4.72906440450668,-9.08124522426278));
#16428=CARTESIAN_POINT('Ctrl Pts',(10.0502525316942,-4.78152352641848,-9.11328422214026));
#16429=CARTESIAN_POINT('Ctrl Pts',(10.0502525316942,-4.83495345882569,-9.14457471976904));
#16430=CARTESIAN_POINT('Ctrl Pts',(10.0502525316942,-4.88931713153333,-9.17512453503235));
#16431=CARTESIAN_POINT('Ctrl Pts',(10.0502525316942,-4.9445675341018,-9.20494811701998));
#16432=CARTESIAN_POINT('Ctrl Pts',(10.0502525316942,-5.00065547708482,-9.23406306612411));
#16433=CARTESIAN_POINT('Ctrl Pts',(10.0502525316942,-5.05753691650348,-9.26248702510056));
#16434=CARTESIAN_POINT('Ctrl Pts',(10.0502525316942,-5.11517936005741,-9.29023486488122));
#16435=CARTESIAN_POINT('Ctrl Pts',(10.0502525316942,-5.17355993514958,-9.31731853484592));
#16436=CARTESIAN_POINT('Ctrl Pts',(10.0502525316942,-5.22084339412737,-9.33846108530483));
#16437=CARTESIAN_POINT('Ctrl Pts',(10.0502525316942,-5.25662833187234,-9.35402540755351));
#16438=CARTESIAN_POINT('Ctrl Pts',(10.0502525316942,-5.28062796260048,-9.3642718170601));
#16439=CARTESIAN_POINT('Ctrl Pts',(10.0502525316942,-5.29266352931554,-9.36936257048691));
#16440=CARTESIAN_POINT('',(10.0502525316942,-5.42237201204004,-7.38503851882133));
#16441=CARTESIAN_POINT('Ctrl Pts',(10.0502525316942,-5.29266352931554,-9.36936257048691));
#16442=CARTESIAN_POINT('Ctrl Pts',(10.0502525316942,-5.32181765856171,-9.34434525366385));
#16443=CARTESIAN_POINT('Ctrl Pts',(10.0502525316942,-5.37803958295792,-9.29515286061949));
#16444=CARTESIAN_POINT('Ctrl Pts',(10.0502525316942,-5.45611344595659,-9.22389100140796));
#16445=CARTESIAN_POINT('Ctrl Pts',(10.0502525316942,-5.54767139923329,-9.13393772674446));
#16446=CARTESIAN_POINT('Ctrl Pts',(10.0502525316942,-5.64122622022819,-9.02993079896417));
#16447=CARTESIAN_POINT('Ctrl Pts',(10.0502525316942,-5.71414742300118,-8.93425530662678));
#16448=CARTESIAN_POINT('Ctrl Pts',(10.0502525316942,-5.76712457531372,-8.84663552299331));
#16449=CARTESIAN_POINT('Ctrl Pts',(10.0502525316942,-5.80148760154654,-8.76653902495464));
#16450=CARTESIAN_POINT('Ctrl Pts',(10.0502525316942,-5.81936638407584,-8.69311263972367));
#16451=CARTESIAN_POINT('Ctrl Pts',(10.0502525316942,-5.82399901560002,-8.62505870129886));
#16452=CARTESIAN_POINT('Ctrl Pts',(10.0502525316942,-5.81938869186267,-8.56077284249031));
#16453=CARTESIAN_POINT('Ctrl Pts',(10.0502525316942,-5.80964873807682,-8.4986070414541));
#16454=CARTESIAN_POINT('Ctrl Pts',(10.0502525316942,-5.79843016859412,-8.43709945169241));
#16455=CARTESIAN_POINT('Ctrl Pts',(10.0502525316942,-5.78835717995633,-8.37520120352267));
#16456=CARTESIAN_POINT('Ctrl Pts',(10.0502525316942,-5.78034060190006,-8.31255178250645));
#16457=CARTESIAN_POINT('Ctrl Pts',(10.0502525316942,-5.77394633717213,-8.24933415385039));
#16458=CARTESIAN_POINT('Ctrl Pts',(10.0502525316942,-5.76796747841793,-8.18604879427487));
#16459=CARTESIAN_POINT('Ctrl Pts',(10.0502525316942,-5.76091367696946,-8.12332066784839));
#16460=CARTESIAN_POINT('Ctrl Pts',(10.0502525316942,-5.75154264947447,-8.06168961610356));
#16461=CARTESIAN_POINT('Ctrl Pts',(10.0502525316942,-5.73934420595248,-8.00141929583747));
#16462=CARTESIAN_POINT('Ctrl Pts',(10.0502525316942,-5.72431483522833,-7.94258074919088));
#16463=CARTESIAN_POINT('Ctrl Pts',(10.0502525316942,-5.70675814390461,-7.88512587067823));
#16464=CARTESIAN_POINT('Ctrl Pts',(10.0502525316942,-5.68709020402104,-7.82895914189736));
#16465=CARTESIAN_POINT('Ctrl Pts',(10.0502525316942,-5.66561822174726,-7.77401905533046));
#16466=CARTESIAN_POINT('Ctrl Pts',(10.0502525316942,-5.64241804293469,-7.72032292706671));
#16467=CARTESIAN_POINT('Ctrl Pts',(10.0502525316942,-5.61742944592276,-7.6679311867486));
#16468=CARTESIAN_POINT('Ctrl Pts',(10.0502525316942,-5.59050809253397,-7.61692741952956));
#16469=CARTESIAN_POINT('Ctrl Pts',(10.0502525316942,-5.56148971316608,-7.56739405041849));
#16470=CARTESIAN_POINT('Ctrl Pts',(10.0502525316942,-5.53026090613148,-7.51938467268366));
#16471=CARTESIAN_POINT('Ctrl Pts',(10.0502525316942,-5.4967684895078,-7.47292244003411));
#16472=CARTESIAN_POINT('Ctrl Pts',(10.0502525316942,-5.46814894648693,-7.43699488267859));
#16473=CARTESIAN_POINT('Ctrl Pts',(10.0502525316942,-5.44565864507534,-7.41074614986957));
#16474=CARTESIAN_POINT('Ctrl Pts',(10.0502525316942,-5.43021006317766,-7.39355619607562));
#16475=CARTESIAN_POINT('Ctrl Pts',(10.0502525316942,-5.42237201204004,-7.38503851882133));
#16476=CARTESIAN_POINT('',(10.0502525316942,-6.33125817110613,-6.62239247796685));
#16477=CARTESIAN_POINT('Origin',(10.0502525316942,0.,0.));
#16478=CARTESIAN_POINT('',(10.0502525316942,-7.92891439885425,-7.2752703501265));
#16479=CARTESIAN_POINT('Ctrl Pts',(10.0502525316942,-6.33125817110613,-6.62239247796685));
#16480=CARTESIAN_POINT('Ctrl Pts',(10.0502525316942,-6.33803255463449,-6.63100021625014));
#16481=CARTESIAN_POINT('Ctrl Pts',(10.0502525316942,-6.35173489391119,-6.64806877891362));
#16482=CARTESIAN_POINT('Ctrl Pts',(10.0502525316942,-6.37274911883029,-6.67323088220656));
#16483=CARTESIAN_POINT('Ctrl Pts',(10.0502525316942,-6.40169119143333,-6.70589726716279));
#16484=CARTESIAN_POINT('Ctrl Pts',(10.0502525316942,-6.43941941070578,-6.74524402479143));
#16485=CARTESIAN_POINT('Ctrl Pts',(10.0502525316942,-6.47871780200897,-6.78307732500951));
#16486=CARTESIAN_POINT('Ctrl Pts',(10.0502525316942,-6.51961240030403,-6.81935524839631));
#16487=CARTESIAN_POINT('Ctrl Pts',(10.0502525316942,-6.56213509649465,-6.85401859544624));
#16488=CARTESIAN_POINT('Ctrl Pts',(10.0502525316942,-6.60632140469039,-6.88699086799345));
#16489=CARTESIAN_POINT('Ctrl Pts',(10.0502525316942,-6.65219708634863,-6.91819814506577));
#16490=CARTESIAN_POINT('Ctrl Pts',(10.0502525316942,-6.69976489037577,-6.9475881722867));
#16491=CARTESIAN_POINT('Ctrl Pts',(10.0502525316942,-6.74899181640015,-6.97514889902642));
#16492=CARTESIAN_POINT('Ctrl Pts',(10.0502525316942,-6.79979302943897,-7.00093106972056));
#16493=CARTESIAN_POINT('Ctrl Pts',(10.0502525316942,-6.85202406661451,-7.02506036068034));
#16494=CARTESIAN_POINT('Ctrl Pts',(10.0502525316942,-6.90550961656264,-7.04770332746178));
#16495=CARTESIAN_POINT('Ctrl Pts',(10.0502525316942,-6.96006716732954,-7.06903990194018));
#16496=CARTESIAN_POINT('Ctrl Pts',(10.0502525316942,-7.01553102941681,-7.08923522069654));
#16497=CARTESIAN_POINT('Ctrl Pts',(10.0502525316942,-7.07177895456439,-7.10840869098247));
#16498=CARTESIAN_POINT('Ctrl Pts',(10.0502525316942,-7.12874865657033,-7.12661440941494));
#16499=CARTESIAN_POINT('Ctrl Pts',(10.0502525316942,-7.18641725377035,-7.14386341521534));
#16500=CARTESIAN_POINT('Ctrl Pts',(10.0502525316942,-7.24478653536347,-7.16013937508649));
#16501=CARTESIAN_POINT('Ctrl Pts',(10.0502525316942,-7.30386662226907,-7.17541617812316));
#16502=CARTESIAN_POINT('Ctrl Pts',(10.0502525316942,-7.36365880682929,-7.18967631564937));
#16503=CARTESIAN_POINT('Ctrl Pts',(10.0502525316942,-7.42414298774012,-7.2029245901952));
#16504=CARTESIAN_POINT('Ctrl Pts',(10.0502525316942,-7.48528632500984,-7.21517989232968));
#16505=CARTESIAN_POINT('Ctrl Pts',(10.0502525316942,-7.54704857406782,-7.22647049097858));
#16506=CARTESIAN_POINT('Ctrl Pts',(10.0502525316942,-7.60938839179095,-7.23682832548438));
#16507=CARTESIAN_POINT('Ctrl Pts',(10.0502525316942,-7.67226934177745,-7.24628378544296));
#16508=CARTESIAN_POINT('Ctrl Pts',(10.0502525316942,-7.73566511738401,-7.254861054624));
#16509=CARTESIAN_POINT('Ctrl Pts',(10.0502525316942,-7.79955765803962,-7.26257856558425));
#16510=CARTESIAN_POINT('Ctrl Pts',(10.0502525316942,-7.85106030720964,-7.26807493359233));
#16511=CARTESIAN_POINT('Ctrl Pts',(10.0502525316942,-7.88990344551799,-7.27181932978281));
#16512=CARTESIAN_POINT('Ctrl Pts',(10.0502525316942,-7.91589476537953,-7.27414795055897));
#16513=CARTESIAN_POINT('Ctrl Pts',(10.0502525316942,-7.92891439885425,-7.2752703501265));
#16514=CARTESIAN_POINT('',(10.0502525316942,-7.43908464225652,-5.34798390487229));
#16515=CARTESIAN_POINT('Ctrl Pts',(10.0502525316942,-7.92891439885425,-7.2752703501265));
#16516=CARTESIAN_POINT('Ctrl Pts',(10.0502525316942,-7.94891084739874,-7.24246834654844));
#16517=CARTESIAN_POINT('Ctrl Pts',(10.0502525316942,-7.98717978950973,-7.17831007049656));
#16518=CARTESIAN_POINT('Ctrl Pts',(10.0502525316942,-8.03941132011984,-7.08640986444703));
#16519=CARTESIAN_POINT('Ctrl Pts',(10.0502525316942,-8.09869101763159,-6.97256625288353));
#16520=CARTESIAN_POINT('Ctrl Pts',(10.0502525316942,-8.15552703155277,-6.84473975688512));
#16521=CARTESIAN_POINT('Ctrl Pts',(10.0502525316942,-8.19531386354866,-6.73121306554078));
#16522=CARTESIAN_POINT('Ctrl Pts',(10.0502525316942,-8.21862212728407,-6.63151085898163));
#16523=CARTESIAN_POINT('Ctrl Pts',(10.0502525316942,-8.22655212821855,-6.54471580350543));
#16524=CARTESIAN_POINT('Ctrl Pts',(10.0502525316942,-8.22086585997457,-6.46935831372324));
#16525=CARTESIAN_POINT('Ctrl Pts',(10.0502525316942,-8.20424193086582,-6.40320361025513));
#16526=CARTESIAN_POINT('Ctrl Pts',(10.0502525316942,-8.17999182956336,-6.34348879371404));
#16527=CARTESIAN_POINT('Ctrl Pts',(10.0502525316942,-8.15151829405778,-6.2873754147921));
#16528=CARTESIAN_POINT('Ctrl Pts',(10.0502525316942,-8.12184190992835,-6.23234494937036));
#16529=CARTESIAN_POINT('Ctrl Pts',(10.0502525316942,-8.09313431783932,-6.1765889417745));
#16530=CARTESIAN_POINT('Ctrl Pts',(10.0502525316942,-8.06615036325875,-6.11948306053102));
#16531=CARTESIAN_POINT('Ctrl Pts',(10.0502525316942,-8.04053373452353,-6.06133545932041));
#16532=CARTESIAN_POINT('Ctrl Pts',(10.0502525316942,-8.01529125034138,-6.00299507467205));
#16533=CARTESIAN_POINT('Ctrl Pts',(10.0502525316942,-7.98919862941808,-5.94551682580168));
#16534=CARTESIAN_POINT('Ctrl Pts',(10.0502525316942,-7.96124121028423,-5.88979801918435));
#16535=CARTESIAN_POINT('Ctrl Pts',(10.0502525316942,-7.93101524786534,-5.83624706470931));
#16536=CARTESIAN_POINT('Ctrl Pts',(10.0502525316942,-7.89853935606421,-5.78493261248025));
#16537=CARTESIAN_POINT('Ctrl Pts',(10.0502525316942,-7.86408741650604,-5.73571509186187));
#16538=CARTESIAN_POINT('Ctrl Pts',(10.0502525316942,-7.82802562040593,-5.68837508612421));
#16539=CARTESIAN_POINT('Ctrl Pts',(10.0502525316942,-7.79062713132508,-5.64275916621446));
#16540=CARTESIAN_POINT('Ctrl Pts',(10.0502525316942,-7.75196943392054,-5.59886036305501));
#16541=CARTESIAN_POINT('Ctrl Pts',(10.0502525316942,-7.71201392777609,-5.55675475816771));
#16542=CARTESIAN_POINT('Ctrl Pts',(10.0502525316942,-7.67064916836037,-5.51656644870715));
#16543=CARTESIAN_POINT('Ctrl Pts',(10.0502525316942,-7.62774439672625,-5.47842458761391));
#16544=CARTESIAN_POINT('Ctrl Pts',(10.0502525316942,-7.58320832269043,-5.44241518816367));
#16545=CARTESIAN_POINT('Ctrl Pts',(10.0502525316942,-7.5369975221287,-5.4085767049601));
#16546=CARTESIAN_POINT('Ctrl Pts',(10.0502525316942,-7.49867649345608,-5.38325149258725));
#16547=CARTESIAN_POINT('Ctrl Pts',(10.0502525316942,-7.46917564122634,-5.36523734954955));
#16548=CARTESIAN_POINT('Ctrl Pts',(10.0502525316942,-7.44917117889019,-5.35366260632437));
#16549=CARTESIAN_POINT('Ctrl Pts',(10.0502525316942,-7.43908464225652,-5.34798390487229));
#16550=CARTESIAN_POINT('',(10.0502525316942,-8.06781615908999,-4.34180314898733));
#16551=CARTESIAN_POINT('Origin',(10.0502525316942,0.,0.));
#16552=CARTESIAN_POINT('',(10.0502525316942,-9.78902788303806,-4.46902397810655));
#16553=CARTESIAN_POINT('Ctrl Pts',(10.0502525316942,-8.06781615908999,-4.34180314898733));
#16554=CARTESIAN_POINT('Ctrl Pts',(10.0502525316942,-8.07691891810119,-4.34789619493555));
#16555=CARTESIAN_POINT('Ctrl Pts',(10.0502525316942,-8.09522509309135,-4.35989510698125));
#16556=CARTESIAN_POINT('Ctrl Pts',(10.0502525316942,-8.1229863261673,-4.37733193665808));
#16557=CARTESIAN_POINT('Ctrl Pts',(10.0502525316942,-8.16060634100777,-4.39945592264773));
#16558=CARTESIAN_POINT('Ctrl Pts',(10.0502525316942,-8.20864682657585,-4.42521825196284));
#16559=CARTESIAN_POINT('Ctrl Pts',(10.0502525316942,-8.25771295042534,-4.44905598790391));
#16560=CARTESIAN_POINT('Ctrl Pts',(10.0502525316942,-8.30781651946229,-4.47092121748728));
#16561=CARTESIAN_POINT('Ctrl Pts',(10.0502525316942,-8.35896957008516,-4.49074778380617));
#16562=CARTESIAN_POINT('Ctrl Pts',(10.0502525316942,-8.41118223898599,-4.50845195831808));
#16563=CARTESIAN_POINT('Ctrl Pts',(10.0502525316942,-8.46445618393006,-4.52395547727261));
#16564=CARTESIAN_POINT('Ctrl Pts',(10.0502525316942,-8.51877787179233,-4.53720779434568));
#16565=CARTESIAN_POINT('Ctrl Pts',(10.0502525316942,-8.5741121935049,-4.54820764638295));
#16566=CARTESIAN_POINT('Ctrl Pts',(10.0502525316942,-8.63039414709753,-4.55702950966199));
#16567=CARTESIAN_POINT('Ctrl Pts',(10.0502525316942,-8.68752517632497,-4.5638375509418));
#16568=CARTESIAN_POINT('Ctrl Pts',(10.0502525316942,-8.7453900186693,-4.56884434816008));
#16569=CARTESIAN_POINT('Ctrl Pts',(10.0502525316942,-8.80387069695484,-4.57227742599473));
#16570=CARTESIAN_POINT('Ctrl Pts',(10.0502525316942,-8.86286066111437,-4.57434503953799));
#16571=CARTESIAN_POINT('Ctrl Pts',(10.0502525316942,-8.92228054501355,-4.57519852862449));
#16572=CARTESIAN_POINT('Ctrl Pts',(10.0502525316942,-8.98208782772813,-4.57490858968921));
#16573=CARTESIAN_POINT('Ctrl Pts',(10.0502525316942,-9.0422641588092,-4.57349279247872));
#16574=CARTESIAN_POINT('Ctrl Pts',(10.0502525316942,-9.10280619261976,-4.57093505021141));
#16575=CARTESIAN_POINT('Ctrl Pts',(10.0502525316942,-9.16371548601266,-4.5672074024046));
#16576=CARTESIAN_POINT('Ctrl Pts',(10.0502525316942,-9.22498785759991,-4.56229279796226));
#16577=CARTESIAN_POINT('Ctrl Pts',(10.0502525316942,-9.28660567396873,-4.55620201600645));
#16578=CARTESIAN_POINT('Ctrl Pts',(10.0502525316942,-9.34854353993788,-4.54896317065147));
#16579=CARTESIAN_POINT('Ctrl Pts',(10.0502525316942,-9.4107719162247,-4.54061558349964));
#16580=CARTESIAN_POINT('Ctrl Pts',(10.0502525316942,-9.47326135298215,-4.53120240639841));
#16581=CARTESIAN_POINT('Ctrl Pts',(10.0502525316942,-9.53598658803447,-4.52076380103831));
#16582=CARTESIAN_POINT('Ctrl Pts',(10.0502525316942,-9.59893007547295,-4.50933089675096));
#16583=CARTESIAN_POINT('Ctrl Pts',(10.0502525316942,-9.6620803346471,-4.4969268049629));
#16584=CARTESIAN_POINT('Ctrl Pts',(10.0502525316942,-9.71276073586856,-4.48623896772408));
#16585=CARTESIAN_POINT('Ctrl Pts',(10.0502525316942,-9.7508598377266,-4.47779691026848));
#16586=CARTESIAN_POINT('Ctrl Pts',(10.0502525316942,-9.77629863524131,-4.47197980068818));
#16587=CARTESIAN_POINT('Ctrl Pts',(10.0502525316942,-9.78902788303806,-4.46902397810655));
#16588=CARTESIAN_POINT('',(10.0502525316942,-8.7276078365385,-2.78743136471945));
#16589=CARTESIAN_POINT('Ctrl Pts',(10.0502525316942,-9.78902788303806,-4.46902397810655));
#16590=CARTESIAN_POINT('Ctrl Pts',(10.0502525316942,-9.7979092591739,-4.4316481764287));
#16591=CARTESIAN_POINT('Ctrl Pts',(10.0502525316942,-9.81447918831044,-4.35880427644625));
#16592=CARTESIAN_POINT('Ctrl Pts',(10.0502525316942,-9.83575560039739,-4.25526155603324));
#16593=CARTESIAN_POINT('Ctrl Pts',(10.0502525316942,-9.85695433232581,-4.12867141346467));
#16594=CARTESIAN_POINT('Ctrl Pts',(10.0502525316942,-9.87150803413088,-3.98953789729602));
#16595=CARTESIAN_POINT('Ctrl Pts',(10.0502525316942,-9.87426588302275,-3.86927279048049));
#16596=CARTESIAN_POINT('Ctrl Pts',(10.0502525316942,-9.86562368292838,-3.76724770763979));
#16597=CARTESIAN_POINT('Ctrl Pts',(10.0502525316942,-9.84634441482148,-3.68225019949279));
#16598=CARTESIAN_POINT('Ctrl Pts',(10.0502525316942,-9.81764970735851,-3.61233812130575));
#16599=CARTESIAN_POINT('Ctrl Pts',(10.0502525316942,-9.78139648362373,-3.55455833609672));
#16600=CARTESIAN_POINT('Ctrl Pts',(10.0502525316942,-9.73988037363202,-3.50525986412372));
#16601=CARTESIAN_POINT('Ctrl Pts',(10.0502525316942,-9.6954604444488,-3.46069167580983));
#16602=CARTESIAN_POINT('Ctrl Pts',(10.0502525316942,-9.65023117691875,-3.41752510010333));
#16603=CARTESIAN_POINT('Ctrl Pts',(10.0502525316942,-9.60569908050971,-3.37336911957978));
#16604=CARTESIAN_POINT('Ctrl Pts',(10.0502525316942,-9.56238912688746,-3.32739669964523));
#16605=CARTESIAN_POINT('Ctrl Pts',(10.0502525316942,-9.5200576682471,-3.28001101822472));
#16606=CARTESIAN_POINT('Ctrl Pts',(10.0502525316942,-9.47802246886347,-3.23232637183425));
#16607=CARTESIAN_POINT('Ctrl Pts',(10.0502525316942,-9.43544515599928,-3.18572437199394));
#16608=CARTESIAN_POINT('Ctrl Pts',(10.0502525316942,-9.3916380122022,-3.14137195551156));
#16609=CARTESIAN_POINT('Ctrl Pts',(10.0502525316942,-9.34634325868463,-3.09978230736302));
#16610=CARTESIAN_POINT('Ctrl Pts',(10.0502525316942,-9.29959981236885,-3.06101496566449));
#16611=CARTESIAN_POINT('Ctrl Pts',(10.0502525316942,-9.25162502046097,-3.02485255677714));
#16612=CARTESIAN_POINT('Ctrl Pts',(10.0502525316942,-9.20269934800391,-2.99097324368151));
#16613=CARTESIAN_POINT('Ctrl Pts',(10.0502525316942,-9.15303517679781,-2.95914669449447));
#16614=CARTESIAN_POINT('Ctrl Pts',(10.0502525316942,-9.10270404556727,-2.92934233715353));
#16615=CARTESIAN_POINT('Ctrl Pts',(10.0502525316942,-9.05169275361811,-2.9016444576704));
#16616=CARTESIAN_POINT('Ctrl Pts',(10.0502525316942,-8.99993365903229,-2.87620551770673));
#16617=CARTESIAN_POINT('Ctrl Pts',(10.0502525316942,-8.94734231311461,-2.85318875574511));
#16618=CARTESIAN_POINT('Ctrl Pts',(10.0502525316942,-8.89385847330528,-2.83270418548989));
#16619=CARTESIAN_POINT('Ctrl Pts',(10.0502525316942,-8.83945272393405,-2.81480179823484));
#16620=CARTESIAN_POINT('Ctrl Pts',(10.0502525316942,-8.79518133889446,-2.80255793908285));
#16621=CARTESIAN_POINT('Ctrl Pts',(10.0502525316942,-8.76155768480736,-2.7945417356489));
#16622=CARTESIAN_POINT('Ctrl Pts',(10.0502525316942,-8.73895551818547,-2.78971521950536));
#16623=CARTESIAN_POINT('Ctrl Pts',(10.0502525316942,-8.7276078365385,-2.78743136471945));
#16624=CARTESIAN_POINT('',(10.0502525316942,-9.01464008964162,-1.6362078766636));
#16625=CARTESIAN_POINT('Origin',(10.0502525316942,0.,0.));
#16626=CARTESIAN_POINT('',(10.0502525316942,-10.6909231138624,-1.22531840158854));
#16627=CARTESIAN_POINT('Ctrl Pts',(10.0502525316942,-9.01464008964162,-1.6362078766636));
#16628=CARTESIAN_POINT('Ctrl Pts',(10.0502525316942,-9.02518018266099,-1.63918980048658));
#16629=CARTESIAN_POINT('Ctrl Pts',(10.0502525316942,-9.04629825740996,-1.64494452480213));
#16630=CARTESIAN_POINT('Ctrl Pts',(10.0502525316942,-9.07808903572539,-1.65294924248453));
#16631=CARTESIAN_POINT('Ctrl Pts',(10.0502525316942,-9.12070448363665,-1.66236517961207));
#16632=CARTESIAN_POINT('Ctrl Pts',(10.0502525316942,-9.17435469805521,-1.67202128432359));
#16633=CARTESIAN_POINT('Ctrl Pts',(10.0502525316942,-9.22838562038483,-1.67953005230647));
#16634=CARTESIAN_POINT('Ctrl Pts',(10.0502525316942,-9.28279367373423,-1.68484226707077));
#16635=CARTESIAN_POINT('Ctrl Pts',(10.0502525316942,-9.33756986179013,-1.68789129020751));
#16636=CARTESIAN_POINT('Ctrl Pts',(10.0502525316942,-9.39269795157698,-1.68859435873067));
#16637=CARTESIAN_POINT('Ctrl Pts',(10.0502525316942,-9.44815533489435,-1.68687652711276));
#16638=CARTESIAN_POINT('Ctrl Pts',(10.0502525316942,-9.50391352130234,-1.68269390490855));
#16639=CARTESIAN_POINT('Ctrl Pts',(10.0502525316942,-9.55993872975698,-1.67605614008548));
#16640=CARTESIAN_POINT('Ctrl Pts',(10.0502525316942,-9.61619215414635,-1.66705415050613));
#16641=CARTESIAN_POINT('Ctrl Pts',(10.0502525316942,-9.67263079222962,-1.65587452359108));
#16642=CARTESIAN_POINT('Ctrl Pts',(10.0502525316942,-9.72921071303343,-1.64275505105007));
#16643=CARTESIAN_POINT('Ctrl Pts',(10.0502525316942,-9.78589002258816,-1.62794857866286));
#16644=CARTESIAN_POINT('Ctrl Pts',(10.0502525316942,-9.84263174012077,-1.6116860945735));
#16645=CARTESIAN_POINT('Ctrl Pts',(10.0502525316942,-9.89940715053283,-1.59413605700216));
#16646=CARTESIAN_POINT('Ctrl Pts',(10.0502525316942,-9.9561976604221,-1.57537884194225));
#16647=CARTESIAN_POINT('Ctrl Pts',(10.0502525316942,-10.0129912468249,-1.55543682981628));
#16648=CARTESIAN_POINT('Ctrl Pts',(10.0502525316942,-10.0697797567623,-1.53429575504446));
#16649=CARTESIAN_POINT('Ctrl Pts',(10.0502525316942,-10.1265560306252,-1.51192854453357));
#16650=CARTESIAN_POINT('Ctrl Pts',(10.0502525316942,-10.1833108225988,-1.48832027384755));
#16651=CARTESIAN_POINT('Ctrl Pts',(10.0502525316942,-10.2400306932429,-1.4634866435649));
#16652=CARTESIAN_POINT('Ctrl Pts',(10.0502525316942,-10.2967001780439,-1.43746223933981));
#16653=CARTESIAN_POINT('Ctrl Pts',(10.0502525316942,-10.353303334518,-1.41029358637873));
#16654=CARTESIAN_POINT('Ctrl Pts',(10.0502525316942,-10.4098254888505,-1.38203082503059));
#16655=CARTESIAN_POINT('Ctrl Pts',(10.0502525316942,-10.4662550259293,-1.35271995777451));
#16656=CARTESIAN_POINT('Ctrl Pts',(10.0502525316942,-10.5225848780961,-1.32239601234813));
#16657=CARTESIAN_POINT('Ctrl Pts',(10.0502525316942,-10.5788112684272,-1.29108451674038));
#16658=CARTESIAN_POINT('Ctrl Pts',(10.0502525316942,-10.6237084709174,-1.26525867423012));
#16659=CARTESIAN_POINT('Ctrl Pts',(10.0502525316942,-10.6573341307832,-1.24545653053149));
#16660=CARTESIAN_POINT('Ctrl Pts',(10.0502525316942,-10.6797302792078,-1.23206310981063));
#16661=CARTESIAN_POINT('Ctrl Pts',(10.0502525316942,-10.6909231138624,-1.22531840158854));
#16662=CARTESIAN_POINT('',(10.0502525316942,-9.16181196696065,0.0459743785884369));
#16663=CARTESIAN_POINT('Ctrl Pts',(10.0502525316942,-10.6909231138624,-1.22531840158854));
#16664=CARTESIAN_POINT('Ctrl Pts',(10.0502525316942,-10.6878200466132,-1.18702740569167));
#16665=CARTESIAN_POINT('Ctrl Pts',(10.0502525316942,-10.6810689826619,-1.11262835024222));
#16666=CARTESIAN_POINT('Ctrl Pts',(10.0502525316942,-10.6693075927691,-1.00757859836431));
#16667=CARTESIAN_POINT('Ctrl Pts',(10.0502525316942,-10.6503502795328,-0.880633449950655));
#16668=CARTESIAN_POINT('Ctrl Pts',(10.0502525316942,-10.6211970514875,-0.743812271574575));
#16669=CARTESIAN_POINT('Ctrl Pts',(10.0502525316942,-10.5866559598108,-0.628581135879224));
#16670=CARTESIAN_POINT('Ctrl Pts',(10.0502525316942,-10.5469092546456,-0.534220102715976));
#16671=CARTESIAN_POINT('Ctrl Pts',(10.0502525316942,-10.5023079065862,-0.459340290208065));
#16672=CARTESIAN_POINT('Ctrl Pts',(10.0502525316942,-10.4534135977985,-0.401717104935219));
#16673=CARTESIAN_POINT('Ctrl Pts',(10.0502525316942,-10.4010797975679,-0.357968125936962));
#16674=CARTESIAN_POINT('Ctrl Pts',(10.0502525316942,-10.3463615649927,-0.323911676451424));
#16675=CARTESIAN_POINT('Ctrl Pts',(10.0502525316942,-10.2903433742921,-0.295251323542575));
#16676=CARTESIAN_POINT('Ctrl Pts',(10.0502525316942,-10.2339885791981,-0.268174082740675));
#16677=CARTESIAN_POINT('Ctrl Pts',(10.0502525316942,-10.1779910903389,-0.239940424315884));
#16678=CARTESIAN_POINT('Ctrl Pts',(10.0502525316942,-10.1225946176937,-0.20960156646214));
#16679=CARTESIAN_POINT('Ctrl Pts',(10.0502525316942,-10.0676920272606,-0.177616245484634));
#16680=CARTESIAN_POINT('Ctrl Pts',(10.0502525316942,-10.0129788108676,-0.14525504277923));
#16681=CARTESIAN_POINT('Ctrl Pts',(10.0502525316942,-9.95808457009925,-0.114091020408568));
#16682=CARTESIAN_POINT('Ctrl Pts',(10.0502525316942,-9.90271585009609,-0.0854465176078895));
#16683=CARTESIAN_POINT('Ctrl Pts',(10.0502525316942,-9.84678607154126,-0.059889260318749));
#16684=CARTESIAN_POINT('Ctrl Pts',(10.0502525316942,-9.79035064491696,-0.037463846664156));
#16685=CARTESIAN_POINT('Ctrl Pts',(10.0502525316942,-9.73354910755133,-0.0178963780480498));
#16686=CARTESIAN_POINT('Ctrl Pts',(10.0502525316942,-9.67654874444263,-0.000794100811298646));
#16687=CARTESIAN_POINT('Ctrl Pts',(10.0502525316942,-9.61948036621956,0.0141276732699914));
#16688=CARTESIAN_POINT('Ctrl Pts',(10.0502525316942,-9.56240256296547,0.0269201266367299));
#16689=CARTESIAN_POINT('Ctrl Pts',(10.0502525316942,-9.50532882588415,0.0374990192894128));
#16690=CARTESIAN_POINT('Ctrl Pts',(10.0502525316942,-9.44824193693312,0.0456984490690186));
#16691=CARTESIAN_POINT('Ctrl Pts',(10.0502525316942,-9.39111202409575,0.0513370708710189));
#16692=CARTESIAN_POINT('Ctrl Pts',(10.0502525316942,-9.33391578939727,0.0542916394702428));
#16693=CARTESIAN_POINT('Ctrl Pts',(10.0502525316942,-9.27664070503215,0.0545055203789827));
#16694=CARTESIAN_POINT('Ctrl Pts',(10.0502525316942,-9.23075255525014,0.0524695120683297));
#16695=CARTESIAN_POINT('Ctrl Pts',(10.0502525316942,-9.19629741683749,0.049703094054239));
#16696=CARTESIAN_POINT('Ctrl Pts',(10.0502525316942,-9.17331000347738,0.0473089300876998));
#16697=CARTESIAN_POINT('Ctrl Pts',(10.0502525316942,-9.16181196696065,0.0459743785884369));
#16698=CARTESIAN_POINT('',(10.0502525316942,-9.07904823952839,1.22955082275859));
#16699=CARTESIAN_POINT('Origin',(10.0502525316942,0.,0.));
#16700=CARTESIAN_POINT('',(10.0502525316942,-10.5463163022605,2.13832987737225));
#16701=CARTESIAN_POINT('Ctrl Pts',(10.0502525316942,-9.07904823952839,1.22955082275859));
#16702=CARTESIAN_POINT('Ctrl Pts',(10.0502525316942,-9.08999392881405,1.22997191254093));
#16703=CARTESIAN_POINT('Ctrl Pts',(10.0502525316942,-9.11185671902711,1.23102468846705));
#16704=CARTESIAN_POINT('Ctrl Pts',(10.0502525316942,-9.14456513970113,1.23323564031797));
#16705=CARTESIAN_POINT('Ctrl Pts',(10.0502525316942,-9.18800452372235,1.23744944958329));
#16706=CARTESIAN_POINT('Ctrl Pts',(10.0502525316942,-9.24201281020108,1.24484477628256));
#16707=CARTESIAN_POINT('Ctrl Pts',(10.0502525316942,-9.29571960787763,1.2543999867847));
#16708=CARTESIAN_POINT('Ctrl Pts',(10.0502525316942,-9.34910630619445,1.26616078343298));
#16709=CARTESIAN_POINT('Ctrl Pts',(10.0502525316942,-9.40214375674832,1.28018776310679));
#16710=CARTESIAN_POINT('Ctrl Pts',(10.0502525316942,-9.45479094589287,1.29655462181801));
#16711=CARTESIAN_POINT('Ctrl Pts',(10.0502525316942,-9.50700321251013,1.31532565068075));
#16712=CARTESIAN_POINT('Ctrl Pts',(10.0502525316942,-9.55873989768809,1.33653378795886));
#16713=CARTESIAN_POINT('Ctrl Pts',(10.0502525316942,-9.60997185513068,1.36015941897336));
#16714=CARTESIAN_POINT('Ctrl Pts',(10.0502525316942,-9.6606902731969,1.38610408395052));
#16715=CARTESIAN_POINT('Ctrl Pts',(10.0502525316942,-9.7109119130093,1.41417703928493));
#16716=CARTESIAN_POINT('Ctrl Pts',(10.0502525316942,-9.76066847540881,1.44413855620418));
#16717=CARTESIAN_POINT('Ctrl Pts',(10.0502525316942,-9.80999825050556,1.47573521813323));
#16718=CARTESIAN_POINT('Ctrl Pts',(10.0502525316942,-9.85893744675637,1.50873591460517));
#16719=CARTESIAN_POINT('Ctrl Pts',(10.0502525316942,-9.90751081093262,1.54297155887855));
#16720=CARTESIAN_POINT('Ctrl Pts',(10.0502525316942,-9.95572549720588,1.57835996316383));
#16721=CARTESIAN_POINT('Ctrl Pts',(10.0502525316942,-10.003576986989,1.61487612711423));
#16722=CARTESIAN_POINT('Ctrl Pts',(10.0502525316942,-10.0510531180319,1.65253109869336));
#16723=CARTESIAN_POINT('Ctrl Pts',(10.0502525316942,-10.0981387150956,1.69134841350201));
#16724=CARTESIAN_POINT('Ctrl Pts',(10.0502525316942,-10.1448203729832,1.73133940840846));
#16725=CARTESIAN_POINT('Ctrl Pts',(10.0502525316942,-10.1910901617733,1.77248499825981));
#16726=CARTESIAN_POINT('Ctrl Pts',(10.0502525316942,-10.2369440613944,1.81474751134677));
#16727=CARTESIAN_POINT('Ctrl Pts',(10.0502525316942,-10.2823812867227,1.85807777307013));
#16728=CARTESIAN_POINT('Ctrl Pts',(10.0502525316942,-10.3274033763511,1.90242356266618));
#16729=CARTESIAN_POINT('Ctrl Pts',(10.0502525316942,-10.3720134991994,1.94773753991041));
#16730=CARTESIAN_POINT('Ctrl Pts',(10.0502525316942,-10.4162157576914,1.99398420741813));
#16731=CARTESIAN_POINT('Ctrl Pts',(10.0502525316942,-10.4600144483414,2.04113811949547));
#16732=CARTESIAN_POINT('Ctrl Pts',(10.0502525316942,-10.4947336011034,2.07957395387303));
#16733=CARTESIAN_POINT('Ctrl Pts',(10.0502525316942,-10.5205943051056,2.10879781201984));
#16734=CARTESIAN_POINT('Ctrl Pts',(10.0502525316942,-10.5377555133892,2.12845650254365));
#16735=CARTESIAN_POINT('Ctrl Pts',(10.0502525316942,-10.5463163022605,2.13832987737225));
#16736=CARTESIAN_POINT('',(10.0502525316942,-8.69919410795919,2.87487982939776));
#16737=CARTESIAN_POINT('Ctrl Pts',(10.0502525316942,-10.5463163022605,2.13832987737225));
#16738=CARTESIAN_POINT('Ctrl Pts',(10.0502525316942,-10.531532541469,2.17378787802072));
#16739=CARTESIAN_POINT('Ctrl Pts',(10.0502525316942,-10.5021213256069,2.24245939102107));
#16740=CARTESIAN_POINT('Ctrl Pts',(10.0502525316942,-10.4584734205235,2.33873317272541));
#16741=CARTESIAN_POINT('Ctrl Pts',(10.0502525316942,-10.4012157360254,2.45360705137856));
#16742=CARTESIAN_POINT('Ctrl Pts',(10.0502525316942,-10.3312092992132,2.57472288173342));
#16743=CARTESIAN_POINT('Ctrl Pts',(10.0502525316942,-10.2627503896831,2.6736404198842));
#16744=CARTESIAN_POINT('Ctrl Pts',(10.0502525316942,-10.1957898638803,2.751100687992));
#16745=CARTESIAN_POINT('Ctrl Pts',(10.0502525316942,-10.1302323265723,2.80853304709422));
#16746=CARTESIAN_POINT('Ctrl Pts',(10.0502525316942,-10.0659245320707,2.84822678059402));
#16747=CARTESIAN_POINT('Ctrl Pts',(10.0502525316942,-10.0026329523419,2.8736624985001));
#16748=CARTESIAN_POINT('Ctrl Pts',(10.0502525316942,-9.94006879903196,2.88914324293729));
#16749=CARTESIAN_POINT('Ctrl Pts',(10.0502525316942,-9.8779357976215,2.89909028540996));
#16750=CARTESIAN_POINT('Ctrl Pts',(10.0502525316942,-9.81597187495431,2.90742768231934));
#16751=CARTESIAN_POINT('Ctrl Pts',(10.0502525316942,-9.753990418012,2.91697531144329));
#16752=CARTESIAN_POINT('Ctrl Pts',(10.0502525316942,-9.69193001905628,2.92871082842625));
#16753=CARTESIAN_POINT('Ctrl Pts',(10.0502525316942,-9.62983054491074,2.94216484288864));
#16754=CARTESIAN_POINT('Ctrl Pts',(10.0502525316942,-9.56779502233835,2.95603486191442));
#16755=CARTESIAN_POINT('Ctrl Pts',(10.0502525316942,-9.50595728442294,2.96871035517328));
#16756=CARTESIAN_POINT('Ctrl Pts',(10.0502525316942,-9.44444686430419,2.97884302078013));
#16757=CARTESIAN_POINT('Ctrl Pts',(10.0502525316942,-9.38335685712271,2.98586616479853));
#16758=CARTESIAN_POINT('Ctrl Pts',(10.0502525316942,-9.32275374295661,2.98975449467364));
#16759=CARTESIAN_POINT('Ctrl Pts',(10.0502525316942,-9.26268559037018,2.99081162285579));
#16760=CARTESIAN_POINT('Ctrl Pts',(10.0502525316942,-9.20319012929579,2.98946277417915));
#16761=CARTESIAN_POINT('Ctrl Pts',(10.0502525316942,-9.144303794535,2.9860191259415));
#16762=CARTESIAN_POINT('Ctrl Pts',(10.0502525316942,-9.08606649232432,2.98054746086824));
#16763=CARTESIAN_POINT('Ctrl Pts',(10.0502525316942,-9.02851708515246,2.97297183097014));
#16764=CARTESIAN_POINT('Ctrl Pts',(10.0502525316942,-8.97169046427448,2.96312913325008));
#16765=CARTESIAN_POINT('Ctrl Pts',(10.0502525316942,-8.91561425843345,2.95083766730388));
#16766=CARTESIAN_POINT('Ctrl Pts',(10.0502525316942,-8.86030439480771,2.93597302048693));
#16767=CARTESIAN_POINT('Ctrl Pts',(10.0502525316942,-8.80576645976534,2.91847745889582));
#16768=CARTESIAN_POINT('Ctrl Pts',(10.0502525316942,-8.76275339706311,2.90236088180168));
#16769=CARTESIAN_POINT('Ctrl Pts',(10.0502525316942,-8.7308394833358,2.88908263860953));
#16770=CARTESIAN_POINT('Ctrl Pts',(10.0502525316942,-8.70971699141988,2.87970215198308));
#16771=CARTESIAN_POINT('Ctrl Pts',(10.0502525316942,-8.69919410795919,2.87487982939776));
#16772=CARTESIAN_POINT('',(10.0502525316942,-8.25473589028142,3.97495252086484));
#16773=CARTESIAN_POINT('Origin',(10.0502525316942,0.,0.));
#16774=CARTESIAN_POINT('',(10.0502525316942,-9.36936257048691,5.29266352931554));
#16775=CARTESIAN_POINT('Ctrl Pts',(10.0502525316942,-8.25473589028142,3.97495252086484));
#16776=CARTESIAN_POINT('Ctrl Pts',(10.0502525316942,-8.26501573550299,3.9787354050507));
#16777=CARTESIAN_POINT('Ctrl Pts',(10.0502525316942,-8.28548315894707,3.98649262817573));
#16778=CARTESIAN_POINT('Ctrl Pts',(10.0502525316942,-8.31590749387114,3.9987028261882));
#16779=CARTESIAN_POINT('Ctrl Pts',(10.0502525316942,-8.35591866443433,4.01613390483614));
#16780=CARTESIAN_POINT('Ctrl Pts',(10.0502525316942,-8.40499831559484,4.03985675684261));
#16781=CARTESIAN_POINT('Ctrl Pts',(10.0502525316942,-8.45312379306447,4.06554061525075));
#16782=CARTESIAN_POINT('Ctrl Pts',(10.0502525316942,-8.50026327435046,4.09322319459339));
#16783=CARTESIAN_POINT('Ctrl Pts',(10.0502525316942,-8.54637031220843,4.12295311857557));
#16784=CARTESIAN_POINT('Ctrl Pts',(10.0502525316942,-8.59138312702269,4.1547878023559));
#16785=CARTESIAN_POINT('Ctrl Pts',(10.0502525316942,-8.63523937649908,4.18877458937294));
#16786=CARTESIAN_POINT('Ctrl Pts',(10.0502525316942,-8.67789021323112,4.22493224148239));
#16787=CARTESIAN_POINT('Ctrl Pts',(10.0502525316942,-8.71931397871314,4.26323309731516));
#16788=CARTESIAN_POINT('Ctrl Pts',(10.0502525316942,-8.75953271831989,4.30358079311506));
#16789=CARTESIAN_POINT('Ctrl Pts',(10.0502525316942,-8.79862131584184,4.34579910040493));
#16790=CARTESIAN_POINT('Ctrl Pts',(10.0502525316942,-8.83668400083504,4.38966981967219));
#16791=CARTESIAN_POINT('Ctrl Pts',(10.0502525316942,-8.87383549938658,4.43496376972658));
#16792=CARTESIAN_POINT('Ctrl Pts',(10.0502525316942,-8.91018166484712,4.48147234048105));
#16793=CARTESIAN_POINT('Ctrl Pts',(10.0502525316942,-8.94579828347148,4.52904236806123));
#16794=CARTESIAN_POINT('Ctrl Pts',(10.0502525316942,-8.98071755670482,4.57759789799493));
#16795=CARTESIAN_POINT('Ctrl Pts',(10.0502525316942,-9.01494291264748,4.62711375721922));
#16796=CARTESIAN_POINT('Ctrl Pts',(10.0502525316942,-9.04845937030362,4.67759669462988));
#16797=CARTESIAN_POINT('Ctrl Pts',(10.0502525316942,-9.08124522426278,4.72906440450668));
#16798=CARTESIAN_POINT('Ctrl Pts',(10.0502525316942,-9.11328422214026,4.78152352641848));
#16799=CARTESIAN_POINT('Ctrl Pts',(10.0502525316942,-9.14457471976904,4.83495345882569));
#16800=CARTESIAN_POINT('Ctrl Pts',(10.0502525316942,-9.17512453503235,4.88931713153333));
#16801=CARTESIAN_POINT('Ctrl Pts',(10.0502525316942,-9.20494811701998,4.9445675341018));
#16802=CARTESIAN_POINT('Ctrl Pts',(10.0502525316942,-9.23406306612411,5.00065547708482));
#16803=CARTESIAN_POINT('Ctrl Pts',(10.0502525316942,-9.26248702510056,5.05753691650348));
#16804=CARTESIAN_POINT('Ctrl Pts',(10.0502525316942,-9.29023486488122,5.11517936005741));
#16805=CARTESIAN_POINT('Ctrl Pts',(10.0502525316942,-9.31731853484592,5.17355993514958));
#16806=CARTESIAN_POINT('Ctrl Pts',(10.0502525316942,-9.33846108530483,5.22084339412737));
#16807=CARTESIAN_POINT('Ctrl Pts',(10.0502525316942,-9.35402540755351,5.25662833187234));
#16808=CARTESIAN_POINT('Ctrl Pts',(10.0502525316942,-9.3642718170601,5.28062796260048));
#16809=CARTESIAN_POINT('Ctrl Pts',(10.0502525316942,-9.36936257048691,5.29266352931554));
#16810=CARTESIAN_POINT('',(10.0502525316942,-7.38503851882133,5.42237201204004));
#16811=CARTESIAN_POINT('Ctrl Pts',(10.0502525316942,-9.36936257048691,5.29266352931554));
#16812=CARTESIAN_POINT('Ctrl Pts',(10.0502525316942,-9.34434525366385,5.32181765856171));
#16813=CARTESIAN_POINT('Ctrl Pts',(10.0502525316942,-9.29515286061949,5.37803958295792));
#16814=CARTESIAN_POINT('Ctrl Pts',(10.0502525316942,-9.22389100140796,5.45611344595659));
#16815=CARTESIAN_POINT('Ctrl Pts',(10.0502525316942,-9.13393772674446,5.54767139923329));
#16816=CARTESIAN_POINT('Ctrl Pts',(10.0502525316942,-9.02993079896417,5.64122622022819));
#16817=CARTESIAN_POINT('Ctrl Pts',(10.0502525316942,-8.93425530662678,5.71414742300118));
#16818=CARTESIAN_POINT('Ctrl Pts',(10.0502525316942,-8.84663552299331,5.76712457531372));
#16819=CARTESIAN_POINT('Ctrl Pts',(10.0502525316942,-8.76653902495464,5.80148760154654));
#16820=CARTESIAN_POINT('Ctrl Pts',(10.0502525316942,-8.69311263972367,5.81936638407584));
#16821=CARTESIAN_POINT('Ctrl Pts',(10.0502525316942,-8.62505870129886,5.82399901560002));
#16822=CARTESIAN_POINT('Ctrl Pts',(10.0502525316942,-8.56077284249031,5.81938869186267));
#16823=CARTESIAN_POINT('Ctrl Pts',(10.0502525316942,-8.4986070414541,5.80964873807682));
#16824=CARTESIAN_POINT('Ctrl Pts',(10.0502525316942,-8.43709945169241,5.79843016859412));
#16825=CARTESIAN_POINT('Ctrl Pts',(10.0502525316942,-8.37520120352267,5.78835717995633));
#16826=CARTESIAN_POINT('Ctrl Pts',(10.0502525316942,-8.31255178250645,5.78034060190006));
#16827=CARTESIAN_POINT('Ctrl Pts',(10.0502525316942,-8.24933415385039,5.77394633717213));
#16828=CARTESIAN_POINT('Ctrl Pts',(10.0502525316942,-8.18604879427487,5.76796747841793));
#16829=CARTESIAN_POINT('Ctrl Pts',(10.0502525316942,-8.12332066784839,5.76091367696946));
#16830=CARTESIAN_POINT('Ctrl Pts',(10.0502525316942,-8.06168961610356,5.75154264947447));
#16831=CARTESIAN_POINT('Ctrl Pts',(10.0502525316942,-8.00141929583747,5.73934420595248));
#16832=CARTESIAN_POINT('Ctrl Pts',(10.0502525316942,-7.94258074919088,5.72431483522833));
#16833=CARTESIAN_POINT('Ctrl Pts',(10.0502525316942,-7.88512587067823,5.70675814390461));
#16834=CARTESIAN_POINT('Ctrl Pts',(10.0502525316942,-7.82895914189736,5.68709020402104));
#16835=CARTESIAN_POINT('Ctrl Pts',(10.0502525316942,-7.77401905533046,5.66561822174726));
#16836=CARTESIAN_POINT('Ctrl Pts',(10.0502525316942,-7.72032292706671,5.64241804293469));
#16837=CARTESIAN_POINT('Ctrl Pts',(10.0502525316942,-7.6679311867486,5.61742944592276));
#16838=CARTESIAN_POINT('Ctrl Pts',(10.0502525316942,-7.61692741952956,5.59050809253397));
#16839=CARTESIAN_POINT('Ctrl Pts',(10.0502525316942,-7.56739405041849,5.56148971316608));
#16840=CARTESIAN_POINT('Ctrl Pts',(10.0502525316942,-7.51938467268366,5.53026090613148));
#16841=CARTESIAN_POINT('Ctrl Pts',(10.0502525316942,-7.47292244003411,5.4967684895078));
#16842=CARTESIAN_POINT('Ctrl Pts',(10.0502525316942,-7.43699488267859,5.46814894648693));
#16843=CARTESIAN_POINT('Ctrl Pts',(10.0502525316942,-7.41074614986957,5.44565864507534));
#16844=CARTESIAN_POINT('Ctrl Pts',(10.0502525316942,-7.39355619607562,5.43021006317766));
#16845=CARTESIAN_POINT('Ctrl Pts',(10.0502525316942,-7.38503851882133,5.42237201204004));
#16846=CARTESIAN_POINT('',(10.0502525316942,-6.62239247796685,6.33125817110613));
#16847=CARTESIAN_POINT('Origin',(10.0502525316942,0.,0.));
#16848=CARTESIAN_POINT('',(10.0502525316942,-7.2752703501265,7.92891439885425));
#16849=CARTESIAN_POINT('Ctrl Pts',(10.0502525316942,-6.62239247796685,6.33125817110613));
#16850=CARTESIAN_POINT('Ctrl Pts',(10.0502525316942,-6.63100021625014,6.33803255463449));
#16851=CARTESIAN_POINT('Ctrl Pts',(10.0502525316942,-6.64806877891362,6.35173489391119));
#16852=CARTESIAN_POINT('Ctrl Pts',(10.0502525316942,-6.67323088220656,6.37274911883029));
#16853=CARTESIAN_POINT('Ctrl Pts',(10.0502525316942,-6.70589726716279,6.40169119143333));
#16854=CARTESIAN_POINT('Ctrl Pts',(10.0502525316942,-6.74524402479143,6.43941941070578));
#16855=CARTESIAN_POINT('Ctrl Pts',(10.0502525316942,-6.78307732500951,6.47871780200897));
#16856=CARTESIAN_POINT('Ctrl Pts',(10.0502525316942,-6.81935524839631,6.51961240030403));
#16857=CARTESIAN_POINT('Ctrl Pts',(10.0502525316942,-6.85401859544624,6.56213509649465));
#16858=CARTESIAN_POINT('Ctrl Pts',(10.0502525316942,-6.88699086799345,6.60632140469039));
#16859=CARTESIAN_POINT('Ctrl Pts',(10.0502525316942,-6.91819814506577,6.65219708634863));
#16860=CARTESIAN_POINT('Ctrl Pts',(10.0502525316942,-6.9475881722867,6.69976489037577));
#16861=CARTESIAN_POINT('Ctrl Pts',(10.0502525316942,-6.97514889902642,6.74899181640015));
#16862=CARTESIAN_POINT('Ctrl Pts',(10.0502525316942,-7.00093106972056,6.79979302943897));
#16863=CARTESIAN_POINT('Ctrl Pts',(10.0502525316942,-7.02506036068034,6.85202406661451));
#16864=CARTESIAN_POINT('Ctrl Pts',(10.0502525316942,-7.04770332746178,6.90550961656264));
#16865=CARTESIAN_POINT('Ctrl Pts',(10.0502525316942,-7.06903990194018,6.96006716732954));
#16866=CARTESIAN_POINT('Ctrl Pts',(10.0502525316942,-7.08923522069654,7.01553102941681));
#16867=CARTESIAN_POINT('Ctrl Pts',(10.0502525316942,-7.10840869098247,7.07177895456439));
#16868=CARTESIAN_POINT('Ctrl Pts',(10.0502525316942,-7.12661440941494,7.12874865657033));
#16869=CARTESIAN_POINT('Ctrl Pts',(10.0502525316942,-7.14386341521534,7.18641725377035));
#16870=CARTESIAN_POINT('Ctrl Pts',(10.0502525316942,-7.16013937508649,7.24478653536347));
#16871=CARTESIAN_POINT('Ctrl Pts',(10.0502525316942,-7.17541617812316,7.30386662226907));
#16872=CARTESIAN_POINT('Ctrl Pts',(10.0502525316942,-7.18967631564937,7.36365880682929));
#16873=CARTESIAN_POINT('Ctrl Pts',(10.0502525316942,-7.2029245901952,7.42414298774012));
#16874=CARTESIAN_POINT('Ctrl Pts',(10.0502525316942,-7.21517989232968,7.48528632500984));
#16875=CARTESIAN_POINT('Ctrl Pts',(10.0502525316942,-7.22647049097858,7.54704857406782));
#16876=CARTESIAN_POINT('Ctrl Pts',(10.0502525316942,-7.23682832548438,7.60938839179095));
#16877=CARTESIAN_POINT('Ctrl Pts',(10.0502525316942,-7.24628378544296,7.67226934177745));
#16878=CARTESIAN_POINT('Ctrl Pts',(10.0502525316942,-7.254861054624,7.73566511738401));
#16879=CARTESIAN_POINT('Ctrl Pts',(10.0502525316942,-7.26257856558425,7.79955765803962));
#16880=CARTESIAN_POINT('Ctrl Pts',(10.0502525316942,-7.26807493359233,7.85106030720964));
#16881=CARTESIAN_POINT('Ctrl Pts',(10.0502525316942,-7.27181932978281,7.88990344551799));
#16882=CARTESIAN_POINT('Ctrl Pts',(10.0502525316942,-7.27414795055897,7.91589476537953));
#16883=CARTESIAN_POINT('Ctrl Pts',(10.0502525316942,-7.2752703501265,7.92891439885425));
#16884=CARTESIAN_POINT('',(10.0502525316942,-5.34798390487229,7.43908464225652));
#16885=CARTESIAN_POINT('Ctrl Pts',(10.0502525316942,-7.2752703501265,7.92891439885425));
#16886=CARTESIAN_POINT('Ctrl Pts',(10.0502525316942,-7.24246834654844,7.94891084739874));
#16887=CARTESIAN_POINT('Ctrl Pts',(10.0502525316942,-7.17831007049656,7.98717978950973));
#16888=CARTESIAN_POINT('Ctrl Pts',(10.0502525316942,-7.08640986444703,8.03941132011984));
#16889=CARTESIAN_POINT('Ctrl Pts',(10.0502525316942,-6.97256625288353,8.09869101763159));
#16890=CARTESIAN_POINT('Ctrl Pts',(10.0502525316942,-6.84473975688512,8.15552703155277));
#16891=CARTESIAN_POINT('Ctrl Pts',(10.0502525316942,-6.73121306554078,8.19531386354866));
#16892=CARTESIAN_POINT('Ctrl Pts',(10.0502525316942,-6.63151085898163,8.21862212728407));
#16893=CARTESIAN_POINT('Ctrl Pts',(10.0502525316942,-6.54471580350543,8.22655212821855));
#16894=CARTESIAN_POINT('Ctrl Pts',(10.0502525316942,-6.46935831372324,8.22086585997457));
#16895=CARTESIAN_POINT('Ctrl Pts',(10.0502525316942,-6.40320361025513,8.20424193086582));
#16896=CARTESIAN_POINT('Ctrl Pts',(10.0502525316942,-6.34348879371404,8.17999182956336));
#16897=CARTESIAN_POINT('Ctrl Pts',(10.0502525316942,-6.2873754147921,8.15151829405778));
#16898=CARTESIAN_POINT('Ctrl Pts',(10.0502525316942,-6.23234494937036,8.12184190992835));
#16899=CARTESIAN_POINT('Ctrl Pts',(10.0502525316942,-6.1765889417745,8.09313431783932));
#16900=CARTESIAN_POINT('Ctrl Pts',(10.0502525316942,-6.11948306053102,8.06615036325875));
#16901=CARTESIAN_POINT('Ctrl Pts',(10.0502525316942,-6.06133545932041,8.04053373452353));
#16902=CARTESIAN_POINT('Ctrl Pts',(10.0502525316942,-6.00299507467205,8.01529125034138));
#16903=CARTESIAN_POINT('Ctrl Pts',(10.0502525316942,-5.94551682580168,7.98919862941808));
#16904=CARTESIAN_POINT('Ctrl Pts',(10.0502525316942,-5.88979801918435,7.96124121028423));
#16905=CARTESIAN_POINT('Ctrl Pts',(10.0502525316942,-5.83624706470931,7.93101524786534));
#16906=CARTESIAN_POINT('Ctrl Pts',(10.0502525316942,-5.78493261248025,7.89853935606421));
#16907=CARTESIAN_POINT('Ctrl Pts',(10.0502525316942,-5.73571509186187,7.86408741650604));
#16908=CARTESIAN_POINT('Ctrl Pts',(10.0502525316942,-5.68837508612421,7.82802562040593));
#16909=CARTESIAN_POINT('Ctrl Pts',(10.0502525316942,-5.64275916621446,7.79062713132508));
#16910=CARTESIAN_POINT('Ctrl Pts',(10.0502525316942,-5.59886036305501,7.75196943392054));
#16911=CARTESIAN_POINT('Ctrl Pts',(10.0502525316942,-5.55675475816771,7.71201392777609));
#16912=CARTESIAN_POINT('Ctrl Pts',(10.0502525316942,-5.51656644870715,7.67064916836037));
#16913=CARTESIAN_POINT('Ctrl Pts',(10.0502525316942,-5.47842458761391,7.62774439672625));
#16914=CARTESIAN_POINT('Ctrl Pts',(10.0502525316942,-5.44241518816367,7.58320832269043));
#16915=CARTESIAN_POINT('Ctrl Pts',(10.0502525316942,-5.4085767049601,7.5369975221287));
#16916=CARTESIAN_POINT('Ctrl Pts',(10.0502525316942,-5.38325149258725,7.49867649345608));
#16917=CARTESIAN_POINT('Ctrl Pts',(10.0502525316942,-5.36523734954955,7.46917564122634));
#16918=CARTESIAN_POINT('Ctrl Pts',(10.0502525316942,-5.35366260632437,7.44917117889019));
#16919=CARTESIAN_POINT('Ctrl Pts',(10.0502525316942,-5.34798390487229,7.43908464225652));
#16920=CARTESIAN_POINT('',(10.0502525316942,-4.34180314898733,8.06781615908999));
#16921=CARTESIAN_POINT('Origin',(10.0502525316942,0.,0.));
#16922=CARTESIAN_POINT('',(10.0502525316942,-4.46902397810655,9.78902788303806));
#16923=CARTESIAN_POINT('Ctrl Pts',(10.0502525316942,-4.34180314898733,8.06781615908999));
#16924=CARTESIAN_POINT('Ctrl Pts',(10.0502525316942,-4.34789619493555,8.07691891810119));
#16925=CARTESIAN_POINT('Ctrl Pts',(10.0502525316942,-4.35989510698125,8.09522509309135));
#16926=CARTESIAN_POINT('Ctrl Pts',(10.0502525316942,-4.37733193665808,8.1229863261673));
#16927=CARTESIAN_POINT('Ctrl Pts',(10.0502525316942,-4.39945592264773,8.16060634100777));
#16928=CARTESIAN_POINT('Ctrl Pts',(10.0502525316942,-4.42521825196285,8.20864682657585));
#16929=CARTESIAN_POINT('Ctrl Pts',(10.0502525316942,-4.44905598790391,8.25771295042534));
#16930=CARTESIAN_POINT('Ctrl Pts',(10.0502525316942,-4.47092121748728,8.30781651946229));
#16931=CARTESIAN_POINT('Ctrl Pts',(10.0502525316942,-4.49074778380617,8.35896957008516));
#16932=CARTESIAN_POINT('Ctrl Pts',(10.0502525316942,-4.50845195831808,8.41118223898599));
#16933=CARTESIAN_POINT('Ctrl Pts',(10.0502525316942,-4.52395547727261,8.46445618393006));
#16934=CARTESIAN_POINT('Ctrl Pts',(10.0502525316942,-4.53720779434568,8.51877787179233));
#16935=CARTESIAN_POINT('Ctrl Pts',(10.0502525316942,-4.54820764638295,8.5741121935049));
#16936=CARTESIAN_POINT('Ctrl Pts',(10.0502525316942,-4.55702950966199,8.63039414709753));
#16937=CARTESIAN_POINT('Ctrl Pts',(10.0502525316942,-4.5638375509418,8.68752517632497));
#16938=CARTESIAN_POINT('Ctrl Pts',(10.0502525316942,-4.56884434816008,8.7453900186693));
#16939=CARTESIAN_POINT('Ctrl Pts',(10.0502525316942,-4.57227742599473,8.80387069695484));
#16940=CARTESIAN_POINT('Ctrl Pts',(10.0502525316942,-4.57434503953799,8.86286066111437));
#16941=CARTESIAN_POINT('Ctrl Pts',(10.0502525316942,-4.57519852862449,8.92228054501355));
#16942=CARTESIAN_POINT('Ctrl Pts',(10.0502525316942,-4.57490858968921,8.98208782772813));
#16943=CARTESIAN_POINT('Ctrl Pts',(10.0502525316942,-4.57349279247872,9.0422641588092));
#16944=CARTESIAN_POINT('Ctrl Pts',(10.0502525316942,-4.57093505021141,9.10280619261976));
#16945=CARTESIAN_POINT('Ctrl Pts',(10.0502525316942,-4.56720740240461,9.16371548601266));
#16946=CARTESIAN_POINT('Ctrl Pts',(10.0502525316942,-4.56229279796226,9.22498785759991));
#16947=CARTESIAN_POINT('Ctrl Pts',(10.0502525316942,-4.55620201600645,9.28660567396873));
#16948=CARTESIAN_POINT('Ctrl Pts',(10.0502525316942,-4.54896317065147,9.34854353993788));
#16949=CARTESIAN_POINT('Ctrl Pts',(10.0502525316942,-4.54061558349964,9.4107719162247));
#16950=CARTESIAN_POINT('Ctrl Pts',(10.0502525316942,-4.53120240639841,9.47326135298215));
#16951=CARTESIAN_POINT('Ctrl Pts',(10.0502525316942,-4.52076380103831,9.53598658803447));
#16952=CARTESIAN_POINT('Ctrl Pts',(10.0502525316942,-4.50933089675096,9.59893007547295));
#16953=CARTESIAN_POINT('Ctrl Pts',(10.0502525316942,-4.4969268049629,9.6620803346471));
#16954=CARTESIAN_POINT('Ctrl Pts',(10.0502525316942,-4.48623896772408,9.71276073586856));
#16955=CARTESIAN_POINT('Ctrl Pts',(10.0502525316942,-4.47779691026848,9.7508598377266));
#16956=CARTESIAN_POINT('Ctrl Pts',(10.0502525316942,-4.47197980068818,9.77629863524131));
#16957=CARTESIAN_POINT('Ctrl Pts',(10.0502525316942,-4.46902397810655,9.78902788303806));
#16958=CARTESIAN_POINT('',(10.0502525316942,-2.78743136471945,8.7276078365385));
#16959=CARTESIAN_POINT('Ctrl Pts',(10.0502525316942,-4.46902397810655,9.78902788303806));
#16960=CARTESIAN_POINT('Ctrl Pts',(10.0502525316942,-4.4316481764287,9.7979092591739));
#16961=CARTESIAN_POINT('Ctrl Pts',(10.0502525316942,-4.35880427644625,9.81447918831044));
#16962=CARTESIAN_POINT('Ctrl Pts',(10.0502525316942,-4.25526155603325,9.83575560039739));
#16963=CARTESIAN_POINT('Ctrl Pts',(10.0502525316942,-4.12867141346467,9.85695433232581));
#16964=CARTESIAN_POINT('Ctrl Pts',(10.0502525316942,-3.98953789729602,9.87150803413088));
#16965=CARTESIAN_POINT('Ctrl Pts',(10.0502525316942,-3.86927279048049,9.87426588302275));
#16966=CARTESIAN_POINT('Ctrl Pts',(10.0502525316942,-3.76724770763979,9.86562368292838));
#16967=CARTESIAN_POINT('Ctrl Pts',(10.0502525316942,-3.68225019949279,9.84634441482148));
#16968=CARTESIAN_POINT('Ctrl Pts',(10.0502525316942,-3.61233812130575,9.81764970735851));
#16969=CARTESIAN_POINT('Ctrl Pts',(10.0502525316942,-3.55455833609672,9.78139648362373));
#16970=CARTESIAN_POINT('Ctrl Pts',(10.0502525316942,-3.50525986412372,9.73988037363202));
#16971=CARTESIAN_POINT('Ctrl Pts',(10.0502525316942,-3.46069167580983,9.6954604444488));
#16972=CARTESIAN_POINT('Ctrl Pts',(10.0502525316942,-3.41752510010333,9.65023117691875));
#16973=CARTESIAN_POINT('Ctrl Pts',(10.0502525316942,-3.37336911957978,9.60569908050971));
#16974=CARTESIAN_POINT('Ctrl Pts',(10.0502525316942,-3.32739669964523,9.56238912688746));
#16975=CARTESIAN_POINT('Ctrl Pts',(10.0502525316942,-3.28001101822472,9.5200576682471));
#16976=CARTESIAN_POINT('Ctrl Pts',(10.0502525316942,-3.23232637183425,9.47802246886347));
#16977=CARTESIAN_POINT('Ctrl Pts',(10.0502525316942,-3.18572437199394,9.43544515599928));
#16978=CARTESIAN_POINT('Ctrl Pts',(10.0502525316942,-3.14137195551156,9.3916380122022));
#16979=CARTESIAN_POINT('Ctrl Pts',(10.0502525316942,-3.09978230736302,9.34634325868463));
#16980=CARTESIAN_POINT('Ctrl Pts',(10.0502525316942,-3.06101496566449,9.29959981236885));
#16981=CARTESIAN_POINT('Ctrl Pts',(10.0502525316942,-3.02485255677714,9.25162502046097));
#16982=CARTESIAN_POINT('Ctrl Pts',(10.0502525316942,-2.99097324368151,9.20269934800391));
#16983=CARTESIAN_POINT('Ctrl Pts',(10.0502525316942,-2.95914669449447,9.15303517679781));
#16984=CARTESIAN_POINT('Ctrl Pts',(10.0502525316942,-2.92934233715353,9.10270404556727));
#16985=CARTESIAN_POINT('Ctrl Pts',(10.0502525316942,-2.9016444576704,9.05169275361811));
#16986=CARTESIAN_POINT('Ctrl Pts',(10.0502525316942,-2.87620551770673,8.99993365903229));
#16987=CARTESIAN_POINT('Ctrl Pts',(10.0502525316942,-2.85318875574511,8.94734231311461));
#16988=CARTESIAN_POINT('Ctrl Pts',(10.0502525316942,-2.83270418548989,8.89385847330528));
#16989=CARTESIAN_POINT('Ctrl Pts',(10.0502525316942,-2.81480179823484,8.83945272393405));
#16990=CARTESIAN_POINT('Ctrl Pts',(10.0502525316942,-2.80255793908285,8.79518133889446));
#16991=CARTESIAN_POINT('Ctrl Pts',(10.0502525316942,-2.7945417356489,8.76155768480736));
#16992=CARTESIAN_POINT('Ctrl Pts',(10.0502525316942,-2.78971521950536,8.73895551818547));
#16993=CARTESIAN_POINT('Ctrl Pts',(10.0502525316942,-2.78743136471945,8.7276078365385));
#16994=CARTESIAN_POINT('',(10.0502525316942,-1.6362078766636,9.01464008964162));
#16995=CARTESIAN_POINT('Origin',(10.0502525316942,0.,0.));
#16996=CARTESIAN_POINT('',(10.0502525316942,-1.22531840158854,10.6909231138624));
#16997=CARTESIAN_POINT('Ctrl Pts',(10.0502525316942,-1.6362078766636,9.01464008964162));
#16998=CARTESIAN_POINT('Ctrl Pts',(10.0502525316942,-1.63918980048658,9.02518018266099));
#16999=CARTESIAN_POINT('Ctrl Pts',(10.0502525316942,-1.64494452480213,9.04629825740996));
#17000=CARTESIAN_POINT('Ctrl Pts',(10.0502525316942,-1.65294924248453,9.07808903572539));
#17001=CARTESIAN_POINT('Ctrl Pts',(10.0502525316942,-1.66236517961207,9.12070448363665));
#17002=CARTESIAN_POINT('Ctrl Pts',(10.0502525316942,-1.67202128432359,9.17435469805521));
#17003=CARTESIAN_POINT('Ctrl Pts',(10.0502525316942,-1.67953005230647,9.22838562038483));
#17004=CARTESIAN_POINT('Ctrl Pts',(10.0502525316942,-1.68484226707077,9.28279367373423));
#17005=CARTESIAN_POINT('Ctrl Pts',(10.0502525316942,-1.68789129020751,9.33756986179013));
#17006=CARTESIAN_POINT('Ctrl Pts',(10.0502525316942,-1.68859435873067,9.39269795157698));
#17007=CARTESIAN_POINT('Ctrl Pts',(10.0502525316942,-1.68687652711276,9.44815533489435));
#17008=CARTESIAN_POINT('Ctrl Pts',(10.0502525316942,-1.68269390490855,9.50391352130234));
#17009=CARTESIAN_POINT('Ctrl Pts',(10.0502525316942,-1.67605614008548,9.55993872975698));
#17010=CARTESIAN_POINT('Ctrl Pts',(10.0502525316942,-1.66705415050613,9.61619215414635));
#17011=CARTESIAN_POINT('Ctrl Pts',(10.0502525316942,-1.65587452359108,9.67263079222962));
#17012=CARTESIAN_POINT('Ctrl Pts',(10.0502525316942,-1.64275505105007,9.72921071303343));
#17013=CARTESIAN_POINT('Ctrl Pts',(10.0502525316942,-1.62794857866286,9.78589002258816));
#17014=CARTESIAN_POINT('Ctrl Pts',(10.0502525316942,-1.6116860945735,9.84263174012077));
#17015=CARTESIAN_POINT('Ctrl Pts',(10.0502525316942,-1.59413605700216,9.89940715053283));
#17016=CARTESIAN_POINT('Ctrl Pts',(10.0502525316942,-1.57537884194225,9.9561976604221));
#17017=CARTESIAN_POINT('Ctrl Pts',(10.0502525316942,-1.55543682981628,10.0129912468249));
#17018=CARTESIAN_POINT('Ctrl Pts',(10.0502525316942,-1.53429575504446,10.0697797567623));
#17019=CARTESIAN_POINT('Ctrl Pts',(10.0502525316942,-1.51192854453357,10.1265560306252));
#17020=CARTESIAN_POINT('Ctrl Pts',(10.0502525316942,-1.48832027384755,10.1833108225988));
#17021=CARTESIAN_POINT('Ctrl Pts',(10.0502525316942,-1.4634866435649,10.2400306932429));
#17022=CARTESIAN_POINT('Ctrl Pts',(10.0502525316942,-1.43746223933981,10.2967001780439));
#17023=CARTESIAN_POINT('Ctrl Pts',(10.0502525316942,-1.41029358637874,10.353303334518));
#17024=CARTESIAN_POINT('Ctrl Pts',(10.0502525316942,-1.38203082503059,10.4098254888505));
#17025=CARTESIAN_POINT('Ctrl Pts',(10.0502525316942,-1.35271995777451,10.4662550259293));
#17026=CARTESIAN_POINT('Ctrl Pts',(10.0502525316942,-1.32239601234813,10.5225848780961));
#17027=CARTESIAN_POINT('Ctrl Pts',(10.0502525316942,-1.29108451674038,10.5788112684272));
#17028=CARTESIAN_POINT('Ctrl Pts',(10.0502525316942,-1.26525867423012,10.6237084709174));
#17029=CARTESIAN_POINT('Ctrl Pts',(10.0502525316942,-1.24545653053149,10.6573341307832));
#17030=CARTESIAN_POINT('Ctrl Pts',(10.0502525316942,-1.23206310981063,10.6797302792078));
#17031=CARTESIAN_POINT('Ctrl Pts',(10.0502525316942,-1.22531840158854,10.6909231138624));
#17032=CARTESIAN_POINT('',(10.0502525316942,0.0459743785884363,9.16181196696065));
#17033=CARTESIAN_POINT('Ctrl Pts',(10.0502525316942,-1.22531840158854,10.6909231138624));
#17034=CARTESIAN_POINT('Ctrl Pts',(10.0502525316942,-1.18702740569167,10.6878200466132));
#17035=CARTESIAN_POINT('Ctrl Pts',(10.0502525316942,-1.11262835024222,10.6810689826619));
#17036=CARTESIAN_POINT('Ctrl Pts',(10.0502525316942,-1.00757859836431,10.6693075927691));
#17037=CARTESIAN_POINT('Ctrl Pts',(10.0502525316942,-0.880633449950656,
10.6503502795328));
#17038=CARTESIAN_POINT('Ctrl Pts',(10.0502525316942,-0.743812271574575,
10.6211970514875));
#17039=CARTESIAN_POINT('Ctrl Pts',(10.0502525316942,-0.628581135879225,
10.5866559598108));
#17040=CARTESIAN_POINT('Ctrl Pts',(10.0502525316942,-0.534220102715977,
10.5469092546456));
#17041=CARTESIAN_POINT('Ctrl Pts',(10.0502525316942,-0.459340290208066,
10.5023079065862));
#17042=CARTESIAN_POINT('Ctrl Pts',(10.0502525316942,-0.40171710493522,10.4534135977985));
#17043=CARTESIAN_POINT('Ctrl Pts',(10.0502525316942,-0.357968125936963,
10.4010797975679));
#17044=CARTESIAN_POINT('Ctrl Pts',(10.0502525316942,-0.323911676451425,
10.3463615649927));
#17045=CARTESIAN_POINT('Ctrl Pts',(10.0502525316942,-0.295251323542575,
10.2903433742921));
#17046=CARTESIAN_POINT('Ctrl Pts',(10.0502525316942,-0.268174082740675,
10.2339885791981));
#17047=CARTESIAN_POINT('Ctrl Pts',(10.0502525316942,-0.239940424315884,
10.1779910903389));
#17048=CARTESIAN_POINT('Ctrl Pts',(10.0502525316942,-0.209601566462141,
10.1225946176937));
#17049=CARTESIAN_POINT('Ctrl Pts',(10.0502525316942,-0.177616245484635,
10.0676920272606));
#17050=CARTESIAN_POINT('Ctrl Pts',(10.0502525316942,-0.145255042779231,
10.0129788108676));
#17051=CARTESIAN_POINT('Ctrl Pts',(10.0502525316942,-0.114091020408569,
9.95808457009925));
#17052=CARTESIAN_POINT('Ctrl Pts',(10.0502525316942,-0.0854465176078901,
9.90271585009609));
#17053=CARTESIAN_POINT('Ctrl Pts',(10.0502525316942,-0.0598892603187496,
9.84678607154126));
#17054=CARTESIAN_POINT('Ctrl Pts',(10.0502525316942,-0.0374638466641566,
9.79035064491696));
#17055=CARTESIAN_POINT('Ctrl Pts',(10.0502525316942,-0.0178963780480504,
9.73354910755133));
#17056=CARTESIAN_POINT('Ctrl Pts',(10.0502525316942,-0.000794100811299239,
9.67654874444263));
#17057=CARTESIAN_POINT('Ctrl Pts',(10.0502525316942,0.0141276732699908,
9.61948036621956));
#17058=CARTESIAN_POINT('Ctrl Pts',(10.0502525316942,0.0269201266367293,
9.56240256296547));
#17059=CARTESIAN_POINT('Ctrl Pts',(10.0502525316942,0.0374990192894122,
9.50532882588415));
#17060=CARTESIAN_POINT('Ctrl Pts',(10.0502525316942,0.045698449069018,9.44824193693312));
#17061=CARTESIAN_POINT('Ctrl Pts',(10.0502525316942,0.0513370708710183,
9.39111202409575));
#17062=CARTESIAN_POINT('Ctrl Pts',(10.0502525316942,0.0542916394702422,
9.33391578939727));
#17063=CARTESIAN_POINT('Ctrl Pts',(10.0502525316942,0.0545055203789821,
9.27664070503215));
#17064=CARTESIAN_POINT('Ctrl Pts',(10.0502525316942,0.0524695120683291,
9.23075255525014));
#17065=CARTESIAN_POINT('Ctrl Pts',(10.0502525316942,0.0497030940542384,
9.19629741683749));
#17066=CARTESIAN_POINT('Ctrl Pts',(10.0502525316942,0.0473089300876993,
9.17331000347738));
#17067=CARTESIAN_POINT('Ctrl Pts',(10.0502525316942,0.0459743785884363,
9.16181196696065));
#17068=CARTESIAN_POINT('',(10.0502525316942,1.22955082275859,9.07904823952839));
#17069=CARTESIAN_POINT('Origin',(10.0502525316942,0.,0.));
#17070=CARTESIAN_POINT('',(10.0502525316942,2.13832987737225,10.5463163022605));
#17071=CARTESIAN_POINT('Ctrl Pts',(10.0502525316942,1.22955082275859,9.07904823952839));
#17072=CARTESIAN_POINT('Ctrl Pts',(10.0502525316942,1.22997191254093,9.08999392881406));
#17073=CARTESIAN_POINT('Ctrl Pts',(10.0502525316942,1.23102468846705,9.11185671902711));
#17074=CARTESIAN_POINT('Ctrl Pts',(10.0502525316942,1.23323564031797,9.14456513970113));
#17075=CARTESIAN_POINT('Ctrl Pts',(10.0502525316942,1.23744944958329,9.18800452372235));
#17076=CARTESIAN_POINT('Ctrl Pts',(10.0502525316942,1.24484477628256,9.24201281020108));
#17077=CARTESIAN_POINT('Ctrl Pts',(10.0502525316942,1.2543999867847,9.29571960787763));
#17078=CARTESIAN_POINT('Ctrl Pts',(10.0502525316942,1.26616078343298,9.34910630619445));
#17079=CARTESIAN_POINT('Ctrl Pts',(10.0502525316942,1.28018776310679,9.40214375674832));
#17080=CARTESIAN_POINT('Ctrl Pts',(10.0502525316942,1.29655462181801,9.45479094589287));
#17081=CARTESIAN_POINT('Ctrl Pts',(10.0502525316942,1.31532565068075,9.50700321251013));
#17082=CARTESIAN_POINT('Ctrl Pts',(10.0502525316942,1.33653378795886,9.55873989768809));
#17083=CARTESIAN_POINT('Ctrl Pts',(10.0502525316942,1.36015941897336,9.60997185513068));
#17084=CARTESIAN_POINT('Ctrl Pts',(10.0502525316942,1.38610408395052,9.6606902731969));
#17085=CARTESIAN_POINT('Ctrl Pts',(10.0502525316942,1.41417703928493,9.7109119130093));
#17086=CARTESIAN_POINT('Ctrl Pts',(10.0502525316942,1.44413855620418,9.76066847540881));
#17087=CARTESIAN_POINT('Ctrl Pts',(10.0502525316942,1.47573521813323,9.80999825050557));
#17088=CARTESIAN_POINT('Ctrl Pts',(10.0502525316942,1.50873591460517,9.85893744675637));
#17089=CARTESIAN_POINT('Ctrl Pts',(10.0502525316942,1.54297155887855,9.90751081093262));
#17090=CARTESIAN_POINT('Ctrl Pts',(10.0502525316942,1.57835996316383,9.95572549720588));
#17091=CARTESIAN_POINT('Ctrl Pts',(10.0502525316942,1.61487612711423,10.003576986989));
#17092=CARTESIAN_POINT('Ctrl Pts',(10.0502525316942,1.65253109869336,10.0510531180319));
#17093=CARTESIAN_POINT('Ctrl Pts',(10.0502525316942,1.69134841350201,10.0981387150956));
#17094=CARTESIAN_POINT('Ctrl Pts',(10.0502525316942,1.73133940840846,10.1448203729832));
#17095=CARTESIAN_POINT('Ctrl Pts',(10.0502525316942,1.77248499825981,10.1910901617733));
#17096=CARTESIAN_POINT('Ctrl Pts',(10.0502525316942,1.81474751134677,10.2369440613944));
#17097=CARTESIAN_POINT('Ctrl Pts',(10.0502525316942,1.85807777307013,10.2823812867227));
#17098=CARTESIAN_POINT('Ctrl Pts',(10.0502525316942,1.90242356266618,10.3274033763511));
#17099=CARTESIAN_POINT('Ctrl Pts',(10.0502525316942,1.94773753991041,10.3720134991994));
#17100=CARTESIAN_POINT('Ctrl Pts',(10.0502525316942,1.99398420741813,10.4162157576914));
#17101=CARTESIAN_POINT('Ctrl Pts',(10.0502525316942,2.04113811949547,10.4600144483414));
#17102=CARTESIAN_POINT('Ctrl Pts',(10.0502525316942,2.07957395387303,10.4947336011034));
#17103=CARTESIAN_POINT('Ctrl Pts',(10.0502525316942,2.10879781201984,10.5205943051056));
#17104=CARTESIAN_POINT('Ctrl Pts',(10.0502525316942,2.12845650254365,10.5377555133892));
#17105=CARTESIAN_POINT('Ctrl Pts',(10.0502525316942,2.13832987737225,10.5463163022605));
#17106=CARTESIAN_POINT('',(10.0502525316942,2.87487982939776,8.69919410795919));
#17107=CARTESIAN_POINT('Ctrl Pts',(10.0502525316942,2.13832987737225,10.5463163022605));
#17108=CARTESIAN_POINT('Ctrl Pts',(10.0502525316942,2.17378787802072,10.531532541469));
#17109=CARTESIAN_POINT('Ctrl Pts',(10.0502525316942,2.24245939102107,10.5021213256069));
#17110=CARTESIAN_POINT('Ctrl Pts',(10.0502525316942,2.33873317272541,10.4584734205235));
#17111=CARTESIAN_POINT('Ctrl Pts',(10.0502525316942,2.45360705137856,10.4012157360254));
#17112=CARTESIAN_POINT('Ctrl Pts',(10.0502525316942,2.57472288173342,10.3312092992132));
#17113=CARTESIAN_POINT('Ctrl Pts',(10.0502525316942,2.6736404198842,10.2627503896831));
#17114=CARTESIAN_POINT('Ctrl Pts',(10.0502525316942,2.751100687992,10.1957898638803));
#17115=CARTESIAN_POINT('Ctrl Pts',(10.0502525316942,2.80853304709422,10.1302323265723));
#17116=CARTESIAN_POINT('Ctrl Pts',(10.0502525316942,2.84822678059402,10.0659245320707));
#17117=CARTESIAN_POINT('Ctrl Pts',(10.0502525316942,2.8736624985001,10.0026329523419));
#17118=CARTESIAN_POINT('Ctrl Pts',(10.0502525316942,2.88914324293729,9.94006879903196));
#17119=CARTESIAN_POINT('Ctrl Pts',(10.0502525316942,2.89909028540996,9.8779357976215));
#17120=CARTESIAN_POINT('Ctrl Pts',(10.0502525316942,2.90742768231934,9.81597187495431));
#17121=CARTESIAN_POINT('Ctrl Pts',(10.0502525316942,2.91697531144329,9.753990418012));
#17122=CARTESIAN_POINT('Ctrl Pts',(10.0502525316942,2.92871082842625,9.69193001905628));
#17123=CARTESIAN_POINT('Ctrl Pts',(10.0502525316942,2.94216484288864,9.62983054491075));
#17124=CARTESIAN_POINT('Ctrl Pts',(10.0502525316942,2.95603486191442,9.56779502233836));
#17125=CARTESIAN_POINT('Ctrl Pts',(10.0502525316942,2.96871035517328,9.50595728442294));
#17126=CARTESIAN_POINT('Ctrl Pts',(10.0502525316942,2.97884302078013,9.44444686430419));
#17127=CARTESIAN_POINT('Ctrl Pts',(10.0502525316942,2.98586616479853,9.38335685712271));
#17128=CARTESIAN_POINT('Ctrl Pts',(10.0502525316942,2.98975449467364,9.32275374295661));
#17129=CARTESIAN_POINT('Ctrl Pts',(10.0502525316942,2.99081162285579,9.26268559037018));
#17130=CARTESIAN_POINT('Ctrl Pts',(10.0502525316942,2.98946277417915,9.20319012929579));
#17131=CARTESIAN_POINT('Ctrl Pts',(10.0502525316942,2.9860191259415,9.144303794535));
#17132=CARTESIAN_POINT('Ctrl Pts',(10.0502525316942,2.98054746086824,9.08606649232432));
#17133=CARTESIAN_POINT('Ctrl Pts',(10.0502525316942,2.97297183097014,9.02851708515246));
#17134=CARTESIAN_POINT('Ctrl Pts',(10.0502525316942,2.96312913325008,8.97169046427448));
#17135=CARTESIAN_POINT('Ctrl Pts',(10.0502525316942,2.95083766730388,8.91561425843345));
#17136=CARTESIAN_POINT('Ctrl Pts',(10.0502525316942,2.93597302048693,8.86030439480771));
#17137=CARTESIAN_POINT('Ctrl Pts',(10.0502525316942,2.91847745889582,8.80576645976534));
#17138=CARTESIAN_POINT('Ctrl Pts',(10.0502525316942,2.90236088180168,8.76275339706311));
#17139=CARTESIAN_POINT('Ctrl Pts',(10.0502525316942,2.88908263860953,8.7308394833358));
#17140=CARTESIAN_POINT('Ctrl Pts',(10.0502525316942,2.87970215198308,8.70971699141988));
#17141=CARTESIAN_POINT('Ctrl Pts',(10.0502525316942,2.87487982939776,8.69919410795919));
#17142=CARTESIAN_POINT('',(10.0502525316942,3.97495252086484,8.25473589028142));
#17143=CARTESIAN_POINT('Origin',(10.0502525316942,0.,0.));
#17144=CARTESIAN_POINT('',(10.0502525316942,5.29266352931554,9.36936257048691));
#17145=CARTESIAN_POINT('Ctrl Pts',(10.0502525316942,3.97495252086484,8.25473589028142));
#17146=CARTESIAN_POINT('Ctrl Pts',(10.0502525316942,3.9787354050507,8.26501573550299));
#17147=CARTESIAN_POINT('Ctrl Pts',(10.0502525316942,3.98649262817573,8.28548315894707));
#17148=CARTESIAN_POINT('Ctrl Pts',(10.0502525316942,3.9987028261882,8.31590749387114));
#17149=CARTESIAN_POINT('Ctrl Pts',(10.0502525316942,4.01613390483614,8.35591866443433));
#17150=CARTESIAN_POINT('Ctrl Pts',(10.0502525316942,4.03985675684261,8.40499831559484));
#17151=CARTESIAN_POINT('Ctrl Pts',(10.0502525316942,4.06554061525075,8.45312379306447));
#17152=CARTESIAN_POINT('Ctrl Pts',(10.0502525316942,4.09322319459338,8.50026327435046));
#17153=CARTESIAN_POINT('Ctrl Pts',(10.0502525316942,4.12295311857557,8.54637031220843));
#17154=CARTESIAN_POINT('Ctrl Pts',(10.0502525316942,4.1547878023559,8.59138312702269));
#17155=CARTESIAN_POINT('Ctrl Pts',(10.0502525316942,4.18877458937293,8.63523937649908));
#17156=CARTESIAN_POINT('Ctrl Pts',(10.0502525316942,4.22493224148239,8.67789021323112));
#17157=CARTESIAN_POINT('Ctrl Pts',(10.0502525316942,4.26323309731516,8.71931397871314));
#17158=CARTESIAN_POINT('Ctrl Pts',(10.0502525316942,4.30358079311506,8.75953271831989));
#17159=CARTESIAN_POINT('Ctrl Pts',(10.0502525316942,4.34579910040492,8.79862131584184));
#17160=CARTESIAN_POINT('Ctrl Pts',(10.0502525316942,4.38966981967219,8.83668400083504));
#17161=CARTESIAN_POINT('Ctrl Pts',(10.0502525316942,4.43496376972658,8.87383549938659));
#17162=CARTESIAN_POINT('Ctrl Pts',(10.0502525316942,4.48147234048104,8.91018166484712));
#17163=CARTESIAN_POINT('Ctrl Pts',(10.0502525316942,4.52904236806123,8.94579828347148));
#17164=CARTESIAN_POINT('Ctrl Pts',(10.0502525316942,4.57759789799493,8.98071755670482));
#17165=CARTESIAN_POINT('Ctrl Pts',(10.0502525316942,4.62711375721922,9.01494291264748));
#17166=CARTESIAN_POINT('Ctrl Pts',(10.0502525316942,4.67759669462988,9.04845937030362));
#17167=CARTESIAN_POINT('Ctrl Pts',(10.0502525316942,4.72906440450668,9.08124522426278));
#17168=CARTESIAN_POINT('Ctrl Pts',(10.0502525316942,4.78152352641848,9.11328422214026));
#17169=CARTESIAN_POINT('Ctrl Pts',(10.0502525316942,4.83495345882569,9.14457471976904));
#17170=CARTESIAN_POINT('Ctrl Pts',(10.0502525316942,4.88931713153333,9.17512453503235));
#17171=CARTESIAN_POINT('Ctrl Pts',(10.0502525316942,4.94456753410179,9.20494811701998));
#17172=CARTESIAN_POINT('Ctrl Pts',(10.0502525316942,5.00065547708482,9.23406306612412));
#17173=CARTESIAN_POINT('Ctrl Pts',(10.0502525316942,5.05753691650348,9.26248702510056));
#17174=CARTESIAN_POINT('Ctrl Pts',(10.0502525316942,5.11517936005741,9.29023486488122));
#17175=CARTESIAN_POINT('Ctrl Pts',(10.0502525316942,5.17355993514958,9.31731853484592));
#17176=CARTESIAN_POINT('Ctrl Pts',(10.0502525316942,5.22084339412736,9.33846108530483));
#17177=CARTESIAN_POINT('Ctrl Pts',(10.0502525316942,5.25662833187234,9.35402540755351));
#17178=CARTESIAN_POINT('Ctrl Pts',(10.0502525316942,5.28062796260048,9.3642718170601));
#17179=CARTESIAN_POINT('Ctrl Pts',(10.0502525316942,5.29266352931554,9.36936257048691));
#17180=CARTESIAN_POINT('',(10.0502525316942,5.42237201204004,7.38503851882133));
#17181=CARTESIAN_POINT('Ctrl Pts',(10.0502525316942,5.29266352931554,9.36936257048691));
#17182=CARTESIAN_POINT('Ctrl Pts',(10.0502525316942,5.32181765856171,9.34434525366385));
#17183=CARTESIAN_POINT('Ctrl Pts',(10.0502525316942,5.37803958295792,9.29515286061949));
#17184=CARTESIAN_POINT('Ctrl Pts',(10.0502525316942,5.45611344595659,9.22389100140797));
#17185=CARTESIAN_POINT('Ctrl Pts',(10.0502525316942,5.54767139923329,9.13393772674446));
#17186=CARTESIAN_POINT('Ctrl Pts',(10.0502525316942,5.64122622022818,9.02993079896417));
#17187=CARTESIAN_POINT('Ctrl Pts',(10.0502525316942,5.71414742300118,8.93425530662678));
#17188=CARTESIAN_POINT('Ctrl Pts',(10.0502525316942,5.76712457531372,8.84663552299331));
#17189=CARTESIAN_POINT('Ctrl Pts',(10.0502525316942,5.80148760154654,8.76653902495464));
#17190=CARTESIAN_POINT('Ctrl Pts',(10.0502525316942,5.81936638407584,8.69311263972367));
#17191=CARTESIAN_POINT('Ctrl Pts',(10.0502525316942,5.82399901560002,8.62505870129887));
#17192=CARTESIAN_POINT('Ctrl Pts',(10.0502525316942,5.81938869186267,8.56077284249031));
#17193=CARTESIAN_POINT('Ctrl Pts',(10.0502525316942,5.80964873807682,8.4986070414541));
#17194=CARTESIAN_POINT('Ctrl Pts',(10.0502525316942,5.79843016859412,8.43709945169241));
#17195=CARTESIAN_POINT('Ctrl Pts',(10.0502525316942,5.78835717995633,8.37520120352267));
#17196=CARTESIAN_POINT('Ctrl Pts',(10.0502525316942,5.78034060190006,8.31255178250645));
#17197=CARTESIAN_POINT('Ctrl Pts',(10.0502525316942,5.77394633717213,8.24933415385039));
#17198=CARTESIAN_POINT('Ctrl Pts',(10.0502525316942,5.76796747841793,8.18604879427487));
#17199=CARTESIAN_POINT('Ctrl Pts',(10.0502525316942,5.76091367696946,8.12332066784839));
#17200=CARTESIAN_POINT('Ctrl Pts',(10.0502525316942,5.75154264947446,8.06168961610356));
#17201=CARTESIAN_POINT('Ctrl Pts',(10.0502525316942,5.73934420595248,8.00141929583747));
#17202=CARTESIAN_POINT('Ctrl Pts',(10.0502525316942,5.72431483522833,7.94258074919088));
#17203=CARTESIAN_POINT('Ctrl Pts',(10.0502525316942,5.7067581439046,7.88512587067823));
#17204=CARTESIAN_POINT('Ctrl Pts',(10.0502525316942,5.68709020402104,7.82895914189736));
#17205=CARTESIAN_POINT('Ctrl Pts',(10.0502525316942,5.66561822174726,7.77401905533046));
#17206=CARTESIAN_POINT('Ctrl Pts',(10.0502525316942,5.64241804293469,7.72032292706671));
#17207=CARTESIAN_POINT('Ctrl Pts',(10.0502525316942,5.61742944592276,7.6679311867486));
#17208=CARTESIAN_POINT('Ctrl Pts',(10.0502525316942,5.59050809253397,7.61692741952956));
#17209=CARTESIAN_POINT('Ctrl Pts',(10.0502525316942,5.56148971316608,7.56739405041849));
#17210=CARTESIAN_POINT('Ctrl Pts',(10.0502525316942,5.53026090613148,7.51938467268366));
#17211=CARTESIAN_POINT('Ctrl Pts',(10.0502525316942,5.4967684895078,7.47292244003411));
#17212=CARTESIAN_POINT('Ctrl Pts',(10.0502525316942,5.46814894648693,7.43699488267859));
#17213=CARTESIAN_POINT('Ctrl Pts',(10.0502525316942,5.44565864507534,7.41074614986957));
#17214=CARTESIAN_POINT('Ctrl Pts',(10.0502525316942,5.43021006317766,7.39355619607562));
#17215=CARTESIAN_POINT('Ctrl Pts',(10.0502525316942,5.42237201204004,7.38503851882133));
#17216=CARTESIAN_POINT('',(10.0502525316942,6.33125817110613,6.62239247796685));
#17217=CARTESIAN_POINT('Origin',(10.0502525316942,0.,0.));
#17218=CARTESIAN_POINT('',(10.0502525316942,7.92891439885425,7.2752703501265));
#17219=CARTESIAN_POINT('Ctrl Pts',(10.0502525316942,6.33125817110613,6.62239247796685));
#17220=CARTESIAN_POINT('Ctrl Pts',(10.0502525316942,6.33803255463449,6.63100021625014));
#17221=CARTESIAN_POINT('Ctrl Pts',(10.0502525316942,6.35173489391119,6.64806877891362));
#17222=CARTESIAN_POINT('Ctrl Pts',(10.0502525316942,6.37274911883029,6.67323088220656));
#17223=CARTESIAN_POINT('Ctrl Pts',(10.0502525316942,6.40169119143333,6.70589726716278));
#17224=CARTESIAN_POINT('Ctrl Pts',(10.0502525316942,6.43941941070578,6.74524402479143));
#17225=CARTESIAN_POINT('Ctrl Pts',(10.0502525316942,6.47871780200897,6.7830773250095));
#17226=CARTESIAN_POINT('Ctrl Pts',(10.0502525316942,6.51961240030403,6.81935524839631));
#17227=CARTESIAN_POINT('Ctrl Pts',(10.0502525316942,6.56213509649465,6.85401859544624));
#17228=CARTESIAN_POINT('Ctrl Pts',(10.0502525316942,6.60632140469038,6.88699086799345));
#17229=CARTESIAN_POINT('Ctrl Pts',(10.0502525316942,6.65219708634863,6.91819814506577));
#17230=CARTESIAN_POINT('Ctrl Pts',(10.0502525316942,6.69976489037577,6.9475881722867));
#17231=CARTESIAN_POINT('Ctrl Pts',(10.0502525316942,6.74899181640015,6.97514889902642));
#17232=CARTESIAN_POINT('Ctrl Pts',(10.0502525316942,6.79979302943897,7.00093106972056));
#17233=CARTESIAN_POINT('Ctrl Pts',(10.0502525316942,6.85202406661451,7.02506036068034));
#17234=CARTESIAN_POINT('Ctrl Pts',(10.0502525316942,6.90550961656264,7.04770332746178));
#17235=CARTESIAN_POINT('Ctrl Pts',(10.0502525316942,6.96006716732954,7.06903990194018));
#17236=CARTESIAN_POINT('Ctrl Pts',(10.0502525316942,7.01553102941681,7.08923522069654));
#17237=CARTESIAN_POINT('Ctrl Pts',(10.0502525316942,7.07177895456438,7.10840869098247));
#17238=CARTESIAN_POINT('Ctrl Pts',(10.0502525316942,7.12874865657033,7.12661440941494));
#17239=CARTESIAN_POINT('Ctrl Pts',(10.0502525316942,7.18641725377035,7.14386341521534));
#17240=CARTESIAN_POINT('Ctrl Pts',(10.0502525316942,7.24478653536347,7.16013937508649));
#17241=CARTESIAN_POINT('Ctrl Pts',(10.0502525316942,7.30386662226907,7.17541617812316));
#17242=CARTESIAN_POINT('Ctrl Pts',(10.0502525316942,7.36365880682929,7.18967631564937));
#17243=CARTESIAN_POINT('Ctrl Pts',(10.0502525316942,7.42414298774012,7.2029245901952));
#17244=CARTESIAN_POINT('Ctrl Pts',(10.0502525316942,7.48528632500984,7.21517989232968));
#17245=CARTESIAN_POINT('Ctrl Pts',(10.0502525316942,7.54704857406782,7.22647049097858));
#17246=CARTESIAN_POINT('Ctrl Pts',(10.0502525316942,7.60938839179095,7.23682832548438));
#17247=CARTESIAN_POINT('Ctrl Pts',(10.0502525316942,7.67226934177745,7.24628378544296));
#17248=CARTESIAN_POINT('Ctrl Pts',(10.0502525316942,7.73566511738401,7.254861054624));
#17249=CARTESIAN_POINT('Ctrl Pts',(10.0502525316942,7.79955765803962,7.26257856558425));
#17250=CARTESIAN_POINT('Ctrl Pts',(10.0502525316942,7.85106030720964,7.26807493359233));
#17251=CARTESIAN_POINT('Ctrl Pts',(10.0502525316942,7.88990344551799,7.27181932978281));
#17252=CARTESIAN_POINT('Ctrl Pts',(10.0502525316942,7.91589476537953,7.27414795055897));
#17253=CARTESIAN_POINT('Ctrl Pts',(10.0502525316942,7.92891439885425,7.2752703501265));
#17254=CARTESIAN_POINT('',(10.0502525316942,7.43908464225652,5.34798390487229));
#17255=CARTESIAN_POINT('Ctrl Pts',(10.0502525316942,7.92891439885425,7.2752703501265));
#17256=CARTESIAN_POINT('Ctrl Pts',(10.0502525316942,7.94891084739874,7.24246834654844));
#17257=CARTESIAN_POINT('Ctrl Pts',(10.0502525316942,7.98717978950973,7.17831007049656));
#17258=CARTESIAN_POINT('Ctrl Pts',(10.0502525316942,8.03941132011983,7.08640986444703));
#17259=CARTESIAN_POINT('Ctrl Pts',(10.0502525316942,8.09869101763159,6.97256625288353));
#17260=CARTESIAN_POINT('Ctrl Pts',(10.0502525316942,8.15552703155277,6.84473975688512));
#17261=CARTESIAN_POINT('Ctrl Pts',(10.0502525316942,8.19531386354866,6.73121306554078));
#17262=CARTESIAN_POINT('Ctrl Pts',(10.0502525316942,8.21862212728407,6.63151085898163));
#17263=CARTESIAN_POINT('Ctrl Pts',(10.0502525316942,8.22655212821854,6.54471580350543));
#17264=CARTESIAN_POINT('Ctrl Pts',(10.0502525316942,8.22086585997457,6.46935831372324));
#17265=CARTESIAN_POINT('Ctrl Pts',(10.0502525316942,8.20424193086582,6.40320361025513));
#17266=CARTESIAN_POINT('Ctrl Pts',(10.0502525316942,8.17999182956336,6.34348879371404));
#17267=CARTESIAN_POINT('Ctrl Pts',(10.0502525316942,8.15151829405778,6.2873754147921));
#17268=CARTESIAN_POINT('Ctrl Pts',(10.0502525316942,8.12184190992835,6.23234494937036));
#17269=CARTESIAN_POINT('Ctrl Pts',(10.0502525316942,8.09313431783932,6.1765889417745));
#17270=CARTESIAN_POINT('Ctrl Pts',(10.0502525316942,8.06615036325875,6.11948306053102));
#17271=CARTESIAN_POINT('Ctrl Pts',(10.0502525316942,8.04053373452353,6.06133545932041));
#17272=CARTESIAN_POINT('Ctrl Pts',(10.0502525316942,8.01529125034138,6.00299507467205));
#17273=CARTESIAN_POINT('Ctrl Pts',(10.0502525316942,7.98919862941808,5.94551682580168));
#17274=CARTESIAN_POINT('Ctrl Pts',(10.0502525316942,7.96124121028423,5.88979801918435));
#17275=CARTESIAN_POINT('Ctrl Pts',(10.0502525316942,7.93101524786534,5.83624706470931));
#17276=CARTESIAN_POINT('Ctrl Pts',(10.0502525316942,7.89853935606421,5.78493261248025));
#17277=CARTESIAN_POINT('Ctrl Pts',(10.0502525316942,7.86408741650604,5.73571509186187));
#17278=CARTESIAN_POINT('Ctrl Pts',(10.0502525316942,7.82802562040593,5.68837508612421));
#17279=CARTESIAN_POINT('Ctrl Pts',(10.0502525316942,7.79062713132508,5.64275916621446));
#17280=CARTESIAN_POINT('Ctrl Pts',(10.0502525316942,7.75196943392054,5.59886036305501));
#17281=CARTESIAN_POINT('Ctrl Pts',(10.0502525316942,7.71201392777609,5.55675475816771));
#17282=CARTESIAN_POINT('Ctrl Pts',(10.0502525316942,7.67064916836037,5.51656644870715));
#17283=CARTESIAN_POINT('Ctrl Pts',(10.0502525316942,7.62774439672625,5.47842458761391));
#17284=CARTESIAN_POINT('Ctrl Pts',(10.0502525316942,7.58320832269043,5.44241518816367));
#17285=CARTESIAN_POINT('Ctrl Pts',(10.0502525316942,7.5369975221287,5.4085767049601));
#17286=CARTESIAN_POINT('Ctrl Pts',(10.0502525316942,7.49867649345608,5.38325149258725));
#17287=CARTESIAN_POINT('Ctrl Pts',(10.0502525316942,7.46917564122634,5.36523734954955));
#17288=CARTESIAN_POINT('Ctrl Pts',(10.0502525316942,7.44917117889019,5.35366260632437));
#17289=CARTESIAN_POINT('Ctrl Pts',(10.0502525316942,7.43908464225652,5.34798390487229));
#17290=CARTESIAN_POINT('',(10.0502525316942,8.06781615908999,4.34180314898733));
#17291=CARTESIAN_POINT('Origin',(10.0502525316942,0.,0.));
#17292=CARTESIAN_POINT('',(10.0502525316942,9.78902788303806,4.46902397810655));
#17293=CARTESIAN_POINT('Ctrl Pts',(10.0502525316942,8.06781615908999,4.34180314898733));
#17294=CARTESIAN_POINT('Ctrl Pts',(10.0502525316942,8.07691891810119,4.34789619493555));
#17295=CARTESIAN_POINT('Ctrl Pts',(10.0502525316942,8.09522509309135,4.35989510698125));
#17296=CARTESIAN_POINT('Ctrl Pts',(10.0502525316942,8.1229863261673,4.37733193665808));
#17297=CARTESIAN_POINT('Ctrl Pts',(10.0502525316942,8.16060634100777,4.39945592264773));
#17298=CARTESIAN_POINT('Ctrl Pts',(10.0502525316942,8.20864682657585,4.42521825196285));
#17299=CARTESIAN_POINT('Ctrl Pts',(10.0502525316942,8.25771295042534,4.44905598790391));
#17300=CARTESIAN_POINT('Ctrl Pts',(10.0502525316942,8.30781651946229,4.47092121748728));
#17301=CARTESIAN_POINT('Ctrl Pts',(10.0502525316942,8.35896957008516,4.49074778380617));
#17302=CARTESIAN_POINT('Ctrl Pts',(10.0502525316942,8.41118223898599,4.50845195831808));
#17303=CARTESIAN_POINT('Ctrl Pts',(10.0502525316942,8.46445618393006,4.52395547727261));
#17304=CARTESIAN_POINT('Ctrl Pts',(10.0502525316942,8.51877787179233,4.53720779434568));
#17305=CARTESIAN_POINT('Ctrl Pts',(10.0502525316942,8.5741121935049,4.54820764638295));
#17306=CARTESIAN_POINT('Ctrl Pts',(10.0502525316942,8.63039414709753,4.557029509662));
#17307=CARTESIAN_POINT('Ctrl Pts',(10.0502525316942,8.68752517632497,4.5638375509418));
#17308=CARTESIAN_POINT('Ctrl Pts',(10.0502525316942,8.7453900186693,4.56884434816008));
#17309=CARTESIAN_POINT('Ctrl Pts',(10.0502525316942,8.80387069695484,4.57227742599473));
#17310=CARTESIAN_POINT('Ctrl Pts',(10.0502525316942,8.86286066111437,4.57434503953799));
#17311=CARTESIAN_POINT('Ctrl Pts',(10.0502525316942,8.92228054501355,4.57519852862449));
#17312=CARTESIAN_POINT('Ctrl Pts',(10.0502525316942,8.98208782772813,4.57490858968921));
#17313=CARTESIAN_POINT('Ctrl Pts',(10.0502525316942,9.0422641588092,4.57349279247872));
#17314=CARTESIAN_POINT('Ctrl Pts',(10.0502525316942,9.10280619261976,4.57093505021141));
#17315=CARTESIAN_POINT('Ctrl Pts',(10.0502525316942,9.16371548601266,4.56720740240461));
#17316=CARTESIAN_POINT('Ctrl Pts',(10.0502525316942,9.22498785759991,4.56229279796226));
#17317=CARTESIAN_POINT('Ctrl Pts',(10.0502525316942,9.28660567396873,4.55620201600645));
#17318=CARTESIAN_POINT('Ctrl Pts',(10.0502525316942,9.34854353993788,4.54896317065147));
#17319=CARTESIAN_POINT('Ctrl Pts',(10.0502525316942,9.4107719162247,4.54061558349964));
#17320=CARTESIAN_POINT('Ctrl Pts',(10.0502525316942,9.47326135298215,4.53120240639841));
#17321=CARTESIAN_POINT('Ctrl Pts',(10.0502525316942,9.53598658803447,4.52076380103831));
#17322=CARTESIAN_POINT('Ctrl Pts',(10.0502525316942,9.59893007547295,4.50933089675096));
#17323=CARTESIAN_POINT('Ctrl Pts',(10.0502525316942,9.6620803346471,4.49692680496291));
#17324=CARTESIAN_POINT('Ctrl Pts',(10.0502525316942,9.71276073586856,4.48623896772408));
#17325=CARTESIAN_POINT('Ctrl Pts',(10.0502525316942,9.7508598377266,4.47779691026849));
#17326=CARTESIAN_POINT('Ctrl Pts',(10.0502525316942,9.77629863524131,4.47197980068818));
#17327=CARTESIAN_POINT('Ctrl Pts',(10.0502525316942,9.78902788303806,4.46902397810655));
#17328=CARTESIAN_POINT('',(10.0502525316942,8.7276078365385,2.78743136471945));
#17329=CARTESIAN_POINT('Ctrl Pts',(10.0502525316942,9.78902788303806,4.46902397810655));
#17330=CARTESIAN_POINT('Ctrl Pts',(10.0502525316942,9.7979092591739,4.43164817642871));
#17331=CARTESIAN_POINT('Ctrl Pts',(10.0502525316942,9.81447918831044,4.35880427644625));
#17332=CARTESIAN_POINT('Ctrl Pts',(10.0502525316942,9.83575560039739,4.25526155603325));
#17333=CARTESIAN_POINT('Ctrl Pts',(10.0502525316942,9.85695433232581,4.12867141346467));
#17334=CARTESIAN_POINT('Ctrl Pts',(10.0502525316942,9.87150803413088,3.98953789729602));
#17335=CARTESIAN_POINT('Ctrl Pts',(10.0502525316942,9.87426588302275,3.86927279048049));
#17336=CARTESIAN_POINT('Ctrl Pts',(10.0502525316942,9.86562368292838,3.76724770763979));
#17337=CARTESIAN_POINT('Ctrl Pts',(10.0502525316942,9.84634441482148,3.68225019949279));
#17338=CARTESIAN_POINT('Ctrl Pts',(10.0502525316942,9.81764970735851,3.61233812130575));
#17339=CARTESIAN_POINT('Ctrl Pts',(10.0502525316942,9.78139648362373,3.55455833609672));
#17340=CARTESIAN_POINT('Ctrl Pts',(10.0502525316942,9.73988037363202,3.50525986412372));
#17341=CARTESIAN_POINT('Ctrl Pts',(10.0502525316942,9.6954604444488,3.46069167580983));
#17342=CARTESIAN_POINT('Ctrl Pts',(10.0502525316942,9.65023117691875,3.41752510010333));
#17343=CARTESIAN_POINT('Ctrl Pts',(10.0502525316942,9.60569908050971,3.37336911957978));
#17344=CARTESIAN_POINT('Ctrl Pts',(10.0502525316942,9.56238912688746,3.32739669964523));
#17345=CARTESIAN_POINT('Ctrl Pts',(10.0502525316942,9.5200576682471,3.28001101822472));
#17346=CARTESIAN_POINT('Ctrl Pts',(10.0502525316942,9.47802246886347,3.23232637183425));
#17347=CARTESIAN_POINT('Ctrl Pts',(10.0502525316942,9.43544515599928,3.18572437199394));
#17348=CARTESIAN_POINT('Ctrl Pts',(10.0502525316942,9.3916380122022,3.14137195551156));
#17349=CARTESIAN_POINT('Ctrl Pts',(10.0502525316942,9.34634325868463,3.09978230736302));
#17350=CARTESIAN_POINT('Ctrl Pts',(10.0502525316942,9.29959981236885,3.0610149656645));
#17351=CARTESIAN_POINT('Ctrl Pts',(10.0502525316942,9.25162502046097,3.02485255677715));
#17352=CARTESIAN_POINT('Ctrl Pts',(10.0502525316942,9.20269934800391,2.99097324368152));
#17353=CARTESIAN_POINT('Ctrl Pts',(10.0502525316942,9.15303517679781,2.95914669449447));
#17354=CARTESIAN_POINT('Ctrl Pts',(10.0502525316942,9.10270404556727,2.92934233715353));
#17355=CARTESIAN_POINT('Ctrl Pts',(10.0502525316942,9.05169275361811,2.9016444576704));
#17356=CARTESIAN_POINT('Ctrl Pts',(10.0502525316942,8.99993365903229,2.87620551770673));
#17357=CARTESIAN_POINT('Ctrl Pts',(10.0502525316942,8.94734231311461,2.85318875574511));
#17358=CARTESIAN_POINT('Ctrl Pts',(10.0502525316942,8.89385847330528,2.83270418548989));
#17359=CARTESIAN_POINT('Ctrl Pts',(10.0502525316942,8.83945272393405,2.81480179823484));
#17360=CARTESIAN_POINT('Ctrl Pts',(10.0502525316942,8.79518133889446,2.80255793908285));
#17361=CARTESIAN_POINT('Ctrl Pts',(10.0502525316942,8.76155768480736,2.7945417356489));
#17362=CARTESIAN_POINT('Ctrl Pts',(10.0502525316942,8.73895551818547,2.78971521950536));
#17363=CARTESIAN_POINT('Ctrl Pts',(10.0502525316942,8.7276078365385,2.78743136471945));
#17364=CARTESIAN_POINT('',(10.0502525316942,9.01464008964162,1.6362078766636));
#17365=CARTESIAN_POINT('Origin',(10.0502525316942,0.,0.));
#17366=CARTESIAN_POINT('',(10.0502525316942,10.6909231138624,1.22531840158854));
#17367=CARTESIAN_POINT('Ctrl Pts',(10.0502525316942,9.01464008964162,1.6362078766636));
#17368=CARTESIAN_POINT('Ctrl Pts',(10.0502525316942,9.02518018266099,1.63918980048658));
#17369=CARTESIAN_POINT('Ctrl Pts',(10.0502525316942,9.04629825740996,1.64494452480213));
#17370=CARTESIAN_POINT('Ctrl Pts',(10.0502525316942,9.07808903572539,1.65294924248453));
#17371=CARTESIAN_POINT('Ctrl Pts',(10.0502525316942,9.12070448363665,1.66236517961207));
#17372=CARTESIAN_POINT('Ctrl Pts',(10.0502525316942,9.17435469805521,1.67202128432359));
#17373=CARTESIAN_POINT('Ctrl Pts',(10.0502525316942,9.22838562038483,1.67953005230647));
#17374=CARTESIAN_POINT('Ctrl Pts',(10.0502525316942,9.28279367373423,1.68484226707077));
#17375=CARTESIAN_POINT('Ctrl Pts',(10.0502525316942,9.33756986179013,1.68789129020751));
#17376=CARTESIAN_POINT('Ctrl Pts',(10.0502525316942,9.39269795157698,1.68859435873067));
#17377=CARTESIAN_POINT('Ctrl Pts',(10.0502525316942,9.44815533489435,1.68687652711276));
#17378=CARTESIAN_POINT('Ctrl Pts',(10.0502525316942,9.50391352130234,1.68269390490855));
#17379=CARTESIAN_POINT('Ctrl Pts',(10.0502525316942,9.55993872975698,1.67605614008548));
#17380=CARTESIAN_POINT('Ctrl Pts',(10.0502525316942,9.61619215414635,1.66705415050613));
#17381=CARTESIAN_POINT('Ctrl Pts',(10.0502525316942,9.67263079222962,1.65587452359108));
#17382=CARTESIAN_POINT('Ctrl Pts',(10.0502525316942,9.72921071303343,1.64275505105007));
#17383=CARTESIAN_POINT('Ctrl Pts',(10.0502525316942,9.78589002258816,1.62794857866286));
#17384=CARTESIAN_POINT('Ctrl Pts',(10.0502525316942,9.84263174012077,1.6116860945735));
#17385=CARTESIAN_POINT('Ctrl Pts',(10.0502525316942,9.89940715053283,1.59413605700217));
#17386=CARTESIAN_POINT('Ctrl Pts',(10.0502525316942,9.9561976604221,1.57537884194225));
#17387=CARTESIAN_POINT('Ctrl Pts',(10.0502525316942,10.0129912468249,1.55543682981628));
#17388=CARTESIAN_POINT('Ctrl Pts',(10.0502525316942,10.0697797567623,1.53429575504446));
#17389=CARTESIAN_POINT('Ctrl Pts',(10.0502525316942,10.1265560306252,1.51192854453357));
#17390=CARTESIAN_POINT('Ctrl Pts',(10.0502525316942,10.1833108225988,1.48832027384755));
#17391=CARTESIAN_POINT('Ctrl Pts',(10.0502525316942,10.2400306932429,1.4634866435649));
#17392=CARTESIAN_POINT('Ctrl Pts',(10.0502525316942,10.2967001780439,1.43746223933981));
#17393=CARTESIAN_POINT('Ctrl Pts',(10.0502525316942,10.353303334518,1.41029358637874));
#17394=CARTESIAN_POINT('Ctrl Pts',(10.0502525316942,10.4098254888505,1.38203082503059));
#17395=CARTESIAN_POINT('Ctrl Pts',(10.0502525316942,10.4662550259293,1.35271995777451));
#17396=CARTESIAN_POINT('Ctrl Pts',(10.0502525316942,10.5225848780961,1.32239601234813));
#17397=CARTESIAN_POINT('Ctrl Pts',(10.0502525316942,10.5788112684272,1.29108451674038));
#17398=CARTESIAN_POINT('Ctrl Pts',(10.0502525316942,10.6237084709174,1.26525867423012));
#17399=CARTESIAN_POINT('Ctrl Pts',(10.0502525316942,10.6573341307832,1.24545653053149));
#17400=CARTESIAN_POINT('Ctrl Pts',(10.0502525316942,10.6797302792078,1.23206310981063));
#17401=CARTESIAN_POINT('Ctrl Pts',(10.0502525316942,10.6909231138624,1.22531840158854));
#17402=CARTESIAN_POINT('',(10.0502525316942,9.16181196696065,-0.0459743785884358));
#17403=CARTESIAN_POINT('Ctrl Pts',(10.0502525316942,10.6909231138624,1.22531840158854));
#17404=CARTESIAN_POINT('Ctrl Pts',(10.0502525316942,10.6878200466132,1.18702740569167));
#17405=CARTESIAN_POINT('Ctrl Pts',(10.0502525316942,10.6810689826619,1.11262835024222));
#17406=CARTESIAN_POINT('Ctrl Pts',(10.0502525316942,10.6693075927691,1.00757859836431));
#17407=CARTESIAN_POINT('Ctrl Pts',(10.0502525316942,10.6503502795328,0.880633449950656));
#17408=CARTESIAN_POINT('Ctrl Pts',(10.0502525316942,10.6211970514875,0.743812271574576));
#17409=CARTESIAN_POINT('Ctrl Pts',(10.0502525316942,10.5866559598108,0.628581135879225));
#17410=CARTESIAN_POINT('Ctrl Pts',(10.0502525316942,10.5469092546456,0.534220102715978));
#17411=CARTESIAN_POINT('Ctrl Pts',(10.0502525316942,10.5023079065862,0.459340290208067));
#17412=CARTESIAN_POINT('Ctrl Pts',(10.0502525316942,10.4534135977985,0.40171710493522));
#17413=CARTESIAN_POINT('Ctrl Pts',(10.0502525316942,10.4010797975679,0.357968125936964));
#17414=CARTESIAN_POINT('Ctrl Pts',(10.0502525316942,10.3463615649927,0.323911676451426));
#17415=CARTESIAN_POINT('Ctrl Pts',(10.0502525316942,10.2903433742921,0.295251323542576));
#17416=CARTESIAN_POINT('Ctrl Pts',(10.0502525316942,10.2339885791981,0.268174082740676));
#17417=CARTESIAN_POINT('Ctrl Pts',(10.0502525316942,10.1779910903389,0.239940424315885));
#17418=CARTESIAN_POINT('Ctrl Pts',(10.0502525316942,10.1225946176937,0.209601566462141));
#17419=CARTESIAN_POINT('Ctrl Pts',(10.0502525316942,10.0676920272606,0.177616245484636));
#17420=CARTESIAN_POINT('Ctrl Pts',(10.0502525316942,10.0129788108676,0.145255042779231));
#17421=CARTESIAN_POINT('Ctrl Pts',(10.0502525316942,9.95808457009925,0.11409102040857));
#17422=CARTESIAN_POINT('Ctrl Pts',(10.0502525316942,9.90271585009609,0.0854465176078907));
#17423=CARTESIAN_POINT('Ctrl Pts',(10.0502525316942,9.84678607154126,0.0598892603187502));
#17424=CARTESIAN_POINT('Ctrl Pts',(10.0502525316942,9.79035064491696,0.0374638466641572));
#17425=CARTESIAN_POINT('Ctrl Pts',(10.0502525316942,9.73354910755133,0.017896378048051));
#17426=CARTESIAN_POINT('Ctrl Pts',(10.0502525316942,9.67654874444263,0.000794100811299831));
#17427=CARTESIAN_POINT('Ctrl Pts',(10.0502525316942,9.61948036621956,-0.0141276732699903));
#17428=CARTESIAN_POINT('Ctrl Pts',(10.0502525316942,9.56240256296547,-0.0269201266367288));
#17429=CARTESIAN_POINT('Ctrl Pts',(10.0502525316942,9.50532882588415,-0.0374990192894116));
#17430=CARTESIAN_POINT('Ctrl Pts',(10.0502525316942,9.44824193693312,-0.0456984490690175));
#17431=CARTESIAN_POINT('Ctrl Pts',(10.0502525316942,9.39111202409575,-0.0513370708710177));
#17432=CARTESIAN_POINT('Ctrl Pts',(10.0502525316942,9.33391578939727,-0.0542916394702416));
#17433=CARTESIAN_POINT('Ctrl Pts',(10.0502525316942,9.27664070503215,-0.0545055203789815));
#17434=CARTESIAN_POINT('Ctrl Pts',(10.0502525316942,9.23075255525014,-0.0524695120683285));
#17435=CARTESIAN_POINT('Ctrl Pts',(10.0502525316942,9.19629741683749,-0.0497030940542379));
#17436=CARTESIAN_POINT('Ctrl Pts',(10.0502525316942,9.17331000347738,-0.0473089300876987));
#17437=CARTESIAN_POINT('Ctrl Pts',(10.0502525316942,9.16181196696065,-0.0459743785884358));
#17438=CARTESIAN_POINT('',(10.0502525316942,9.07904823952839,-1.22955082275859));
#17439=CARTESIAN_POINT('Origin',(10.0502525316942,0.,0.));
#17440=CARTESIAN_POINT('',(10.0502525316942,10.5463163022605,-2.13832987737225));
#17441=CARTESIAN_POINT('Ctrl Pts',(10.0502525316942,9.07904823952839,-1.22955082275859));
#17442=CARTESIAN_POINT('Ctrl Pts',(10.0502525316942,9.08999392881405,-1.22997191254093));
#17443=CARTESIAN_POINT('Ctrl Pts',(10.0502525316942,9.11185671902711,-1.23102468846705));
#17444=CARTESIAN_POINT('Ctrl Pts',(10.0502525316942,9.14456513970113,-1.23323564031797));
#17445=CARTESIAN_POINT('Ctrl Pts',(10.0502525316942,9.18800452372235,-1.23744944958329));
#17446=CARTESIAN_POINT('Ctrl Pts',(10.0502525316942,9.24201281020108,-1.24484477628256));
#17447=CARTESIAN_POINT('Ctrl Pts',(10.0502525316942,9.29571960787763,-1.2543999867847));
#17448=CARTESIAN_POINT('Ctrl Pts',(10.0502525316942,9.34910630619445,-1.26616078343298));
#17449=CARTESIAN_POINT('Ctrl Pts',(10.0502525316942,9.40214375674832,-1.28018776310679));
#17450=CARTESIAN_POINT('Ctrl Pts',(10.0502525316942,9.45479094589287,-1.29655462181801));
#17451=CARTESIAN_POINT('Ctrl Pts',(10.0502525316942,9.50700321251013,-1.31532565068075));
#17452=CARTESIAN_POINT('Ctrl Pts',(10.0502525316942,9.55873989768809,-1.33653378795886));
#17453=CARTESIAN_POINT('Ctrl Pts',(10.0502525316942,9.60997185513068,-1.36015941897336));
#17454=CARTESIAN_POINT('Ctrl Pts',(10.0502525316942,9.6606902731969,-1.38610408395052));
#17455=CARTESIAN_POINT('Ctrl Pts',(10.0502525316942,9.7109119130093,-1.41417703928493));
#17456=CARTESIAN_POINT('Ctrl Pts',(10.0502525316942,9.76066847540881,-1.44413855620418));
#17457=CARTESIAN_POINT('Ctrl Pts',(10.0502525316942,9.80999825050556,-1.47573521813323));
#17458=CARTESIAN_POINT('Ctrl Pts',(10.0502525316942,9.85893744675637,-1.50873591460517));
#17459=CARTESIAN_POINT('Ctrl Pts',(10.0502525316942,9.90751081093262,-1.54297155887855));
#17460=CARTESIAN_POINT('Ctrl Pts',(10.0502525316942,9.95572549720588,-1.57835996316384));
#17461=CARTESIAN_POINT('Ctrl Pts',(10.0502525316942,10.003576986989,-1.61487612711423));
#17462=CARTESIAN_POINT('Ctrl Pts',(10.0502525316942,10.0510531180319,-1.65253109869336));
#17463=CARTESIAN_POINT('Ctrl Pts',(10.0502525316942,10.0981387150956,-1.69134841350201));
#17464=CARTESIAN_POINT('Ctrl Pts',(10.0502525316942,10.1448203729832,-1.73133940840847));
#17465=CARTESIAN_POINT('Ctrl Pts',(10.0502525316942,10.1910901617733,-1.77248499825981));
#17466=CARTESIAN_POINT('Ctrl Pts',(10.0502525316942,10.2369440613944,-1.81474751134677));
#17467=CARTESIAN_POINT('Ctrl Pts',(10.0502525316942,10.2823812867227,-1.85807777307013));
#17468=CARTESIAN_POINT('Ctrl Pts',(10.0502525316942,10.3274033763511,-1.90242356266618));
#17469=CARTESIAN_POINT('Ctrl Pts',(10.0502525316942,10.3720134991994,-1.94773753991041));
#17470=CARTESIAN_POINT('Ctrl Pts',(10.0502525316942,10.4162157576914,-1.99398420741813));
#17471=CARTESIAN_POINT('Ctrl Pts',(10.0502525316942,10.4600144483414,-2.04113811949547));
#17472=CARTESIAN_POINT('Ctrl Pts',(10.0502525316942,10.4947336011034,-2.07957395387303));
#17473=CARTESIAN_POINT('Ctrl Pts',(10.0502525316942,10.5205943051056,-2.10879781201984));
#17474=CARTESIAN_POINT('Ctrl Pts',(10.0502525316942,10.5377555133892,-2.12845650254365));
#17475=CARTESIAN_POINT('Ctrl Pts',(10.0502525316942,10.5463163022605,-2.13832987737225));
#17476=CARTESIAN_POINT('Ctrl Pts',(10.0502525316942,10.5463163022605,-2.13832987737225));
#17477=CARTESIAN_POINT('Ctrl Pts',(10.0502525316942,10.531532541469,-2.17378787802072));
#17478=CARTESIAN_POINT('Ctrl Pts',(10.0502525316942,10.5021213256069,-2.24245939102107));
#17479=CARTESIAN_POINT('Ctrl Pts',(10.0502525316942,10.4584734205235,-2.33873317272541));
#17480=CARTESIAN_POINT('Ctrl Pts',(10.0502525316942,10.4012157360254,-2.45360705137856));
#17481=CARTESIAN_POINT('Ctrl Pts',(10.0502525316942,10.3312092992132,-2.57472288173342));
#17482=CARTESIAN_POINT('Ctrl Pts',(10.0502525316942,10.2627503896831,-2.6736404198842));
#17483=CARTESIAN_POINT('Ctrl Pts',(10.0502525316942,10.1957898638803,-2.751100687992));
#17484=CARTESIAN_POINT('Ctrl Pts',(10.0502525316942,10.1302323265723,-2.80853304709422));
#17485=CARTESIAN_POINT('Ctrl Pts',(10.0502525316942,10.0659245320707,-2.84822678059402));
#17486=CARTESIAN_POINT('Ctrl Pts',(10.0502525316942,10.0026329523419,-2.8736624985001));
#17487=CARTESIAN_POINT('Ctrl Pts',(10.0502525316942,9.94006879903196,-2.88914324293729));
#17488=CARTESIAN_POINT('Ctrl Pts',(10.0502525316942,9.8779357976215,-2.89909028540996));
#17489=CARTESIAN_POINT('Ctrl Pts',(10.0502525316942,9.81597187495431,-2.90742768231934));
#17490=CARTESIAN_POINT('Ctrl Pts',(10.0502525316942,9.753990418012,-2.91697531144329));
#17491=CARTESIAN_POINT('Ctrl Pts',(10.0502525316942,9.69193001905628,-2.92871082842625));
#17492=CARTESIAN_POINT('Ctrl Pts',(10.0502525316942,9.62983054491074,-2.94216484288864));
#17493=CARTESIAN_POINT('Ctrl Pts',(10.0502525316942,9.56779502233835,-2.95603486191442));
#17494=CARTESIAN_POINT('Ctrl Pts',(10.0502525316942,9.50595728442294,-2.96871035517328));
#17495=CARTESIAN_POINT('Ctrl Pts',(10.0502525316942,9.44444686430419,-2.97884302078014));
#17496=CARTESIAN_POINT('Ctrl Pts',(10.0502525316942,9.38335685712271,-2.98586616479853));
#17497=CARTESIAN_POINT('Ctrl Pts',(10.0502525316942,9.32275374295661,-2.98975449467364));
#17498=CARTESIAN_POINT('Ctrl Pts',(10.0502525316942,9.26268559037018,-2.99081162285579));
#17499=CARTESIAN_POINT('Ctrl Pts',(10.0502525316942,9.20319012929579,-2.98946277417915));
#17500=CARTESIAN_POINT('Ctrl Pts',(10.0502525316942,9.144303794535,-2.9860191259415));
#17501=CARTESIAN_POINT('Ctrl Pts',(10.0502525316942,9.08606649232432,-2.98054746086824));
#17502=CARTESIAN_POINT('Ctrl Pts',(10.0502525316942,9.02851708515246,-2.97297183097014));
#17503=CARTESIAN_POINT('Ctrl Pts',(10.0502525316942,8.97169046427448,-2.96312913325008));
#17504=CARTESIAN_POINT('Ctrl Pts',(10.0502525316942,8.91561425843345,-2.95083766730389));
#17505=CARTESIAN_POINT('Ctrl Pts',(10.0502525316942,8.86030439480771,-2.93597302048693));
#17506=CARTESIAN_POINT('Ctrl Pts',(10.0502525316942,8.80576645976534,-2.91847745889582));
#17507=CARTESIAN_POINT('Ctrl Pts',(10.0502525316942,8.76275339706311,-2.90236088180168));
#17508=CARTESIAN_POINT('Ctrl Pts',(10.0502525316942,8.7308394833358,-2.88908263860953));
#17509=CARTESIAN_POINT('Ctrl Pts',(10.0502525316942,8.70971699141988,-2.87970215198308));
#17510=CARTESIAN_POINT('Ctrl Pts',(10.0502525316942,8.69919410795919,-2.87487982939776));
#17511=CARTESIAN_POINT('Origin',(29.1,0.,0.));
#17512=CARTESIAN_POINT('',(29.35,6.525,7.99082036443648E-16));
#17513=CARTESIAN_POINT('',(29.1,6.275,-7.68465866464964E-16));
#17514=CARTESIAN_POINT('Origin',(29.35,0.,0.));
#17515=CARTESIAN_POINT('Origin',(29.35,6.025,0.));
#17516=CARTESIAN_POINT('',(29.35,9.5,-1.16341445918999E-15));
#17517=CARTESIAN_POINT('Origin',(29.35,0.,0.));
#17518=CARTESIAN_POINT('Origin',(29.1,0.,0.));
#17519=CARTESIAN_POINT('',(28.85,10.,1.22464679914735E-15));
#17520=CARTESIAN_POINT('',(29.1,9.75,1.19403062916867E-15));
#17521=CARTESIAN_POINT('',(28.85,-10.,-1.22464679914735E-15));
#17522=CARTESIAN_POINT('Origin',(28.85,0.,0.));
#17523=CARTESIAN_POINT('Origin',(28.85,0.,0.));
#17524=CARTESIAN_POINT('Origin',(25.175,0.,0.));
#17525=CARTESIAN_POINT('',(25.175,-10.,-1.22464679914735E-15));
#17526=CARTESIAN_POINT('',(21.,-10.,-1.22464679914735E-15));
#17527=CARTESIAN_POINT('',(25.175,-10.,-1.22464679914735E-15));
#17528=CARTESIAN_POINT('Origin',(21.,0.,0.));
#17529=CARTESIAN_POINT('Origin',(15.75,0.,0.));
#17530=CARTESIAN_POINT('',(14.657256909085,15.6550387777217,-0.574937672128248));
#17531=CARTESIAN_POINT('',(15.8,14.2136654476498,-2.58416182157067));
#17532=CARTESIAN_POINT('Ctrl Pts',(14.657256909085,15.6550387777217,-0.574937672128247));
#17533=CARTESIAN_POINT('Ctrl Pts',(14.6763724381383,15.6262431452138,-0.80344402932419));
#17534=CARTESIAN_POINT('Ctrl Pts',(14.6998065311113,15.5861385521166,-1.05535166589827));
#17535=CARTESIAN_POINT('Ctrl Pts',(14.7651359522577,15.4797512169027,-1.49901297546982));
#17536=CARTESIAN_POINT('Ctrl Pts',(14.7991842945127,15.4284906283794,-1.63134031220526));
#17537=CARTESIAN_POINT('Ctrl Pts',(14.8880411294635,15.3057468955346,-1.8758277497676));
#17538=CARTESIAN_POINT('Ctrl Pts',(14.9527298447847,15.2276701479799,-1.94065298884131));
#17539=CARTESIAN_POINT('Ctrl Pts',(15.1817050684316,14.9444552503125,-2.21319070454604));
#17540=CARTESIAN_POINT('Ctrl Pts',(15.241493513239,14.8626126835113,-2.32251843283214));
#17541=CARTESIAN_POINT('Ctrl Pts',(15.4262634482943,14.6383589683629,-2.47073976049445));
#17542=CARTESIAN_POINT('Ctrl Pts',(15.4835457818315,14.5700757971062,-2.5074724098941));
#17543=CARTESIAN_POINT('Ctrl Pts',(15.6181084961337,14.4133333652787,-2.57062182851529));
#17544=CARTESIAN_POINT('Ctrl Pts',(15.7034661294672,14.3167713861451,-2.59269541157918));
#17545=CARTESIAN_POINT('Ctrl Pts',(15.8,14.2136654476498,-2.58416182157067));
#17546=CARTESIAN_POINT('',(15.8,14.4464654837189,0.0762417569101993));
#17547=CARTESIAN_POINT('Ctrl Pts',(15.8,14.4464654837189,0.0762417569101992));
#17548=CARTESIAN_POINT('Ctrl Pts',(15.7480221813552,14.5017894200628,0.0989497576662197));
#17549=CARTESIAN_POINT('Ctrl Pts',(15.6946673265391,14.55856814069,0.115136586527327));
#17550=CARTESIAN_POINT('Ctrl Pts',(15.5889287876155,14.6712292799262,0.130653500227229));
#17551=CARTESIAN_POINT('Ctrl Pts',(15.5369709165892,14.7266555496971,0.130547397724583));
#17552=CARTESIAN_POINT('Ctrl Pts',(15.4102920065978,14.8619679647836,0.108175767558855));
#17553=CARTESIAN_POINT('Ctrl Pts',(15.3183831004347,14.9605133746384,0.0733004344337784));
#17554=CARTESIAN_POINT('Ctrl Pts',(15.0640351589848,15.2315511945023,-0.110790343309231));
#17555=CARTESIAN_POINT('Ctrl Pts',(14.8841363199333,15.424113326113,-0.268817147256488));
#17556=CARTESIAN_POINT('Ctrl Pts',(14.657256909085,15.6550387777217,-0.574937672128247));
#17557=CARTESIAN_POINT('Origin',(15.8,0.,0.));
#17558=CARTESIAN_POINT('Origin',(15.75,0.,0.));
#17559=CARTESIAN_POINT('',(14.657256909085,15.0664921537995,4.29087481037367));
#17560=CARTESIAN_POINT('',(15.8,14.3165490635069,1.93458023611785));
#17561=CARTESIAN_POINT('Ctrl Pts',(14.657256909085,15.0664921537995,4.29087481037367));
#17562=CARTESIAN_POINT('Ctrl Pts',(14.6763724381383,15.1097182275582,4.06465401053977));
#17563=CARTESIAN_POINT('Ctrl Pts',(14.6998065311111,15.1494202336739,3.81268261045276));
#17564=CARTESIAN_POINT('Ctrl Pts',(14.7651359522566,15.1853387496715,3.35786013639478));
#17565=CARTESIAN_POINT('Ctrl Pts',(14.799184294511,15.1774784288,3.21616896751162));
#17566=CARTESIAN_POINT('Ctrl Pts',(14.8880411294635,15.136292974961,2.94571769745758));
#17567=CARTESIAN_POINT('Ctrl Pts',(14.9527298447853,15.0820696759655,2.85993818955593));
#17568=CARTESIAN_POINT('Ctrl Pts',(15.1817050684299,14.8969350877898,2.51322120266238));
#17569=CARTESIAN_POINT('Ctrl Pts',(15.2414935132389,14.8528823073187,2.38395361025704));
#17570=CARTESIAN_POINT('Ctrl Pts',(15.4262634482944,14.6854072593997,2.17368854169722));
#17571=CARTESIAN_POINT('Ctrl Pts',(15.483545781832,14.6318171173353,2.11765305577633));
#17572=CARTESIAN_POINT('Ctrl Pts',(15.618108496126,14.5022604497125,2.00915831452887));
#17573=CARTESIAN_POINT('Ctrl Pts',(15.7034661294598,14.417245662525,1.95832579695071));
#17574=CARTESIAN_POINT('Ctrl Pts',(15.8,14.3165490635069,1.93458023611785));
#17575=CARTESIAN_POINT('',(15.8,13.7158451371576,4.53671356284346));
#17576=CARTESIAN_POINT('Ctrl Pts',(15.8,13.7158451371576,4.53671356284347));
#17577=CARTESIAN_POINT('Ctrl Pts',(15.748022181354,13.7614441691838,4.57540619146144));
#17578=CARTESIAN_POINT('Ctrl Pts',(15.6946673265388,13.8104419362193,4.60834637011984));
#17579=CARTESIAN_POINT('Ctrl Pts',(15.5889287876157,13.9127940567891,4.6579180386363));
#17580=CARTESIAN_POINT('Ctrl Pts',(15.5369709165892,13.9655403593053,4.67494478845388));
#17581=CARTESIAN_POINT('Ctrl Pts',(15.4102920065987,14.101143327321,4.69548193961612));
#17582=CARTESIAN_POINT('Ctrl Pts',(15.3183831004355,14.2056426521345,4.69276573315276));
#17583=CARTESIAN_POINT('Ctrl Pts',(15.0640351589826,14.5203021157126,4.60144029184562));
#17584=CARTESIAN_POINT('Ctrl Pts',(14.8841363199283,14.7522725537633,4.51065284133898));
#17585=CARTESIAN_POINT('Ctrl Pts',(14.657256909085,15.0664921537995,4.29087481037367));
#17586=CARTESIAN_POINT('Origin',(15.8,0.,0.));
#17587=CARTESIAN_POINT('Origin',(15.75,0.,0.));
#17588=CARTESIAN_POINT('',(14.657256909085,13.00313230344,8.73666657015347));
#17589=CARTESIAN_POINT('',(15.8,13.0180291077652,6.26395210128207));
#17590=CARTESIAN_POINT('Ctrl Pts',(14.657256909085,13.00313230344,8.73666657015347));
#17591=CARTESIAN_POINT('Ctrl Pts',(14.6763724381384,13.1141488141925,8.53487539574017));
#17592=CARTESIAN_POINT('Ctrl Pts',(14.6998065311113,13.2297711105426,8.307504948367));
#17593=CARTESIAN_POINT('Ctrl Pts',(14.7651359522578,13.4044795231469,7.88604250250778));
#17594=CARTESIAN_POINT('Ctrl Pts',(14.7991842945128,13.4407888928981,7.74885722031068));
#17595=CARTESIAN_POINT('Ctrl Pts',(14.8880411294636,13.4851932372434,7.4789157724344));
#17596=CARTESIAN_POINT('Ctrl Pts',(14.9527298447847,13.4601311411101,7.38057869159978));
#17597=CARTESIAN_POINT('Ctrl Pts',(15.1817050684307,13.3911991258219,6.99362150790972));
#17598=CARTESIAN_POINT('Ctrl Pts',(15.2414935132379,13.3892483247697,6.85706766399487));
#17599=CARTESIAN_POINT('Ctrl Pts',(15.4262634482922,13.294945568639,6.60534106445171));
#17600=CARTESIAN_POINT('Ctrl Pts',(15.4835457818296,13.2612942322572,6.5354878857941));
#17601=CARTESIAN_POINT('Ctrl Pts',(15.6181084961386,13.1716052381211,6.39226804310028));
#17602=CARTESIAN_POINT('Ctrl Pts',(15.7034661294722,13.1064594825804,6.3176524320107));
#17603=CARTESIAN_POINT('Ctrl Pts',(15.8,13.0180291077652,6.26395210128207));
#17604=CARTESIAN_POINT('',(15.8,11.642622304659,8.55310023610356));
#17605=CARTESIAN_POINT('Ctrl Pts',(15.8,11.642622304659,8.55310023610356));
#17606=CARTESIAN_POINT('Ctrl Pts',(15.7480221813541,11.6740328814042,8.60398998850625));
#17607=CARTESIAN_POINT('Ctrl Pts',(15.6946673265388,11.7104534520241,8.65045910276782));
#17608=CARTESIAN_POINT('Ctrl Pts',(15.5889287876158,11.7924776152374,8.72923310580032));
#17609=CARTESIAN_POINT('Ctrl Pts',(15.5369709165892,11.8373807749034,8.76172601103367));
#17610=CARTESIAN_POINT('Ctrl Pts',(15.4102920066149,11.9600005325229,8.82316162406934));
#17611=CARTESIAN_POINT('Ctrl Pts',(15.3183831004502,12.0602246502893,8.85287042548813));
#17612=CARTESIAN_POINT('Ctrl Pts',(15.0640351591008,12.3877046967887,8.86324989111168));
#17613=CARTESIAN_POINT('Ctrl Pts',(14.8841363200439,12.6363765585323,8.84858870232169));
#17614=CARTESIAN_POINT('Ctrl Pts',(14.657256909085,13.00313230344,8.73666657015347));
#17615=CARTESIAN_POINT('Origin',(15.8,0.,0.));
#17616=CARTESIAN_POINT('Origin',(15.75,0.,0.));
#17617=CARTESIAN_POINT('',(14.657256909085,9.66693526506972,12.3272525341113));
#17618=CARTESIAN_POINT('',(15.8,10.4452137610132,9.98016469125221));
#17619=CARTESIAN_POINT('Ctrl Pts',(14.657256909085,9.66693526506972,12.3272525341113));
#17620=CARTESIAN_POINT('Ctrl Pts',(14.6763724381382,9.83487514324392,12.1696437112352));
#17621=CARTESIAN_POINT('Ctrl Pts',(14.6998065311108,10.0150998138711,11.9891308201514));
#17622=CARTESIAN_POINT('Ctrl Pts',(14.7651359522559,10.3114964463889,11.6422840832027));
#17623=CARTESIAN_POINT('Ctrl Pts',(14.7991842945103,10.3884212926728,11.5230333389365));
#17624=CARTESIAN_POINT('Ctrl Pts',(14.8880411294629,10.5140688285991,11.2800254629353));
#17625=CARTESIAN_POINT('Ctrl Pts',(14.9527298447851,10.5206211879139,11.1787567277932));
#17626=CARTESIAN_POINT('Ctrl Pts',(15.1817050684339,10.5746392914499,10.7894374125313));
#17627=CARTESIAN_POINT('Ctrl Pts',(15.2414935132424,10.6149814278139,10.6589641587713));
#17628=CARTESIAN_POINT('Ctrl Pts',(15.4262634482973,10.6030819742843,10.3904167816911));
#17629=CARTESIAN_POINT('Ctrl Pts',(15.4835457818349,10.5926634708524,10.3135836261195));
#17630=CARTESIAN_POINT('Ctrl Pts',(15.6181084961163,10.5516215338708,10.1496580381011));
#17631=CARTESIAN_POINT('Ctrl Pts',(15.7034661294501,10.5127217304364,10.0585632293736));
#17632=CARTESIAN_POINT('Ctrl Pts',(15.8,10.4452137610132,9.98016469125221));
#17633=CARTESIAN_POINT('',(15.8,8.42973848206085,11.7322498653004));
#17634=CARTESIAN_POINT('Ctrl Pts',(15.8,8.42973848206085,11.7322498653004));
#17635=CARTESIAN_POINT('Ctrl Pts',(15.7480221813568,8.44388591742224,11.79035529795));
#17636=CARTESIAN_POINT('Ctrl Pts',(15.6946673265394,8.46416419241759,11.8458046271437));
#17637=CARTESIAN_POINT('Ctrl Pts',(15.5889287876157,8.51783130168368,11.9460700164254));
#17638=CARTESIAN_POINT('Ctrl Pts',(15.5369709165892,8.55049588437244,11.9908484451188));
#17639=CARTESIAN_POINT('Ctrl Pts',(15.4102920066131,8.64812955539648,12.0871687741808));
#17640=CARTESIAN_POINT('Ctrl Pts',(15.3183831004487,8.73426783116772,12.1463944789968));
#17641=CARTESIAN_POINT('Ctrl Pts',(15.0640351590996,9.04251243207698,12.2574628371007));
#17642=CARTESIAN_POINT('Ctrl Pts',(14.8841363200498,9.28354398309004,12.3203630492662));
#17643=CARTESIAN_POINT('Ctrl Pts',(14.657256909085,9.66693526506972,12.3272525341113));
#17644=CARTESIAN_POINT('Origin',(15.8,0.,0.));
#17645=CARTESIAN_POINT('Origin',(15.75,0.,0.));
#17646=CARTESIAN_POINT('',(14.657256909085,5.38447124945594,14.7111611310115));
#17647=CARTESIAN_POINT('',(15.8,6.84994811524973,12.7194492253464));
#17648=CARTESIAN_POINT('Ctrl Pts',(14.657256909085,5.38447124945594,14.7111611310115));
#17649=CARTESIAN_POINT('Ctrl Pts',(14.6763724381383,5.59289536967339,14.6131625093778));
#17650=CARTESIAN_POINT('Ctrl Pts',(14.6998065311112,5.82008076812136,14.4971770340655));
#17651=CARTESIAN_POINT('Ctrl Pts',(14.7651359522584,6.20915225305531,14.2588977812518));
#17652=CARTESIAN_POINT('Ctrl Pts',(14.799184294514,6.31916263594444,14.1692546686358));
#17653=CARTESIAN_POINT('Ctrl Pts',(14.8880411294634,6.51375410718549,13.9769676685644));
#17654=CARTESIAN_POINT('Ctrl Pts',(14.9527298447846,6.55127953136691,13.8826801684932));
#17655=CARTESIAN_POINT('Ctrl Pts',(15.181705068432,6.72296008538512,13.5291080087931));
#17656=CARTESIAN_POINT('Ctrl Pts',(15.2414935132389,6.80164618977777,13.4174869763306));
#17657=CARTESIAN_POINT('Ctrl Pts',(15.4262634482928,6.87331484027241,13.1584061100604));
#17658=CARTESIAN_POINT('Ctrl Pts',(15.4835457818303,6.88714900549683,13.08211394217));
#17659=CARTESIAN_POINT('Ctrl Pts',(15.6181084961339,6.89877159640274,12.9135287874598));
#17660=CARTESIAN_POINT('Ctrl Pts',(15.7034661294676,6.88992552885059,12.814871775685));
#17661=CARTESIAN_POINT('Ctrl Pts',(15.8,6.84994811524973,12.7194492253464));
#17662=CARTESIAN_POINT('',(15.8,4.39169312339699,13.7629651342901));
#17663=CARTESIAN_POINT('Ctrl Pts',(15.8,4.391693123397,13.7629651342901));
#17664=CARTESIAN_POINT('Ctrl Pts',(15.7480221813548,4.3871925678319,13.8225984825995));
#17665=CARTESIAN_POINT('Ctrl Pts',(15.6946673265391,4.3893435683581,13.8816002600415));
#17666=CARTESIAN_POINT('Ctrl Pts',(15.5889287876156,4.40940031310063,13.9935423606787));
#17667=CARTESIAN_POINT('Ctrl Pts',(15.5369709165893,4.42662888187114,14.0462230882418));
#17668=CARTESIAN_POINT('Ctrl Pts',(15.41029200661,4.48971940232603,14.1679996284208));
#17669=CARTESIAN_POINT('Ctrl Pts',(15.3183831004461,4.55334002150981,14.2509448119967));
#17670=CARTESIAN_POINT('Ctrl Pts',(15.064035159032,4.81217604769203,14.4518299178822));
#17671=CARTESIAN_POINT('Ctrl Pts',(14.8841363199712,5.02197344046365,14.5861344199722));
#17672=CARTESIAN_POINT('Ctrl Pts',(14.657256909085,5.38447124945594,14.7111611310115));
#17673=CARTESIAN_POINT('Origin',(15.8,0.,0.));
#17674=CARTESIAN_POINT('Origin',(15.75,0.,0.));
#17675=CARTESIAN_POINT('',(14.657256909085,0.574937672128249,15.6550387777217));
#17676=CARTESIAN_POINT('',(15.8,2.58416182157067,14.2136654476498));
#17677=CARTESIAN_POINT('Ctrl Pts',(14.657256909085,0.574937672128248,15.6550387777217));
#17678=CARTESIAN_POINT('Ctrl Pts',(14.6763724381383,0.803444029323373,15.6262431452139));
#17679=CARTESIAN_POINT('Ctrl Pts',(14.6998065311111,1.05535166589663,15.5861385521169));
#17680=CARTESIAN_POINT('Ctrl Pts',(14.7651359522555,1.49901297545523,15.4797512169063));
#17681=CARTESIAN_POINT('Ctrl Pts',(14.7991842945089,1.63134031219408,15.4284906283848));
#17682=CARTESIAN_POINT('Ctrl Pts',(14.8880411294632,1.87582774976802,15.3057468955349));
#17683=CARTESIAN_POINT('Ctrl Pts',(14.9527298447857,1.94065298884221,15.2276701479787));
#17684=CARTESIAN_POINT('Ctrl Pts',(15.1817050684304,2.21319070454514,14.9444552503138));
#17685=CARTESIAN_POINT('Ctrl Pts',(15.2414935132402,2.32251843283394,14.8626126835097));
#17686=CARTESIAN_POINT('Ctrl Pts',(15.4262634482963,2.47073976049573,14.6383589683605));
#17687=CARTESIAN_POINT('Ctrl Pts',(15.4835457818332,2.50747240989508,14.5700757971041));
#17688=CARTESIAN_POINT('Ctrl Pts',(15.6181084961336,2.57062182851507,14.4133333652788));
#17689=CARTESIAN_POINT('Ctrl Pts',(15.703466129467,2.59269541157921,14.3167713861453));
#17690=CARTESIAN_POINT('Ctrl Pts',(15.8,2.58416182157067,14.2136654476498));
#17691=CARTESIAN_POINT('',(15.8,-0.0762417569101978,14.4464654837189));
#17692=CARTESIAN_POINT('Ctrl Pts',(15.8,-0.0762417569101987,14.4464654837189));
#17693=CARTESIAN_POINT('Ctrl Pts',(15.7480221813551,-0.0989497576662681,
14.5017894200629));
#17694=CARTESIAN_POINT('Ctrl Pts',(15.6946673265391,-0.115136586527329,
14.55856814069));
#17695=CARTESIAN_POINT('Ctrl Pts',(15.5889287876155,-0.130653500227236,
14.6712292799263));
#17696=CARTESIAN_POINT('Ctrl Pts',(15.5369709165891,-0.130547397724572,
14.7266555496972));
#17697=CARTESIAN_POINT('Ctrl Pts',(15.4102920065971,-0.10817576755874,14.8619679647843));
#17698=CARTESIAN_POINT('Ctrl Pts',(15.3183831004339,-0.0733004344332546,
14.9605133746391));
#17699=CARTESIAN_POINT('Ctrl Pts',(15.0640351589857,0.110790343308599,15.2315511945014));
#17700=CARTESIAN_POINT('Ctrl Pts',(14.8841363199342,0.268817147255368,15.4241133261121));
#17701=CARTESIAN_POINT('Ctrl Pts',(14.657256909085,0.574937672128248,15.6550387777217));
#17702=CARTESIAN_POINT('Origin',(15.8,0.,0.));
#17703=CARTESIAN_POINT('Origin',(15.75,0.,0.));
#17704=CARTESIAN_POINT('',(14.657256909085,-4.29087481037367,15.0664921537995));
#17705=CARTESIAN_POINT('',(15.8,-1.93458023611785,14.3165490635069));
#17706=CARTESIAN_POINT('Ctrl Pts',(14.657256909085,-4.29087481037367,15.0664921537995));
#17707=CARTESIAN_POINT('Ctrl Pts',(14.6763724381383,-4.0646540105399,15.1097182275582));
#17708=CARTESIAN_POINT('Ctrl Pts',(14.6998065311111,-3.81268261045262,15.1494202336739));
#17709=CARTESIAN_POINT('Ctrl Pts',(14.7651359522567,-3.35786013639414,15.1853387496715));
#17710=CARTESIAN_POINT('Ctrl Pts',(14.7991842945111,-3.21616896751135,15.1774784288));
#17711=CARTESIAN_POINT('Ctrl Pts',(14.8880411294633,-2.94571769745804,15.1362929749611));
#17712=CARTESIAN_POINT('Ctrl Pts',(14.952729844785,-2.85993818955639,15.0820696759657));
#17713=CARTESIAN_POINT('Ctrl Pts',(15.1817050684315,-2.51322120266002,14.8969350877885));
#17714=CARTESIAN_POINT('Ctrl Pts',(15.2414935132395,-2.3839536102566,14.8528823073182));
#17715=CARTESIAN_POINT('Ctrl Pts',(15.4262634482938,-2.17368854169781,14.6854072594003));
#17716=CARTESIAN_POINT('Ctrl Pts',(15.4835457818316,-2.11765305577666,14.6318171173356));
#17717=CARTESIAN_POINT('Ctrl Pts',(15.6181084961252,-2.00915831452951,14.5022604497133));
#17718=CARTESIAN_POINT('Ctrl Pts',(15.703466129459,-1.9583257969509,14.4172456625258));
#17719=CARTESIAN_POINT('Ctrl Pts',(15.8,-1.93458023611785,14.3165490635069));
#17720=CARTESIAN_POINT('',(15.8,-4.53671356284346,13.7158451371576));
#17721=CARTESIAN_POINT('Ctrl Pts',(15.8,-4.53671356284346,13.7158451371576));
#17722=CARTESIAN_POINT('Ctrl Pts',(15.7480221813549,-4.57540619146074,13.761444169183));
#17723=CARTESIAN_POINT('Ctrl Pts',(15.6946673265391,-4.60834637011968,13.810441936219));
#17724=CARTESIAN_POINT('Ctrl Pts',(15.5889287876154,-4.65791803863646,13.9127940567894));
#17725=CARTESIAN_POINT('Ctrl Pts',(15.5369709165891,-4.6749447884539,13.9655403593054));
#17726=CARTESIAN_POINT('Ctrl Pts',(15.4102920065921,-4.69548193961718,14.1011433273281));
#17727=CARTESIAN_POINT('Ctrl Pts',(15.3183831004293,-4.69276573315053,14.2056426521421));
#17728=CARTESIAN_POINT('Ctrl Pts',(15.0640351589376,-4.60144029182949,14.5203021157682));
#17729=CARTESIAN_POINT('Ctrl Pts',(14.8841363198831,-4.51065284129522,14.7522725538258));
#17730=CARTESIAN_POINT('Ctrl Pts',(14.657256909085,-4.29087481037367,15.0664921537995));
#17731=CARTESIAN_POINT('Origin',(15.8,0.,0.));
#17732=CARTESIAN_POINT('Origin',(15.75,0.,0.));
#17733=CARTESIAN_POINT('',(14.657256909085,-8.73666657015347,13.00313230344));
#17734=CARTESIAN_POINT('',(15.8,-6.26395210128207,13.0180291077652));
#17735=CARTESIAN_POINT('Ctrl Pts',(14.657256909085,-8.73666657015347,13.00313230344));
#17736=CARTESIAN_POINT('Ctrl Pts',(14.6763724381384,-8.53487539574048,13.1141488141923));
#17737=CARTESIAN_POINT('Ctrl Pts',(14.6998065311113,-8.30750494836773,13.2297711105422));
#17738=CARTESIAN_POINT('Ctrl Pts',(14.7651359522579,-7.88604250250723,13.4044795231472));
#17739=CARTESIAN_POINT('Ctrl Pts',(14.7991842945131,-7.74885722031004,13.4407888928982));
#17740=CARTESIAN_POINT('Ctrl Pts',(14.8880411294634,-7.47891577243505,13.4851932372433));
#17741=CARTESIAN_POINT('Ctrl Pts',(14.952729844784,-7.38057869160082,13.4601311411102));
#17742=CARTESIAN_POINT('Ctrl Pts',(15.1817050684321,-6.99362150790738,13.3911991258215));
#17743=CARTESIAN_POINT('Ctrl Pts',(15.241493513237,-6.85706766399776,13.3892483247691));
#17744=CARTESIAN_POINT('Ctrl Pts',(15.4262634482865,-6.60534106445877,13.2949455686422));
#17745=CARTESIAN_POINT('Ctrl Pts',(15.483545781826,-6.53548788579804,13.2612942322595));
#17746=CARTESIAN_POINT('Ctrl Pts',(15.6181084961187,-6.39226804312133,13.1716052381345));
#17747=CARTESIAN_POINT('Ctrl Pts',(15.7034661294532,-6.31765243202127,13.1064594825978));
#17748=CARTESIAN_POINT('Ctrl Pts',(15.8,-6.26395210128207,13.0180291077652));
#17749=CARTESIAN_POINT('',(15.8,-8.55310023610356,11.642622304659));
#17750=CARTESIAN_POINT('Ctrl Pts',(15.8,-8.55310023610356,11.642622304659));
#17751=CARTESIAN_POINT('Ctrl Pts',(15.7480221813554,-8.60398998850506,11.6740328814034));
#17752=CARTESIAN_POINT('Ctrl Pts',(15.6946673265394,-8.65045910276734,11.7104534520236));
#17753=CARTESIAN_POINT('Ctrl Pts',(15.5889287876151,-8.72923310580083,11.792477615238));
#17754=CARTESIAN_POINT('Ctrl Pts',(15.5369709165891,-8.76172601103371,11.8373807749035));
#17755=CARTESIAN_POINT('Ctrl Pts',(15.4102920066095,-8.82316162407197,11.9600005325281));
#17756=CARTESIAN_POINT('Ctrl Pts',(15.3183831004453,-8.8528704254883,12.0602246502956));
#17757=CARTESIAN_POINT('Ctrl Pts',(15.0640351590599,-8.86324989111337,12.3877046968413));
#17758=CARTESIAN_POINT('Ctrl Pts',(14.8841363200047,-8.84858870230231,12.6363765585959));
#17759=CARTESIAN_POINT('Ctrl Pts',(14.657256909085,-8.73666657015347,13.00313230344));
#17760=CARTESIAN_POINT('Origin',(15.8,0.,0.));
#17761=CARTESIAN_POINT('Origin',(15.75,0.,0.));
#17762=CARTESIAN_POINT('',(14.657256909085,-12.3272525341113,9.66693526506972));
#17763=CARTESIAN_POINT('',(15.8,-9.9801646912522,10.4452137610133));
#17764=CARTESIAN_POINT('Ctrl Pts',(14.657256909085,-12.3272525341113,9.66693526506972));
#17765=CARTESIAN_POINT('Ctrl Pts',(14.6763724381383,-12.1696437112339,9.83487514324528));
#17766=CARTESIAN_POINT('Ctrl Pts',(14.6998065311112,-11.989130820148,10.0150998138746));
#17767=CARTESIAN_POINT('Ctrl Pts',(14.7651359522564,-11.6422840832012,10.3114964463897));
#17768=CARTESIAN_POINT('Ctrl Pts',(14.7991842945105,-11.5230333389356,10.3884212926736));
#17769=CARTESIAN_POINT('Ctrl Pts',(14.8880411294634,-11.2800254629345,10.514068828599));
#17770=CARTESIAN_POINT('Ctrl Pts',(14.9527298447854,-11.1787567277925,10.5206211879141));
#17771=CARTESIAN_POINT('Ctrl Pts',(15.1817050684299,-10.7894374125385,10.5746392914487));
#17772=CARTESIAN_POINT('Ctrl Pts',(15.2414935132389,-10.658964158777,10.6149814278134));
#17773=CARTESIAN_POINT('Ctrl Pts',(15.4262634482945,-10.390416781695,10.6030819742848));
#17774=CARTESIAN_POINT('Ctrl Pts',(15.4835457818311,-10.3135836261246,10.5926634708532));
#17775=CARTESIAN_POINT('Ctrl Pts',(15.6181084961506,-10.1496580380588,10.5516215338609));
#17776=CARTESIAN_POINT('Ctrl Pts',(15.7034661294835,-10.0585632293465,10.5127217304131));
#17777=CARTESIAN_POINT('Ctrl Pts',(15.8,-9.9801646912522,10.4452137610133));
#17778=CARTESIAN_POINT('',(15.8,-11.7322498653003,8.42973848206085));
#17779=CARTESIAN_POINT('Ctrl Pts',(15.8,-11.7322498653004,8.42973848206086));
#17780=CARTESIAN_POINT('Ctrl Pts',(15.7480221813559,-11.790355297951,8.4438859174225));
#17781=CARTESIAN_POINT('Ctrl Pts',(15.6946673265394,-11.8458046271437,8.46416419241756));
#17782=CARTESIAN_POINT('Ctrl Pts',(15.5889287876151,-11.946070016426,8.51783130168396));
#17783=CARTESIAN_POINT('Ctrl Pts',(15.5369709165889,-11.990848445119,8.55049588437264));
#17784=CARTESIAN_POINT('Ctrl Pts',(15.4102920065756,-12.0871687742093,8.64812955542542));
#17785=CARTESIAN_POINT('Ctrl Pts',(15.318383100414,-12.1463944790119,8.73426783120985));
#17786=CARTESIAN_POINT('Ctrl Pts',(15.0640351588785,-12.2574628371972,9.0425124323448));
#17787=CARTESIAN_POINT('Ctrl Pts',(14.8841363198405,-12.3203630492726,9.28354398344375));
#17788=CARTESIAN_POINT('Ctrl Pts',(14.657256909085,-12.3272525341113,9.66693526506972));
#17789=CARTESIAN_POINT('Origin',(15.8,0.,0.));
#17790=CARTESIAN_POINT('Origin',(15.75,0.,0.));
#17791=CARTESIAN_POINT('',(14.657256909085,-14.7111611310115,5.38447124945594));
#17792=CARTESIAN_POINT('',(15.8,-12.7194492253464,6.84994811524973));
#17793=CARTESIAN_POINT('Ctrl Pts',(14.657256909085,-14.7111611310115,5.38447124945595));
#17794=CARTESIAN_POINT('Ctrl Pts',(14.6763724381389,-14.6131625093749,5.59289536967964));
#17795=CARTESIAN_POINT('Ctrl Pts',(14.6998065311128,-14.4971770340571,5.8200807681381));
#17796=CARTESIAN_POINT('Ctrl Pts',(14.7651359522601,-14.2588977812484,6.20915225305788));
#17797=CARTESIAN_POINT('Ctrl Pts',(14.7991842945143,-14.1692546686343,6.31916263594739));
#17798=CARTESIAN_POINT('Ctrl Pts',(14.8880411294636,-13.9769676685657,6.51375410718182));
#17799=CARTESIAN_POINT('Ctrl Pts',(14.9527298447806,-13.8826801684986,6.55127953136504));
#17800=CARTESIAN_POINT('Ctrl Pts',(15.1817050684442,-13.5291080087754,6.72296008539242));
#17801=CARTESIAN_POINT('Ctrl Pts',(15.241493513237,-13.4174869763346,6.80164618977413));
#17802=CARTESIAN_POINT('Ctrl Pts',(15.4262634482843,-13.1584061100718,6.87331484027025));
#17803=CARTESIAN_POINT('Ctrl Pts',(15.4835457818224,-13.0821139421803,6.88714900549545));
#17804=CARTESIAN_POINT('Ctrl Pts',(15.6181084961469,-12.9135287874431,6.89877159640481));
#17805=CARTESIAN_POINT('Ctrl Pts',(15.7034661294807,-12.814871775672,6.88992552884512));
#17806=CARTESIAN_POINT('Ctrl Pts',(15.8,-12.7194492253464,6.84994811524973));
#17807=CARTESIAN_POINT('',(15.8,-13.7629651342901,4.39169312339699));
#17808=CARTESIAN_POINT('Ctrl Pts',(15.8,-13.7629651342901,4.39169312339699));
#17809=CARTESIAN_POINT('Ctrl Pts',(15.7480221813558,-13.8225984825983,4.387192567832));
#17810=CARTESIAN_POINT('Ctrl Pts',(15.6946673265393,-13.8816002600413,4.38934356835805));
#17811=CARTESIAN_POINT('Ctrl Pts',(15.5889287876154,-13.993542360679,4.40940031310068));
#17812=CARTESIAN_POINT('Ctrl Pts',(15.5369709165891,-14.046223088242,4.42662888187123));
#17813=CARTESIAN_POINT('Ctrl Pts',(15.4102920065779,-14.1679996284516,4.48971940234203));
#17814=CARTESIAN_POINT('Ctrl Pts',(15.3183831004165,-14.2509448120201,4.55334002154002));
#17815=CARTESIAN_POINT('Ctrl Pts',(15.0640351588442,-14.4518299180306,4.81217604788315));
#17816=CARTESIAN_POINT('Ctrl Pts',(14.8841363197935,-14.5861344200701,5.02197344074748));
#17817=CARTESIAN_POINT('Ctrl Pts',(14.657256909085,-14.7111611310115,5.38447124945594));
#17818=CARTESIAN_POINT('Origin',(15.8,0.,0.));
#17819=CARTESIAN_POINT('Origin',(15.75,0.,0.));
#17820=CARTESIAN_POINT('',(14.657256909085,-15.6550387777217,0.574937672128249));
#17821=CARTESIAN_POINT('',(15.8,-14.2136654476498,2.58416182157067));
#17822=CARTESIAN_POINT('Ctrl Pts',(14.657256909085,-15.6550387777217,0.574937672128249));
#17823=CARTESIAN_POINT('Ctrl Pts',(14.6763724381385,-15.6262431452137,0.803444029325674));
#17824=CARTESIAN_POINT('Ctrl Pts',(14.6998065311114,-15.5861385521163,1.05535166589991));
#17825=CARTESIAN_POINT('Ctrl Pts',(14.7651359522591,-15.4797512169005,1.49901297547856));
#17826=CARTESIAN_POINT('Ctrl Pts',(14.7991842945149,-15.4284906283764,1.63134031221159));
#17827=CARTESIAN_POINT('Ctrl Pts',(14.8880411294635,-15.3057468955348,1.87582774976688));
#17828=CARTESIAN_POINT('Ctrl Pts',(14.9527298447838,-15.2276701479809,1.94065298884041));
#17829=CARTESIAN_POINT('Ctrl Pts',(15.181705068436,-14.9444552503071,2.213190704551));
#17830=CARTESIAN_POINT('Ctrl Pts',(15.2414935132407,-14.8626126835091,2.32251843283411));
#17831=CARTESIAN_POINT('Ctrl Pts',(15.4262634482963,-14.6383589683605,2.47073976049581));
#17832=CARTESIAN_POINT('Ctrl Pts',(15.4835457818331,-14.5700757971043,2.507472409895));
#17833=CARTESIAN_POINT('Ctrl Pts',(15.618108496131,-14.4133333652819,2.57062182851381));
#17834=CARTESIAN_POINT('Ctrl Pts',(15.7034661294645,-14.316771386148,2.59269541157943));
#17835=CARTESIAN_POINT('Ctrl Pts',(15.8,-14.2136654476498,2.58416182157067));
#17836=CARTESIAN_POINT('',(15.8,-14.4464654837189,-0.0762417569101986));
#17837=CARTESIAN_POINT('Ctrl Pts',(15.8,-14.4464654837189,-0.0762417569101976));
#17838=CARTESIAN_POINT('Ctrl Pts',(15.7480221813552,-14.5017894200628,-0.0989497576662283));
#17839=CARTESIAN_POINT('Ctrl Pts',(15.6946673265391,-14.55856814069,-0.115136586527329));
#17840=CARTESIAN_POINT('Ctrl Pts',(15.5889287876155,-14.6712292799262,-0.130653500227226));
#17841=CARTESIAN_POINT('Ctrl Pts',(15.5369709165891,-14.7266555496972,-0.130547397724577));
#17842=CARTESIAN_POINT('Ctrl Pts',(15.4102920065966,-14.8619679647848,-0.108175767558644));
#17843=CARTESIAN_POINT('Ctrl Pts',(15.3183831004334,-14.9605133746397,-0.0733004344328703));
#17844=CARTESIAN_POINT('Ctrl Pts',(15.0640351589848,-15.2315511945023,0.110790343309237));
#17845=CARTESIAN_POINT('Ctrl Pts',(14.8841363199333,-15.424113326113,0.268817147256498));
#17846=CARTESIAN_POINT('Ctrl Pts',(14.657256909085,-15.6550387777217,0.574937672128249));
#17847=CARTESIAN_POINT('Origin',(15.8,0.,0.));
#17848=CARTESIAN_POINT('Origin',(15.75,0.,0.));
#17849=CARTESIAN_POINT('',(14.657256909085,-15.0664921537995,-4.29087481037367));
#17850=CARTESIAN_POINT('',(15.8,-14.3165490635069,-1.93458023611785));
#17851=CARTESIAN_POINT('Ctrl Pts',(14.657256909085,-15.0664921537995,-4.29087481037367));
#17852=CARTESIAN_POINT('Ctrl Pts',(14.6763724381386,-15.109718227559,-4.06465401053565));
#17853=CARTESIAN_POINT('Ctrl Pts',(14.6998065311121,-15.1494202336756,-3.81268261044208));
#17854=CARTESIAN_POINT('Ctrl Pts',(14.765135952259,-15.1853387496716,-3.35786013638255));
#17855=CARTESIAN_POINT('Ctrl Pts',(14.7991842945136,-15.1774784287992,-3.21616896750232));
#17856=CARTESIAN_POINT('Ctrl Pts',(14.8880411294635,-15.1362929749603,-2.94571769745994));
#17857=CARTESIAN_POINT('Ctrl Pts',(14.9527298447828,-15.0820696759676,-2.85993818955902));
#17858=CARTESIAN_POINT('Ctrl Pts',(15.1817050684391,-14.8969350877823,-2.51322120264979));
#17859=CARTESIAN_POINT('Ctrl Pts',(15.2414935132397,-14.8528823073179,-2.38395361025663));
#17860=CARTESIAN_POINT('Ctrl Pts',(15.4262634482939,-14.6854072594002,-2.17368854169763));
#17861=CARTESIAN_POINT('Ctrl Pts',(15.483545781831,-14.6318171173362,-2.11765305577722));
#17862=CARTESIAN_POINT('Ctrl Pts',(15.6181084961287,-14.5022604497099,-2.00915831452651));
#17863=CARTESIAN_POINT('Ctrl Pts',(15.7034661294625,-14.4172456625222,-1.95832579695004));
#17864=CARTESIAN_POINT('Ctrl Pts',(15.8,-14.3165490635069,-1.93458023611785));
#17865=CARTESIAN_POINT('',(15.8,-13.7158451371576,-4.53671356284346));
#17866=CARTESIAN_POINT('Ctrl Pts',(15.8,-13.7158451371576,-4.53671356284346));
#17867=CARTESIAN_POINT('Ctrl Pts',(15.7480221813554,-13.7614441691826,-4.57540619146037));
#17868=CARTESIAN_POINT('Ctrl Pts',(15.694667326539,-13.8104419362191,-4.60834637011974));
#17869=CARTESIAN_POINT('Ctrl Pts',(15.5889287876157,-13.9127940567892,-4.65791803863634));
#17870=CARTESIAN_POINT('Ctrl Pts',(15.5369709165891,-13.9655403593054,-4.67494478845391));
#17871=CARTESIAN_POINT('Ctrl Pts',(15.4102920065913,-14.101143327329,-4.69548193961731));
#17872=CARTESIAN_POINT('Ctrl Pts',(15.3183831004285,-14.2056426521431,-4.69276573315023));
#17873=CARTESIAN_POINT('Ctrl Pts',(15.0640351589399,-14.5203021157653,-4.60144029183033));
#17874=CARTESIAN_POINT('Ctrl Pts',(14.8841363198868,-14.7522725538208,-4.51065284129877));
#17875=CARTESIAN_POINT('Ctrl Pts',(14.657256909085,-15.0664921537995,-4.29087481037367));
#17876=CARTESIAN_POINT('Origin',(15.8,0.,0.));
#17877=CARTESIAN_POINT('Origin',(15.75,0.,0.));
#17878=CARTESIAN_POINT('',(14.657256909085,-13.00313230344,-8.73666657015347));
#17879=CARTESIAN_POINT('',(15.8,-13.0180291077652,-6.26395210128206));
#17880=CARTESIAN_POINT('Ctrl Pts',(14.657256909085,-13.00313230344,-8.73666657015347));
#17881=CARTESIAN_POINT('Ctrl Pts',(14.6763724381383,-13.1141488141921,-8.53487539574091));
#17882=CARTESIAN_POINT('Ctrl Pts',(14.6998065311112,-13.2297711105418,-8.30750494836842));
#17883=CARTESIAN_POINT('Ctrl Pts',(14.7651359522592,-13.404479523151,-7.88604250249817));
#17884=CARTESIAN_POINT('Ctrl Pts',(14.7991842945157,-13.4407888928998,-7.74885722030159));
#17885=CARTESIAN_POINT('Ctrl Pts',(14.8880411294636,-13.4851932372431,-7.47891577243508));
#17886=CARTESIAN_POINT('Ctrl Pts',(14.9527298447833,-13.4601311411105,-7.38057869160189));
#17887=CARTESIAN_POINT('Ctrl Pts',(15.1817050684368,-13.39119912582,-6.99362150789967));
#17888=CARTESIAN_POINT('Ctrl Pts',(15.2414935132409,-13.3892483247688,-6.85706766398949));
#17889=CARTESIAN_POINT('Ctrl Pts',(15.4262634482971,-13.2949455686362,-6.60534106444548));
#17890=CARTESIAN_POINT('Ctrl Pts',(15.4835457818346,-13.2612942322542,-6.53548788578821));
#17891=CARTESIAN_POINT('Ctrl Pts',(15.6181084961093,-13.1716052381403,-6.39226804313223));
#17892=CARTESIAN_POINT('Ctrl Pts',(15.7034661294435,-13.1064594826067,-6.31765243202665));
#17893=CARTESIAN_POINT('Ctrl Pts',(15.8,-13.0180291077652,-6.26395210128207));
#17894=CARTESIAN_POINT('',(15.8,-11.642622304659,-8.55310023610356));
#17895=CARTESIAN_POINT('Ctrl Pts',(15.8,-11.642622304659,-8.55310023610356));
#17896=CARTESIAN_POINT('Ctrl Pts',(15.748022181353,-11.6740328814048,-8.60398998850739));
#17897=CARTESIAN_POINT('Ctrl Pts',(15.6946673265384,-11.7104534520244,-8.65045910276812));
#17898=CARTESIAN_POINT('Ctrl Pts',(15.5889287876162,-11.7924776152371,-8.72923310580004));
#17899=CARTESIAN_POINT('Ctrl Pts',(15.5369709165894,-11.8373807749032,-8.76172601103358));
#17900=CARTESIAN_POINT('Ctrl Pts',(15.4102920066065,-11.960000532531,-8.82316162407342));
#17901=CARTESIAN_POINT('Ctrl Pts',(15.318383100443,-12.0602246502986,-8.85287042548839));
#17902=CARTESIAN_POINT('Ctrl Pts',(15.0640351590301,-12.3877046968796,-8.8632498911146));
#17903=CARTESIAN_POINT('Ctrl Pts',(14.8841363199762,-12.6363765586419,-8.84858870228826));
#17904=CARTESIAN_POINT('Ctrl Pts',(14.657256909085,-13.00313230344,-8.73666657015347));
#17905=CARTESIAN_POINT('Origin',(15.8,0.,0.));
#17906=CARTESIAN_POINT('Origin',(15.75,0.,0.));
#17907=CARTESIAN_POINT('',(14.657256909085,-9.66693526506972,-12.3272525341113));
#17908=CARTESIAN_POINT('',(15.8,-10.4452137610133,-9.9801646912522));
#17909=CARTESIAN_POINT('Ctrl Pts',(14.657256909085,-9.66693526506972,-12.3272525341113));
#17910=CARTESIAN_POINT('Ctrl Pts',(14.6763724381384,-9.83487514324582,-12.1696437112334));
#17911=CARTESIAN_POINT('Ctrl Pts',(14.6998065311114,-10.015099813876,-11.9891308201465));
#17912=CARTESIAN_POINT('Ctrl Pts',(14.7651359522567,-10.3114964463902,-11.6422840832003));
#17913=CARTESIAN_POINT('Ctrl Pts',(14.7991842945106,-10.3884212926739,-11.523033338935));
#17914=CARTESIAN_POINT('Ctrl Pts',(14.8880411294633,-10.5140688285986,-11.2800254629351));
#17915=CARTESIAN_POINT('Ctrl Pts',(14.9527298447848,-10.5206211879141,-11.1787567277935));
#17916=CARTESIAN_POINT('Ctrl Pts',(15.1817050684351,-10.5746392914498,-10.7894374125298));
#17917=CARTESIAN_POINT('Ctrl Pts',(15.2414935132425,-10.6149814278149,-10.6589641587703));
#17918=CARTESIAN_POINT('Ctrl Pts',(15.4262634483023,-10.6030819742836,-10.3904167816842));
#17919=CARTESIAN_POINT('Ctrl Pts',(15.4835457818389,-10.5926634708515,-10.3135836261144));
#17920=CARTESIAN_POINT('Ctrl Pts',(15.6181084961081,-10.551621533873,-10.1496580381114));
#17921=CARTESIAN_POINT('Ctrl Pts',(15.703466129442,-10.5127217304422,-10.0585632293802));
#17922=CARTESIAN_POINT('Ctrl Pts',(15.8,-10.4452137610133,-9.98016469125221));
#17923=CARTESIAN_POINT('',(15.8,-8.42973848206085,-11.7322498653004));
#17924=CARTESIAN_POINT('Ctrl Pts',(15.8,-8.42973848206086,-11.7322498653004));
#17925=CARTESIAN_POINT('Ctrl Pts',(15.7480221813553,-8.44388591742267,-11.7903552979517));
#17926=CARTESIAN_POINT('Ctrl Pts',(15.6946673265394,-8.46416419241757,-11.8458046271437));
#17927=CARTESIAN_POINT('Ctrl Pts',(15.5889287876151,-8.51783130168398,-11.946070016426));
#17928=CARTESIAN_POINT('Ctrl Pts',(15.536970916589,-8.55049588437258,-11.9908484451189));
#17929=CARTESIAN_POINT('Ctrl Pts',(15.4102920065769,-8.64812955542444,-12.0871687742084));
#17930=CARTESIAN_POINT('Ctrl Pts',(15.3183831004154,-8.73426783120814,-12.1463944790113));
#17931=CARTESIAN_POINT('Ctrl Pts',(15.0640351588785,-9.04251243234484,-12.2574628371973));
#17932=CARTESIAN_POINT('Ctrl Pts',(14.8841363198405,-9.28354398344382,-12.3203630492726));
#17933=CARTESIAN_POINT('Ctrl Pts',(14.657256909085,-9.66693526506972,-12.3272525341113));
#17934=CARTESIAN_POINT('Origin',(15.8,0.,0.));
#17935=CARTESIAN_POINT('Origin',(15.75,0.,0.));
#17936=CARTESIAN_POINT('',(14.657256909085,-5.38447124945594,-14.7111611310115));
#17937=CARTESIAN_POINT('',(15.8,-6.84994811524973,-12.7194492253464));
#17938=CARTESIAN_POINT('Ctrl Pts',(14.657256909085,-5.38447124945595,-14.7111611310115));
#17939=CARTESIAN_POINT('Ctrl Pts',(14.6763724381384,-5.59289536967403,-14.6131625093775));
#17940=CARTESIAN_POINT('Ctrl Pts',(14.6998065311115,-5.82008076812493,-14.4971770340638));
#17941=CARTESIAN_POINT('Ctrl Pts',(14.7651359522571,-6.20915225304582,-14.2588977812571));
#17942=CARTESIAN_POINT('Ctrl Pts',(14.7991842945112,-6.31916263593875,-14.1692546686417));
#17943=CARTESIAN_POINT('Ctrl Pts',(14.8880411294635,-6.51375410718485,-13.9769676685645));
#17944=CARTESIAN_POINT('Ctrl Pts',(14.952729844784,-6.55127953136673,-13.8826801684939));
#17945=CARTESIAN_POINT('Ctrl Pts',(15.181705068435,-6.72296008538707,-13.5291080087886));
#17946=CARTESIAN_POINT('Ctrl Pts',(15.2414935132397,-6.80164618977864,-13.4174869763291));
#17947=CARTESIAN_POINT('Ctrl Pts',(15.4262634482948,-6.87331484027296,-13.1584061100578));
#17948=CARTESIAN_POINT('Ctrl Pts',(15.4835457818317,-6.88714900549704,-13.0821139421683));
#17949=CARTESIAN_POINT('Ctrl Pts',(15.618108496136,-6.8987715964028,-12.9135287874573));
#17950=CARTESIAN_POINT('Ctrl Pts',(15.7034661294695,-6.88992552884981,-12.8148717756832));
#17951=CARTESIAN_POINT('Ctrl Pts',(15.8,-6.84994811524973,-12.7194492253464));
#17952=CARTESIAN_POINT('',(15.8,-4.391693123397,-13.7629651342901));
#17953=CARTESIAN_POINT('Ctrl Pts',(15.8,-4.391693123397,-13.7629651342901));
#17954=CARTESIAN_POINT('Ctrl Pts',(15.7480221813555,-4.38719256783197,-13.8225984825987));
#17955=CARTESIAN_POINT('Ctrl Pts',(15.6946673265391,-4.38934356835812,-13.8816002600416));
#17956=CARTESIAN_POINT('Ctrl Pts',(15.5889287876154,-4.40940031310067,-13.993542360679));
#17957=CARTESIAN_POINT('Ctrl Pts',(15.5369709165889,-4.42662888187134,-14.0462230882423));
#17958=CARTESIAN_POINT('Ctrl Pts',(15.4102920065966,-4.48971940233274,-14.1679996284337));
#17959=CARTESIAN_POINT('Ctrl Pts',(15.3183831004327,-4.55334002152343,-14.2509448120073));
#17960=CARTESIAN_POINT('Ctrl Pts',(15.0640351589831,-4.81217604774183,-14.4518299179208));
#17961=CARTESIAN_POINT('Ctrl Pts',(14.8841363199243,-5.02197344053858,-14.586134419998));
#17962=CARTESIAN_POINT('Ctrl Pts',(14.657256909085,-5.38447124945595,-14.7111611310115));
#17963=CARTESIAN_POINT('Origin',(15.8,0.,0.));
#17964=CARTESIAN_POINT('Origin',(15.75,0.,0.));
#17965=CARTESIAN_POINT('',(14.657256909085,-0.57493767212825,-15.6550387777217));
#17966=CARTESIAN_POINT('',(15.8,-2.58416182157067,-14.2136654476498));
#17967=CARTESIAN_POINT('Ctrl Pts',(14.657256909085,-0.57493767212825,-15.6550387777217));
#17968=CARTESIAN_POINT('Ctrl Pts',(14.6763724381382,-0.803444029322114,
-15.6262431452141));
#17969=CARTESIAN_POINT('Ctrl Pts',(14.6998065311109,-1.05535166589373,-15.5861385521174));
#17970=CARTESIAN_POINT('Ctrl Pts',(14.7651359522566,-1.49901297546359,-15.4797512169046));
#17971=CARTESIAN_POINT('Ctrl Pts',(14.7991842945114,-1.63134031220087,-15.4284906283814));
#17972=CARTESIAN_POINT('Ctrl Pts',(14.8880411294633,-1.87582774976806,-15.3057468955348));
#17973=CARTESIAN_POINT('Ctrl Pts',(14.9527298447852,-1.94065298884167,-15.2276701479793));
#17974=CARTESIAN_POINT('Ctrl Pts',(15.1817050684308,-2.21319070454549,-14.9444552503134));
#17975=CARTESIAN_POINT('Ctrl Pts',(15.24149351324,-2.3225184328336,-14.8626126835099));
#17976=CARTESIAN_POINT('Ctrl Pts',(15.4262634482958,-2.47073976049543,-14.6383589683611));
#17977=CARTESIAN_POINT('Ctrl Pts',(15.483545781833,-2.507472409895,-14.5700757971044));
#17978=CARTESIAN_POINT('Ctrl Pts',(15.6181084961295,-2.57062182851311,-14.4133333652836));
#17979=CARTESIAN_POINT('Ctrl Pts',(15.7034661294631,-2.59269541157956,-14.3167713861495));
#17980=CARTESIAN_POINT('Ctrl Pts',(15.8,-2.58416182157067,-14.2136654476498));
#17981=CARTESIAN_POINT('',(15.8,0.0762417569101962,-14.4464654837189));
#17982=CARTESIAN_POINT('Ctrl Pts',(15.8,0.0762417569101968,-14.4464654837189));
#17983=CARTESIAN_POINT('Ctrl Pts',(15.7480221813555,0.0989497576660791,
-14.5017894200625));
#17984=CARTESIAN_POINT('Ctrl Pts',(15.6946673265393,0.115136586527307,-14.5585681406898));
#17985=CARTESIAN_POINT('Ctrl Pts',(15.5889287876154,0.130653500227241,-14.6712292799264));
#17986=CARTESIAN_POINT('Ctrl Pts',(15.5369709165891,0.130547397724574,-14.7266555496972));
#17987=CARTESIAN_POINT('Ctrl Pts',(15.410292006597,0.108175767558706,-14.8619679647844));
#17988=CARTESIAN_POINT('Ctrl Pts',(15.3183831004337,0.0733004344331047,
-14.9605133746394));
#17989=CARTESIAN_POINT('Ctrl Pts',(15.0640351589872,-0.110790343307477,
-15.2315511944997));
#17990=CARTESIAN_POINT('Ctrl Pts',(14.8841363199356,-0.268817147253357,
-15.4241133261106));
#17991=CARTESIAN_POINT('Ctrl Pts',(14.657256909085,-0.57493767212825,-15.6550387777217));
#17992=CARTESIAN_POINT('Origin',(15.8,0.,0.));
#17993=CARTESIAN_POINT('Origin',(15.75,0.,0.));
#17994=CARTESIAN_POINT('',(14.657256909085,4.29087481037367,-15.0664921537995));
#17995=CARTESIAN_POINT('',(15.8,1.93458023611785,-14.3165490635069));
#17996=CARTESIAN_POINT('Ctrl Pts',(14.657256909085,4.29087481037367,-15.0664921537995));
#17997=CARTESIAN_POINT('Ctrl Pts',(14.6763724381383,4.06465401053917,-15.1097182275583));
#17998=CARTESIAN_POINT('Ctrl Pts',(14.6998065311113,3.81268261045103,-15.1494202336741));
#17999=CARTESIAN_POINT('Ctrl Pts',(14.7651359522575,3.35786013638889,-15.1853387496718));
#18000=CARTESIAN_POINT('Ctrl Pts',(14.7991842945124,3.216168967507,-15.1774784287995));
#18001=CARTESIAN_POINT('Ctrl Pts',(14.8880411294634,2.94571769745822,-15.1362929749609));
#18002=CARTESIAN_POINT('Ctrl Pts',(14.9527298447845,2.85993818955692,-15.0820696759661));
#18003=CARTESIAN_POINT('Ctrl Pts',(15.1817050684319,2.51322120265964,-14.8969350877882));
#18004=CARTESIAN_POINT('Ctrl Pts',(15.2414935132387,2.38395361025797,-14.8528823073188));
#18005=CARTESIAN_POINT('Ctrl Pts',(15.4262634482925,2.17368854169906,-14.6854072594014));
#18006=CARTESIAN_POINT('Ctrl Pts',(15.4835457818303,2.11765305577787,-14.6318171173369));
#18007=CARTESIAN_POINT('Ctrl Pts',(15.6181084961299,2.00915831452544,-14.5022604497087));
#18008=CARTESIAN_POINT('Ctrl Pts',(15.7034661294637,1.95832579694974,-14.4172456625209));
#18009=CARTESIAN_POINT('Ctrl Pts',(15.8,1.93458023611785,-14.3165490635069));
#18010=CARTESIAN_POINT('',(15.8,4.53671356284346,-13.7158451371576));
#18011=CARTESIAN_POINT('Ctrl Pts',(15.8,4.53671356284346,-13.7158451371576));
#18012=CARTESIAN_POINT('Ctrl Pts',(15.7480221813544,4.57540619146115,-13.7614441691835));
#18013=CARTESIAN_POINT('Ctrl Pts',(15.694667326539,4.60834637011977,-13.8104419362192));
#18014=CARTESIAN_POINT('Ctrl Pts',(15.5889287876155,4.65791803863639,-13.9127940567893));
#18015=CARTESIAN_POINT('Ctrl Pts',(15.5369709165891,4.67494478845389,-13.9655403593054));
#18016=CARTESIAN_POINT('Ctrl Pts',(15.4102920066053,4.69548193961504,-14.101143327314));
#18017=CARTESIAN_POINT('Ctrl Pts',(15.3183831004414,4.69276573315488,-14.2056426521272));
#18018=CARTESIAN_POINT('Ctrl Pts',(15.0640351590345,4.60144029186426,-14.5203021156484));
#18019=CARTESIAN_POINT('Ctrl Pts',(14.8841363199801,4.51065284138912,-14.7522725536916));
#18020=CARTESIAN_POINT('Ctrl Pts',(14.657256909085,4.29087481037367,-15.0664921537995));
#18021=CARTESIAN_POINT('Origin',(15.8,0.,0.));
#18022=CARTESIAN_POINT('Origin',(15.75,0.,0.));
#18023=CARTESIAN_POINT('',(14.657256909085,8.73666657015347,-13.00313230344));
#18024=CARTESIAN_POINT('',(15.8,6.26395210128206,-13.0180291077652));
#18025=CARTESIAN_POINT('Ctrl Pts',(14.657256909085,8.73666657015347,-13.00313230344));
#18026=CARTESIAN_POINT('Ctrl Pts',(14.6763724381385,8.53487539573899,-13.1141488141932));
#18027=CARTESIAN_POINT('Ctrl Pts',(14.6998065311118,8.30750494836237,-13.229771110545));
#18028=CARTESIAN_POINT('Ctrl Pts',(14.7651359522573,7.88604250251314,-13.4044795231442));
#18029=CARTESIAN_POINT('Ctrl Pts',(14.7991842945111,7.74885722031548,-13.4407888928976));
#18030=CARTESIAN_POINT('Ctrl Pts',(14.8880411294636,7.47891577243524,-13.4851932372429));
#18031=CARTESIAN_POINT('Ctrl Pts',(14.9527298447839,7.3805786916008,-13.4601311411104));
#18032=CARTESIAN_POINT('Ctrl Pts',(15.181705068435,6.99362150790287,-13.3911991258204));
#18033=CARTESIAN_POINT('Ctrl Pts',(15.2414935132393,6.85706766399212,-13.3892483247693));
#18034=CARTESIAN_POINT('Ctrl Pts',(15.4262634482953,6.60534106444771,-13.2949455686372));
#18035=CARTESIAN_POINT('Ctrl Pts',(15.4835457818325,6.53548788579067,-13.2612942322554));
#18036=CARTESIAN_POINT('Ctrl Pts',(15.6181084961243,6.39226804311592,-13.1716052381305));
#18037=CARTESIAN_POINT('Ctrl Pts',(15.7034661294581,6.31765243201851,-13.1064594825933));
#18038=CARTESIAN_POINT('Ctrl Pts',(15.8,6.26395210128206,-13.0180291077652));
#18039=CARTESIAN_POINT('',(15.8,8.55310023610356,-11.642622304659));
#18040=CARTESIAN_POINT('Ctrl Pts',(15.8,8.55310023610356,-11.642622304659));
#18041=CARTESIAN_POINT('Ctrl Pts',(15.7480221813542,8.60398998850618,-11.6740328814041));
#18042=CARTESIAN_POINT('Ctrl Pts',(15.694667326539,8.65045910276766,-11.7104534520239));
#18043=CARTESIAN_POINT('Ctrl Pts',(15.5889287876153,8.72923310580071,-11.7924776152379));
#18044=CARTESIAN_POINT('Ctrl Pts',(15.5369709165891,8.76172601103374,-11.8373807749035));
#18045=CARTESIAN_POINT('Ctrl Pts',(15.4102920066146,8.82316162406948,-11.9600005325232));
#18046=CARTESIAN_POINT('Ctrl Pts',(15.3183831004499,8.85287042548813,-12.0602246502897));
#18047=CARTESIAN_POINT('Ctrl Pts',(15.0640351591031,8.8632498911116,-12.3877046967857));
#18048=CARTESIAN_POINT('Ctrl Pts',(14.884136320048,8.84858870232365,-12.6363765585259));
#18049=CARTESIAN_POINT('Ctrl Pts',(14.657256909085,8.73666657015347,-13.00313230344));
#18050=CARTESIAN_POINT('Origin',(15.8,0.,0.));
#18051=CARTESIAN_POINT('Origin',(15.75,0.,0.));
#18052=CARTESIAN_POINT('',(14.657256909085,12.3272525341113,-9.66693526506972));
#18053=CARTESIAN_POINT('',(15.8,9.9801646912522,-10.4452137610133));
#18054=CARTESIAN_POINT('Ctrl Pts',(14.657256909085,12.3272525341113,-9.66693526506972));
#18055=CARTESIAN_POINT('Ctrl Pts',(14.6763724381382,12.1696437112347,-9.83487514324446));
#18056=CARTESIAN_POINT('Ctrl Pts',(14.699806531111,11.9891308201493,-10.0150998138733));
#18057=CARTESIAN_POINT('Ctrl Pts',(14.7651359522566,11.6422840831999,-10.311496446391));
#18058=CARTESIAN_POINT('Ctrl Pts',(14.7991842945111,11.5230333389337,-10.3884212926745));
#18059=CARTESIAN_POINT('Ctrl Pts',(14.8880411294632,11.2800254629352,-10.5140688285987));
#18060=CARTESIAN_POINT('Ctrl Pts',(14.9527298447846,11.1787567277939,-10.520621187914));
#18061=CARTESIAN_POINT('Ctrl Pts',(15.1817050684329,10.7894374125334,-10.5746392914494));
#18062=CARTESIAN_POINT('Ctrl Pts',(15.2414935132398,10.6589641587761,-10.614981427813));
#18063=CARTESIAN_POINT('Ctrl Pts',(15.4262634482933,10.3904167816966,-10.603081974285));
#18064=CARTESIAN_POINT('Ctrl Pts',(15.483545781831,10.3135836261245,-10.5926634708533));
#18065=CARTESIAN_POINT('Ctrl Pts',(15.6181084961289,10.1496580380854,-10.5516215338674));
#18066=CARTESIAN_POINT('Ctrl Pts',(15.7034661294626,10.0585632293635,-10.5127217304277));
#18067=CARTESIAN_POINT('Ctrl Pts',(15.8,9.98016469125221,-10.4452137610133));
#18068=CARTESIAN_POINT('',(15.8,11.7322498653004,-8.42973848206085));
#18069=CARTESIAN_POINT('Ctrl Pts',(15.8,11.7322498653004,-8.42973848206086));
#18070=CARTESIAN_POINT('Ctrl Pts',(15.7480221813556,11.7903552979513,-8.44388591742258));
#18071=CARTESIAN_POINT('Ctrl Pts',(15.6946673265392,11.8458046271439,-8.46416419241769));
#18072=CARTESIAN_POINT('Ctrl Pts',(15.5889287876152,11.9460700164259,-8.51783130168395));
#18073=CARTESIAN_POINT('Ctrl Pts',(15.5369709165888,11.9908484451191,-8.55049588437278));
#18074=CARTESIAN_POINT('Ctrl Pts',(15.4102920065736,12.0871687742109,-8.64812955542696));
#18075=CARTESIAN_POINT('Ctrl Pts',(15.3183831004117,12.1463944790129,-8.73426783121256));
#18076=CARTESIAN_POINT('Ctrl Pts',(15.0640351588785,12.2574628371973,-9.04251243234485));
#18077=CARTESIAN_POINT('Ctrl Pts',(14.8841363198405,12.3203630492726,-9.28354398344382));
#18078=CARTESIAN_POINT('Ctrl Pts',(14.657256909085,12.3272525341113,-9.66693526506972));
#18079=CARTESIAN_POINT('Origin',(15.8,0.,0.));
#18080=CARTESIAN_POINT('Origin',(15.75,0.,0.));
#18081=CARTESIAN_POINT('',(15.8218384638272,-14.4233723052509,1.76635367265361E-15));
#18082=CARTESIAN_POINT('Origin',(15.8218384638272,0.,0.));
#18083=CARTESIAN_POINT('',(19.5,-10.5,-1.28587913910472E-15));
#18084=CARTESIAN_POINT('',(15.75,-14.5,-1.77573785876366E-15));
#18085=CARTESIAN_POINT('Origin',(19.5,0.,0.));
#18086=CARTESIAN_POINT('Origin',(21.25,0.,0.));
#18087=CARTESIAN_POINT('',(21.,-10.5,-1.28587913910472E-15));
#18088=CARTESIAN_POINT('',(21.25,-10.5,-1.28587913910472E-15));
#18089=CARTESIAN_POINT('Origin',(21.,0.,0.));
#18090=CARTESIAN_POINT('Origin',(15.75,0.,0.));
#18091=CARTESIAN_POINT('',(14.657256909085,14.7111611310115,-5.38447124945595));
#18092=CARTESIAN_POINT('',(15.8,12.7194492253464,-6.84994811524973));
#18093=CARTESIAN_POINT('Ctrl Pts',(14.657256909085,14.7111611310115,-5.38447124945595));
#18094=CARTESIAN_POINT('Ctrl Pts',(14.6763724381386,14.6131625093767,-5.59289536967573));
#18095=CARTESIAN_POINT('Ctrl Pts',(14.6998065311119,14.4971770340621,-5.82008076812812));
#18096=CARTESIAN_POINT('Ctrl Pts',(14.7651359522581,14.258897781254,-6.20915225305041));
#18097=CARTESIAN_POINT('Ctrl Pts',(14.7991842945124,14.169254668639,-6.3191626359417));
#18098=CARTESIAN_POINT('Ctrl Pts',(14.8880411294633,13.9769676685652,-6.51375410718384));
#18099=CARTESIAN_POINT('Ctrl Pts',(14.9527298447829,13.8826801684955,-6.55127953136609));
#18100=CARTESIAN_POINT('Ctrl Pts',(15.1817050684388,13.5291080087829,-6.72296008538962));
#18101=CARTESIAN_POINT('Ctrl Pts',(15.2414935132397,13.4174869763298,-6.80164618977748));
#18102=CARTESIAN_POINT('Ctrl Pts',(15.4262634482914,13.1584061100624,-6.87331484027209));
#18103=CARTESIAN_POINT('Ctrl Pts',(15.4835457818292,13.0821139421714,-6.88714900549669));
#18104=CARTESIAN_POINT('Ctrl Pts',(15.6181084961279,12.9135287874673,-6.89877159640229));
#18105=CARTESIAN_POINT('Ctrl Pts',(15.7034661294619,12.8148717756907,-6.88992552885296));
#18106=CARTESIAN_POINT('Ctrl Pts',(15.8,12.7194492253464,-6.84994811524973));
#18107=CARTESIAN_POINT('',(15.8,13.7629651342901,-4.391693123397));
#18108=CARTESIAN_POINT('Ctrl Pts',(15.8,13.7629651342901,-4.391693123397));
#18109=CARTESIAN_POINT('Ctrl Pts',(15.7480221813554,13.8225984825988,-4.38719256783196));
#18110=CARTESIAN_POINT('Ctrl Pts',(15.694667326539,13.8816002600417,-4.38934356835814));
#18111=CARTESIAN_POINT('Ctrl Pts',(15.5889287876158,13.9935423606786,-4.4094003131006));
#18112=CARTESIAN_POINT('Ctrl Pts',(15.5369709165891,14.046223088242,-4.42662888187122));
#18113=CARTESIAN_POINT('Ctrl Pts',(15.4102920065917,14.1679996284383,-4.48971940233513));
#18114=CARTESIAN_POINT('Ctrl Pts',(15.3183831004289,14.2509448120103,-4.55334002152732));
#18115=CARTESIAN_POINT('Ctrl Pts',(15.064035158936,14.4518299179581,-4.81217604778975));
#18116=CARTESIAN_POINT('Ctrl Pts',(14.8841363198809,14.5861344200219,-5.0219734406079));
#18117=CARTESIAN_POINT('Ctrl Pts',(14.657256909085,14.7111611310115,-5.38447124945595));
#18118=CARTESIAN_POINT('Origin',(15.8,0.,0.));
#18119=CARTESIAN_POINT('Ctrl Pts',(10.0502525316942,9.07904823952839,-1.22955082275859));
#18120=CARTESIAN_POINT('Ctrl Pts',(11.9668350211294,10.626255672559,-2.28040731262864));
#18121=CARTESIAN_POINT('Ctrl Pts',(13.8834175105647,12.1734631055895,-3.33126380249869));
#18122=CARTESIAN_POINT('Ctrl Pts',(15.8,13.7206705386201,-4.38212029236875));
#18123=CARTESIAN_POINT('Ctrl Pts',(10.0502525316942,9.23541522932356,-1.23556639107773));
#18124=CARTESIAN_POINT('Ctrl Pts',(11.9668350211294,10.8110857311875,-2.30170134729121));
#18125=CARTESIAN_POINT('Ctrl Pts',(13.8834175105647,12.3868775190731,-3.36825415935173));
#18126=CARTESIAN_POINT('Ctrl Pts',(15.8,13.962548020937,-4.43438911556521));
#18127=CARTESIAN_POINT('Ctrl Pts',(10.0502525316942,9.54242006948555,-1.29909254545997));
#18128=CARTESIAN_POINT('Ctrl Pts',(11.9668350211294,11.1694737466003,-2.40552260970753));
#18129=CARTESIAN_POINT('Ctrl Pts',(13.8834175105647,12.7961532691502,-3.51235208206864));
#18130=CARTESIAN_POINT('Ctrl Pts',(15.8,14.4232069462649,-4.6187821463162));
#18131=CARTESIAN_POINT('Ctrl Pts',(10.0502525316941,10.0380523375239,-1.61547231497529));
#18132=CARTESIAN_POINT('Ctrl Pts',(11.9668350211294,11.7265860195463,-2.82582698043838));
#18133=CARTESIAN_POINT('Ctrl Pts',(13.8834175105647,13.4155069687334,-4.03604403376329));
#18134=CARTESIAN_POINT('Ctrl Pts',(15.8,15.1040406507558,-5.24639869922638));
#18135=CARTESIAN_POINT('Ctrl Pts',(10.0502525316942,10.3628708264469,-1.92675755961641));
#18136=CARTESIAN_POINT('Ctrl Pts',(11.9668350211294,12.0820376211579,-3.22250341643877));
#18137=CARTESIAN_POINT('Ctrl Pts',(13.8834175105647,13.8004759242586,-4.51903745819411));
#18138=CARTESIAN_POINT('Ctrl Pts',(15.8,15.5196427189696,-5.81478331501647));
#18139=CARTESIAN_POINT('Ctrl Pts',(10.0502525316942,10.5463163022605,-2.13832987737225));
#18140=CARTESIAN_POINT('Ctrl Pts',(11.9668350211294,12.2789538289737,-3.48877307262933));
#18141=CARTESIAN_POINT('Ctrl Pts',(13.8834175105647,14.0115913556869,-4.8392162678864));
#18142=CARTESIAN_POINT('Ctrl Pts',(15.8,15.7442288824001,-6.18965946314348));
#18143=CARTESIAN_POINT('',(10.0502525316942,10.5463163022605,-2.13832987737225));
#18144=CARTESIAN_POINT('',(15.8,13.7206705386201,-4.38212029236875));
#18145=CARTESIAN_POINT('Ctrl Pts',(15.8,13.7206705386201,-4.38212029236875));
#18146=CARTESIAN_POINT('Ctrl Pts',(15.548617912719,13.5237121602493,-4.24557960414941));
#18147=CARTESIAN_POINT('Ctrl Pts',(15.2955018759958,13.3249640154793,-4.1079402696292));
#18148=CARTESIAN_POINT('Ctrl Pts',(15.0417466762032,13.1251225182505,-3.96976145165633));
#18149=CARTESIAN_POINT('Ctrl Pts',(14.7869012710152,12.9244224444144,-3.8309889776992));
#18150=CARTESIAN_POINT('Ctrl Pts',(14.531411198903,12.7226197192327,-3.69167215691655));
#18151=CARTESIAN_POINT('Ctrl Pts',(14.2763854175014,12.5204677360886,-3.55239975640987));
#18152=CARTESIAN_POINT('Ctrl Pts',(14.0169028604353,12.3147829883978,-3.41069346140857));
#18153=CARTESIAN_POINT('Ctrl Pts',(13.7579009635647,12.1087368195378,-3.26903291905456));
#18154=CARTESIAN_POINT('Ctrl Pts',(13.5005478461954,11.9031704882056,-3.12806496166618));
#18155=CARTESIAN_POINT('Ctrl Pts',(13.309996810501,11.7509637547505,-3.02368856803761));
#18156=CARTESIAN_POINT('Ctrl Pts',(13.1203496871979,11.5990211190179,-2.91969243162131));
#18157=CARTESIAN_POINT('Ctrl Pts',(12.9320806449423,11.4476993942222,-2.81634921885376));
#18158=CARTESIAN_POINT('Ctrl Pts',(12.7398362813705,11.2931824947395,-2.71082390290202));
#18159=CARTESIAN_POINT('Ctrl Pts',(12.5465414849355,11.1373617066507,-2.60462118886898));
#18160=CARTESIAN_POINT('Ctrl Pts',(12.3528698198642,10.980602615666,-2.49810765644039));
#18161=CARTESIAN_POINT('Ctrl Pts',(12.1588877119196,10.8235922502235,-2.39142338986208));
#18162=CARTESIAN_POINT('Ctrl Pts',(11.9645275261794,10.6656407015684,-2.28442707498219));
#18163=CARTESIAN_POINT('Ctrl Pts',(11.7704660711024,10.5071588397368,-2.1775164013726));
#18164=CARTESIAN_POINT('Ctrl Pts',(11.5758128991793,10.3481937475419,-2.07027974418958));
#18165=CARTESIAN_POINT('Ctrl Pts',(11.3814602824284,10.188695283085,-1.96312905478021));
#18166=CARTESIAN_POINT('Ctrl Pts',(11.1880912392173,10.0291195021211,-1.85649845736384));
#18167=CARTESIAN_POINT('Ctrl Pts',(10.9918630490256,9.86718424000789,-1.7482912241759));
#18168=CARTESIAN_POINT('Ctrl Pts',(10.7966477335655,9.705169511719,-1.64061939633804));
#18169=CARTESIAN_POINT('Ctrl Pts',(10.6031590586335,9.54359206502118,-1.5339733721044));
#18170=CARTESIAN_POINT('Ctrl Pts',(10.4170476660414,9.38817519823576,-1.43139351779768));
#18171=CARTESIAN_POINT('Ctrl Pts',(10.2325337582959,9.23316336539109,-1.32976299718727));
#18172=CARTESIAN_POINT('Ctrl Pts',(10.0502525316942,9.07904823952839,-1.22955082275859));
#18173=CARTESIAN_POINT('Ctrl Pts',(15.8,13.7206705386201,-4.38212029236875));
#18174=CARTESIAN_POINT('Ctrl Pts',(15.8,13.7291554381927,-4.38395384756931));
#18175=CARTESIAN_POINT('Ctrl Pts',(15.8,13.7376273491274,-4.38582790366735));
#18176=CARTESIAN_POINT('Ctrl Pts',(15.8,13.7460862714518,-4.38774246062322));
#18177=CARTESIAN_POINT('Ctrl Pts',(15.8,13.7545322021969,-4.38969752766812));
#18178=CARTESIAN_POINT('Ctrl Pts',(15.8,13.7629651342901,-4.391693123397));
#18179=CARTESIAN_POINT('Ctrl Pts',(10.0502525316942,8.25473589028142,-3.97495252086484));
#18180=CARTESIAN_POINT('Ctrl Pts',(11.9668350211294,9.40148508750639,-5.45248982387649));
#18181=CARTESIAN_POINT('Ctrl Pts',(13.8834175105647,10.5482342847314,-6.93002712688815));
#18182=CARTESIAN_POINT('Ctrl Pts',(15.8,11.6949834819563,-8.4075644298998));
#18183=CARTESIAN_POINT('Ctrl Pts',(10.0502525316942,8.40159082201817,-4.02899372351995));
#18184=CARTESIAN_POINT('Ctrl Pts',(11.9668350211294,9.57068870058278,-5.52985728348808));
#18185=CARTESIAN_POINT('Ctrl Pts',(13.8834175105647,10.7397728044506,-7.03115572742428));
#18186=CARTESIAN_POINT('Ctrl Pts',(15.8,11.9088706830152,-8.53201928739242));
#18187=CARTESIAN_POINT('Ctrl Pts',(10.0502525316942,8.67393758705161,-4.18428628311195));
#18188=CARTESIAN_POINT('Ctrl Pts',(11.9668350211294,9.87945189609368,-5.73935104252815));
#18189=CARTESIAN_POINT('Ctrl Pts',(13.8834175105647,11.0844841840221,-7.29468404041884));
#18190=CARTESIAN_POINT('Ctrl Pts',(15.8,12.2899984930642,-8.84974879983504));
#18191=CARTESIAN_POINT('Ctrl Pts',(10.0502525316941,9.04754461221301,-4.63834053369693));
#18192=CARTESIAN_POINT('Ctrl Pts',(11.9668350211294,10.2794154126352,-6.31124182863328));
#18193=CARTESIAN_POINT('Ctrl Pts',(13.8834175105647,11.5116939035746,-7.98413616433455));
#18194=CARTESIAN_POINT('Ctrl Pts',(15.8,12.7435647039968,-9.6570374592709));
#18195=CARTESIAN_POINT('Ctrl Pts',(10.0502525316942,9.26027499705532,-5.0347585282786));
#18196=CARTESIAN_POINT('Ctrl Pts',(11.9668350211294,10.4948922896145,-6.79833782460276));
#18197=CARTESIAN_POINT('Ctrl Pts',(13.8834175105647,11.7285731829415,-8.56244161305559));
#18198=CARTESIAN_POINT('Ctrl Pts',(15.8,12.9631904755006,-10.3260209093797));
#18199=CARTESIAN_POINT('Ctrl Pts',(10.0502525316942,9.36936257048691,-5.29266352931554));
#18200=CARTESIAN_POINT('Ctrl Pts',(11.9668350211294,10.5998888833726,-7.11242577089739));
#18201=CARTESIAN_POINT('Ctrl Pts',(13.8834175105647,11.8304151962582,-8.93218801247923));
#18202=CARTESIAN_POINT('Ctrl Pts',(15.8,13.0609415091439,-10.7519502540611));
#18203=CARTESIAN_POINT('',(10.0502525316942,9.36936257048691,-5.29266352931554));
#18204=CARTESIAN_POINT('',(15.8,11.6949834819563,-8.4075644298998));
#18205=CARTESIAN_POINT('Ctrl Pts',(15.8,11.6949834819563,-8.4075644298998));
#18206=CARTESIAN_POINT('Ctrl Pts',(15.5486176029459,11.5498581470164,-8.21684279750606));
#18207=CARTESIAN_POINT('Ctrl Pts',(15.295501252176,11.4033701387254,-8.02452322133575));
#18208=CARTESIAN_POINT('Ctrl Pts',(15.0417457381106,11.256008997669,-7.83135270226724));
#18209=CARTESIAN_POINT('Ctrl Pts',(14.7869002270792,11.1080148725482,-7.63735242672831));
#18210=CARTESIAN_POINT('Ctrl Pts',(14.5314100499567,10.9591402752373,-7.44249371079193));
#18211=CARTESIAN_POINT('Ctrl Pts',(14.2763841657392,10.8099197880111,-7.24756931575073));
#18212=CARTESIAN_POINT('Ctrl Pts',(14.0169020050303,10.658091848795,-7.04923884684408));
#18213=CARTESIAN_POINT('Ctrl Pts',(13.7579005049326,10.505906041498,-6.85084020761633));
#18214=CARTESIAN_POINT('Ctrl Pts',(13.5005477794198,10.3539625665122,-6.65324852970488));
#18215=CARTESIAN_POINT('Ctrl Pts',(13.3099967661951,10.2414594521436,-6.50694623445706));
#18216=CARTESIAN_POINT('Ctrl Pts',(13.1203496652059,10.1290900041791,-6.36108719500251));
#18217=CARTESIAN_POINT('Ctrl Pts',(12.9320806449423,10.0171093135792,-6.21604099337274));
#18218=CARTESIAN_POINT('Ctrl Pts',(12.7398364624418,9.9027642328534,-6.06793224761062));
#18219=CARTESIAN_POINT('Ctrl Pts',(12.5465418490568,9.78738841037906,-5.91877633502142));
#18220=CARTESIAN_POINT('Ctrl Pts',(12.3528703671111,9.67121625884532,-5.76903486398257));
#18221=CARTESIAN_POINT('Ctrl Pts',(12.1588882142736,9.55485775408309,-5.61905319074209));
#18222=CARTESIAN_POINT('Ctrl Pts',(11.9645279828264,9.43770055909591,-5.46848389786619));
#18223=CARTESIAN_POINT('Ctrl Pts',(11.7704664817053,9.32001254164005,-5.31783217681151));
#18224=CARTESIAN_POINT('Ctrl Pts',(11.5758141145056,9.20196619521644,-5.16672176100727));
#18225=CARTESIAN_POINT('Ctrl Pts',(11.3814622995116,9.08338602074528,-5.01552828296685));
#18226=CARTESIAN_POINT('Ctrl Pts',(11.1880940466152,8.96457159711152,-4.86480554216724));
#18227=CARTESIAN_POINT('Ctrl Pts',(10.9918680747371,8.84400125838504,-4.71185532487703));
#18228=CARTESIAN_POINT('Ctrl Pts',(10.7966549511866,8.72318989747891,-4.55938973719067));
#18229=CARTESIAN_POINT('Ctrl Pts',(10.6031684174481,8.60247741697815,-4.40803483976878));
#18230=CARTESIAN_POINT('Ctrl Pts',(10.4170538516967,8.4863641637451,-4.26244666645391));
#18231=CARTESIAN_POINT('Ctrl Pts',(10.232536813699,8.37034275782415,-4.11788655117324));
#18232=CARTESIAN_POINT('Ctrl Pts',(10.0502525316942,8.25473589028142,-3.97495252086484));
#18233=CARTESIAN_POINT('Ctrl Pts',(15.8,11.6949834819563,-8.4075644298998));
#18234=CARTESIAN_POINT('Ctrl Pts',(15.8,11.7024865012679,-8.41193022268479));
#18235=CARTESIAN_POINT('Ctrl Pts',(15.8,11.709964652185,-8.41633052040236));
#18236=CARTESIAN_POINT('Ctrl Pts',(15.8,11.7174179347465,-8.4207653230234));
#18237=CARTESIAN_POINT('Ctrl Pts',(15.8,11.7248463432757,-8.4252346384098));
#18238=CARTESIAN_POINT('Ctrl Pts',(15.8,11.7322498653003,-8.42973848206085));
#18239=CARTESIAN_POINT('Ctrl Pts',(10.0502525316942,6.62239247796684,-6.33125817110613));
#18240=CARTESIAN_POINT('Ctrl Pts',(11.9668350211294,7.25643163809036,-8.09084464143287));
#18241=CARTESIAN_POINT('Ctrl Pts',(13.8834175105647,7.89047079821388,-9.85043111175961));
#18242=CARTESIAN_POINT('Ctrl Pts',(15.8,8.5245099583374,-11.6100175820864));
#18243=CARTESIAN_POINT('Ctrl Pts',(10.0502525316942,6.74536016772826,-6.42803507865412));
#18244=CARTESIAN_POINT('Ctrl Pts',(11.9668350211294,7.39344597705573,-8.21671225999592));
#18245=CARTESIAN_POINT('Ctrl Pts',(13.8834175105647,8.04138429933134,-10.0057987839539));
#18246=CARTESIAN_POINT('Ctrl Pts',(15.8,8.68947010865881,-11.7944759652957));
#18247=CARTESIAN_POINT('Ctrl Pts',(10.0502525316942,6.95639005916885,-6.65988565896846));
#18248=CARTESIAN_POINT('Ctrl Pts',(11.9668350211295,7.62236086025717,-8.51136454012836));
#18249=CARTESIAN_POINT('Ctrl Pts',(13.8834175105647,8.28779124445876,-10.3629488876586));
#18250=CARTESIAN_POINT('Ctrl Pts',(15.8,8.95376204554707,-12.2144277688185));
#18251=CARTESIAN_POINT('Ctrl Pts',(10.0502525316941,7.17140112925238,-7.20716777578593));
#18252=CARTESIAN_POINT('Ctrl Pts',(11.9668350211294,7.82602495118042,-9.17886046565846));
#18253=CARTESIAN_POINT('Ctrl Pts',(13.8834175105647,8.48103967091343,-11.1506718004078));
#18254=CARTESIAN_POINT('Ctrl Pts',(15.8,9.13566349284146,-13.1223644902804));
#18255=CARTESIAN_POINT('Ctrl Pts',(10.0502525316942,7.25121893082227,-7.64992225296746));
#18256=CARTESIAN_POINT('Ctrl Pts',(11.9668350211294,7.88043377854935,-9.70870355968973));
#18257=CARTESIAN_POINT('Ctrl Pts',(13.8834175105647,8.50859598070372,-11.7676943247925));
#18258=CARTESIAN_POINT('Ctrl Pts',(15.8,9.13781082843079,-13.8264756315147));
#18259=CARTESIAN_POINT('Ctrl Pts',(10.0502525316942,7.27527035012649,-7.92891439885425));
#18260=CARTESIAN_POINT('Ctrl Pts',(11.9668350211294,7.88323296009842,-10.0398646795257));
#18261=CARTESIAN_POINT('Ctrl Pts',(13.8834175105647,8.49119557007034,-12.1508149601973));
#18262=CARTESIAN_POINT('Ctrl Pts',(15.8,9.09915818004226,-14.2617652408688));
#18263=CARTESIAN_POINT('',(10.0502525316942,7.27527035012649,-7.92891439885425));
#18264=CARTESIAN_POINT('',(15.8,8.5245099583374,-11.6100175820864));
#18265=CARTESIAN_POINT('Ctrl Pts',(15.8,8.5245099583374,-11.6100175820864));
#18266=CARTESIAN_POINT('Ctrl Pts',(15.5486176754283,8.44542381127122,-11.3837844012201));
#18267=CARTESIAN_POINT('Ctrl Pts',(15.2955013981408,8.36553547761206,-11.1556103968136));
#18268=CARTESIAN_POINT('Ctrl Pts',(15.0417459576106,8.28507970174558,-10.9263572847368));
#18269=CARTESIAN_POINT('Ctrl Pts',(14.7869004713578,8.20427831565627,-10.696119380477));
#18270=CARTESIAN_POINT('Ctrl Pts',(14.531410318819,8.12290482377608,-10.4647929695858));
#18271=CARTESIAN_POINT('Ctrl Pts',(14.2763844586717,8.0412226669247,-10.2332972079364));
#18272=CARTESIAN_POINT('Ctrl Pts',(14.0169022052172,7.95811317318716,-9.99775622451133));
#18273=CARTESIAN_POINT('Ctrl Pts',(13.7579006122767,7.87468439208872,-9.76203981942054));
#18274=CARTESIAN_POINT('Ctrl Pts',(13.5005477950714,7.79123671760748,-9.52716576584172));
#18275=CARTESIAN_POINT('Ctrl Pts',(13.30999677658,7.72944979203263,-9.35325863471847));
#18276=CARTESIAN_POINT('Ctrl Pts',(13.1203496703607,7.66765301700974,-9.1798143702817));
#18277=CARTESIAN_POINT('Ctrl Pts',(12.9320806449423,7.605974791296,-9.00726329348628));
#18278=CARTESIAN_POINT('Ctrl Pts',(12.7398364200678,7.54299426293975,-8.83106889328651));
#18279=CARTESIAN_POINT('Ctrl Pts',(12.5465417638457,7.47935703277434,-8.65356006118378));
#18280=CARTESIAN_POINT('Ctrl Pts',(12.3528702390454,7.41514339569062,-8.47524825078843));
#18281=CARTESIAN_POINT('Ctrl Pts',(12.1588880967136,7.35082677040844,-8.29665045733793));
#18282=CARTESIAN_POINT('Ctrl Pts',(11.9645278759626,7.28593212986481,-8.11724699610014));
#18283=CARTESIAN_POINT('Ctrl Pts',(11.7704663856167,7.22055811872365,-7.9376011083099));
#18284=CARTESIAN_POINT('Ctrl Pts',(11.5758138300784,7.15498499387682,-7.75740806182766));
#18285=CARTESIAN_POINT('Ctrl Pts',(11.3814618274401,7.08892983490276,-7.57697105649293));
#18286=CARTESIAN_POINT('Ctrl Pts',(11.1880933895773,7.02250642528014,-7.39690936354705));
#18287=CARTESIAN_POINT('Ctrl Pts',(10.99186689856,6.95510125442749,-7.21418629579141));
#18288=CARTESIAN_POINT('Ctrl Pts',(10.7966532620494,6.88731709712089,-7.03184966122165));
#18289=CARTESIAN_POINT('Ctrl Pts',(10.6031662272196,6.81928375787422,-6.85059991984744));
#18290=CARTESIAN_POINT('Ctrl Pts',(10.4170524040777,6.75384296552633,-6.67625706354029));
#18291=CARTESIAN_POINT('Ctrl Pts',(10.2325360986479,6.68817184019669,-6.50292032538242));
#18292=CARTESIAN_POINT('Ctrl Pts',(10.0502525316942,6.62239247796684,-6.33125817110613));
#18293=CARTESIAN_POINT('Ctrl Pts',(15.8,8.5245099583374,-11.6100175820864));
#18294=CARTESIAN_POINT('Ctrl Pts',(15.8,8.53029664958107,-11.6164882582397));
#18295=CARTESIAN_POINT('Ctrl Pts',(15.8,8.53604902696561,-11.6229840657775));
#18296=CARTESIAN_POINT('Ctrl Pts',(15.8,8.54176709053684,-11.6295050046841));
#18297=CARTESIAN_POINT('Ctrl Pts',(15.8,8.54745083246671,-11.6360510806824));
#18298=CARTESIAN_POINT('Ctrl Pts',(15.8,8.55310023610356,-11.642622304659));
#18299=CARTESIAN_POINT('Ctrl Pts',(10.0502525316942,4.34180314898733,-8.06781615908999));
#18300=CARTESIAN_POINT('Ctrl Pts',(11.9668350211294,4.40106810140592,-9.93721121325641));
#18301=CARTESIAN_POINT('Ctrl Pts',(13.8834175105647,4.46033305382451,-11.8066062674228));
#18302=CARTESIAN_POINT('Ctrl Pts',(15.8,4.51959800624309,-13.6760013215893));
#18303=CARTESIAN_POINT('Ctrl Pts',(10.0502525316942,4.4288466625333,-8.19785557353568));
#18304=CARTESIAN_POINT('Ctrl Pts',(11.9668350211294,4.49248124812732,-10.0992581912947));
#18305=CARTESIAN_POINT('Ctrl Pts',(13.8834175105647,4.55584907137465,-12.0010045410108));
#18306=CARTESIAN_POINT('Ctrl Pts',(15.8,4.61948365696867,-13.9024071587698));
#18307=CARTESIAN_POINT('Ctrl Pts',(10.0502525316942,4.55790932427761,-8.48356457498289));
#18308=CARTESIAN_POINT('Ctrl Pts',(11.9668350211294,4.61914675531023,-10.4502219249867));
#18309=CARTESIAN_POINT('Ctrl Pts',(13.8834175105647,4.67984453466857,-12.416810143598));
#18310=CARTESIAN_POINT('Ctrl Pts',(15.8,4.74108196570119,-14.3834674936017));
#18311=CARTESIAN_POINT('Ctrl Pts',(10.0502525316941,4.59327853800038,-9.07050287838802));
#18312=CARTESIAN_POINT('Ctrl Pts',(11.9668350211294,4.60657624071161,-11.1479839451212));
#18313=CARTESIAN_POINT('Ctrl Pts',(13.8834175105647,4.62021662092399,-13.2256962639304));
#18314=CARTESIAN_POINT('Ctrl Pts',(15.8,4.63351432363523,-15.3031773306636));
#18315=CARTESIAN_POINT('Ctrl Pts',(10.0502525316942,4.5323630334273,-9.51625828739342));
#18316=CARTESIAN_POINT('Ctrl Pts',(11.9668350211294,4.49458350302914,-11.668713745839));
#18317=CARTESIAN_POINT('Ctrl Pts',(13.8834175105647,4.45573812100051,-13.8210431256713));
#18318=CARTESIAN_POINT('Ctrl Pts',(15.8,4.41795859060236,-15.9734985841168));
#18319=CARTESIAN_POINT('Ctrl Pts',(10.0502525316942,4.46902397810654,-9.78902788303806));
#18320=CARTESIAN_POINT('Ctrl Pts',(11.9668350211294,4.39491126897609,-11.9845316814717));
#18321=CARTESIAN_POINT('Ctrl Pts',(13.8834175105647,4.32079855984563,-14.1800354799052));
#18322=CARTESIAN_POINT('Ctrl Pts',(15.8,4.24668585071518,-16.3755392783388));
#18323=CARTESIAN_POINT('',(10.0502525316942,4.46902397810654,-9.78902788303806));
#18324=CARTESIAN_POINT('',(15.8,4.51959800624309,-13.6760013215893));
#18325=CARTESIAN_POINT('Ctrl Pts',(15.8,4.51959800624309,-13.6760013215893));
#18326=CARTESIAN_POINT('Ctrl Pts',(15.5486181428678,4.51429251817175,-13.4364022627908));
#18327=CARTESIAN_POINT('Ctrl Pts',(15.2955023394683,4.50882385781799,-13.1947094870259));
#18328=CARTESIAN_POINT('Ctrl Pts',(15.0417473731674,4.50314899406868,-12.9518150706376));
#18329=CARTESIAN_POINT('Ctrl Pts',(14.7869020465192,4.49744974598318,-12.7078769606258));
#18330=CARTESIAN_POINT('Ctrl Pts',(14.5314120523271,4.49154276300949,-12.4627268269524));
#18331=CARTESIAN_POINT('Ctrl Pts',(14.2763863472162,4.48539455472627,-12.2173202460906));
#18332=CARTESIAN_POINT('Ctrl Pts',(14.0169034957089,4.4791388927086,-11.9676246346112));
#18333=CARTESIAN_POINT('Ctrl Pts',(13.7579013040888,4.47263377735531,-11.7176635180578));
#18334=CARTESIAN_POINT('Ctrl Pts',(13.5005478956223,4.46585038850025,-11.4684976917997));
#18335=CARTESIAN_POINT('Ctrl Pts',(13.3099968432959,4.46082779372533,-11.2840089349569));
#18336=CARTESIAN_POINT('Ctrl Pts',(13.1203497034762,4.45565279642652,-11.0999573476245));
#18337=CARTESIAN_POINT('Ctrl Pts',(12.9320806449423,4.45031453415308,-10.9167918673754));
#18338=CARTESIAN_POINT('Ctrl Pts',(12.7398361468871,4.44486355054889,-10.729758713411));
#18339=CARTESIAN_POINT('Ctrl Pts',(12.5465412144991,4.43919418585341,-10.5412725252545));
#18340=CARTESIAN_POINT('Ctrl Pts',(12.3528694134188,4.4332247563449,-10.3518445394593));
#18341=CARTESIAN_POINT('Ctrl Pts',(12.1588873388164,4.42724576346212,-10.1621130789817));
#18342=CARTESIAN_POINT('Ctrl Pts',(11.9645271870233,4.42096600829023,-9.97143676938844));
#18343=CARTESIAN_POINT('Ctrl Pts',(11.7704657661435,4.41430525673782,-9.78038176737572));
#18344=CARTESIAN_POINT('Ctrl Pts',(11.5758119966791,4.4076241740617,-9.58874359350173));
#18345=CARTESIAN_POINT('Ctrl Pts',(11.3814587845899,4.40056003028008,-9.39672444178994));
#18346=CARTESIAN_POINT('Ctrl Pts',(11.1880891545369,4.39302967416939,-9.20494844642816));
#18347=CARTESIAN_POINT('Ctrl Pts',(10.9918593168755,4.3853879335469,-9.01033581554672));
#18348=CARTESIAN_POINT('Ctrl Pts',(10.796642373555,4.37726632301398,-8.81597360566157));
#18349=CARTESIAN_POINT('Ctrl Pts',(10.6031521084281,4.36857183761346,-8.62256814054944));
#18350=CARTESIAN_POINT('Ctrl Pts',(10.4170430723424,4.36020902775276,-8.43654066954402));
#18351=CARTESIAN_POINT('Ctrl Pts',(10.2325314892389,4.35131627654661,-8.25139886794601));
#18352=CARTESIAN_POINT('Ctrl Pts',(10.0502525316942,4.34180314898733,-8.06781615908999));
#18353=CARTESIAN_POINT('Ctrl Pts',(15.8,4.51959800624309,-13.6760013215893));
#18354=CARTESIAN_POINT('Ctrl Pts',(15.8,4.52310192776169,-13.6839434862452));
#18355=CARTESIAN_POINT('Ctrl Pts',(15.8,4.52656544883607,-13.6918989487026));
#18356=CARTESIAN_POINT('Ctrl Pts',(15.8,4.52998856951466,-13.6998677089605));
#18357=CARTESIAN_POINT('Ctrl Pts',(15.8,4.53337128058405,-13.7078497700428));
#18358=CARTESIAN_POINT('Ctrl Pts',(15.8,4.53671356284346,-13.7158451371576));
#18359=CARTESIAN_POINT('Ctrl Pts',(10.0502525316942,1.6362078766636,-9.01464008964162));
#18360=CARTESIAN_POINT('Ctrl Pts',(11.9668350211294,1.11489735491132,-10.8108543149047));
#18361=CARTESIAN_POINT('Ctrl Pts',(13.8834175105647,0.593586833159036,-12.6070685401678));
#18362=CARTESIAN_POINT('Ctrl Pts',(15.8,0.0722763114067552,-14.4032827654308));
#18363=CARTESIAN_POINT('Ctrl Pts',(10.0502525316942,1.67880678842043,-9.16521284706123));
#18364=CARTESIAN_POINT('Ctrl Pts',(11.9668350211294,1.15176115367482,-10.9932183651601));
#18365=CARTESIAN_POINT('Ctrl Pts',(13.8834175105647,0.624355593844835,-12.8214683576781));
#18366=CARTESIAN_POINT('Ctrl Pts',(15.8,0.0973099590992221,-14.6494738757771));
#18367=CARTESIAN_POINT('Ctrl Pts',(10.0502525316942,1.71327315824379,-9.47681709721301));
#18368=CARTESIAN_POINT('Ctrl Pts',(11.9668350211294,1.16378287280497,-11.3661427921348));
#18369=CARTESIAN_POINT('Ctrl Pts',(13.8834175105647,0.613808798404413,-13.2552357701884));
#18370=CARTESIAN_POINT('Ctrl Pts',(15.8,0.064318512965595,-15.1445614651102));
#18371=CARTESIAN_POINT('Ctrl Pts',(10.0502525316941,1.56553830329485,-10.0459586957056));
#18372=CARTESIAN_POINT('Ctrl Pts',(11.9668350211294,0.936208214997359,-12.025869817826));
#18373=CARTESIAN_POINT('Ctrl Pts',(13.8834175105647,0.307141231238404,-14.0061068566225));
#18374=CARTESIAN_POINT('Ctrl Pts',(15.8,-0.322188857059085,-15.9860179787428));
#18375=CARTESIAN_POINT('Ctrl Pts',(10.0502525316942,1.36984786349029,-10.4510766569791));
#18376=CARTESIAN_POINT('Ctrl Pts',(11.9668350211294,0.668772078627757,-12.4865089298363));
#18377=CARTESIAN_POINT('Ctrl Pts',(13.8834175105647,-0.0332784309391876,
-14.5214919285394));
#18378=CARTESIAN_POINT('Ctrl Pts',(15.8,-0.734354215801725,-16.5569242013966));
#18379=CARTESIAN_POINT('Ctrl Pts',(10.0502525316942,1.22531840158854,-10.6909231138624));
#18380=CARTESIAN_POINT('Ctrl Pts',(11.9668350211294,0.476385041699009,-12.7560692212929));
#18381=CARTESIAN_POINT('Ctrl Pts',(13.8834175105647,-0.272548318190526,
-14.8212153287235));
#18382=CARTESIAN_POINT('Ctrl Pts',(15.8,-1.02148167808006,-16.886361436154));
#18383=CARTESIAN_POINT('',(10.0502525316942,1.22531840158854,-10.6909231138624));
#18384=CARTESIAN_POINT('',(15.8,0.0722763114067552,-14.4032827654308));
#18385=CARTESIAN_POINT('Ctrl Pts',(15.8,0.0722763114067553,-14.4032827654308));
#18386=CARTESIAN_POINT('Ctrl Pts',(15.5486186601036,0.141270531448607,-14.1737715055214));
#18387=CARTESIAN_POINT('Ctrl Pts',(15.2955033810753,0.210756563075219,-13.9422185866342));
#18388=CARTESIAN_POINT('Ctrl Pts',(15.0417489395233,0.280417814421832,-13.7094591215782));
#18389=CARTESIAN_POINT('Ctrl Pts',(14.7869037890756,0.35037848967631,-13.4756991900179));
#18390=CARTESIAN_POINT('Ctrl Pts',(14.5314139696902,0.42051613703443,-13.2407223608425));
#18391=CARTESIAN_POINT('Ctrl Pts',(14.2763884357263,0.490503613096802,-13.005427090821));
#18392=CARTESIAN_POINT('Ctrl Pts',(14.0169049225921,0.561714506695558,-12.7660187369198));
#18393=CARTESIAN_POINT('Ctrl Pts',(13.7579020686525,0.632770201645049,-12.5262807827892));
#18394=CARTESIAN_POINT('Ctrl Pts',(13.5005480060748,0.703315478824952,-12.2872132071322));
#18395=CARTESIAN_POINT('Ctrl Pts',(13.3099969165817,0.755548885558801,-12.1102018689483));
#18396=CARTESIAN_POINT('Ctrl Pts',(13.1203497398528,0.807502254261702,-11.9335592090234));
#18397=CARTESIAN_POINT('Ctrl Pts',(12.9320806449423,0.859026524117212,-11.7577088361878));
#18398=CARTESIAN_POINT('Ctrl Pts',(12.7398358447889,0.911638839304298,-11.578145006029));
#18399=CARTESIAN_POINT('Ctrl Pts',(12.5465406070012,0.964492472594393,-11.3971317706528));
#18400=CARTESIAN_POINT('Ctrl Pts',(12.3528685003953,1.0173517555332,-11.215130105891));
#18401=CARTESIAN_POINT('Ctrl Pts',(12.1588865006919,1.07029561816294,-11.0328372218068));
#18402=CARTESIAN_POINT('Ctrl Pts',(11.9645264251562,1.12324541000608,-10.8495527946017));
#18403=CARTESIAN_POINT('Ctrl Pts',(11.7704650810958,1.17594987240342,-10.66579047727));
#18404=CARTESIAN_POINT('Ctrl Pts',(11.575809969755,1.22881559404307,-10.4814659044725));
#18405=CARTESIAN_POINT('Ctrl Pts',(11.3814554207367,1.28143472519663,-10.2966606229241));
#18406=CARTESIAN_POINT('Ctrl Pts',(11.188084472835,1.33353531202393,-10.1119425360162));
#18407=CARTESIAN_POINT('Ctrl Pts',(10.9918509346328,1.38640717621279,-9.92448995248599));
#18408=CARTESIAN_POINT('Ctrl Pts',(10.7966303348178,1.43874524883781,-9.73712725458209));
#18409=CARTESIAN_POINT('Ctrl Pts',(10.6031364978011,1.49024279648084,-9.5504974919454));
#18410=CARTESIAN_POINT('Ctrl Pts',(10.4170327545854,1.5397735026292,-9.37099566409577));
#18411=CARTESIAN_POINT('Ctrl Pts',(10.2325263927829,1.58852655489966,-9.19217237538429));
#18412=CARTESIAN_POINT('Ctrl Pts',(10.0502525316942,1.6362078766636,-9.01464008964162));
#18413=CARTESIAN_POINT('Ctrl Pts',(15.8,0.0722763114067552,-14.4032827654308));
#18414=CARTESIAN_POINT('Ctrl Pts',(15.8,0.07315447494878,-14.4119189841766));
#18415=CARTESIAN_POINT('Ctrl Pts',(15.8,0.073990106138469,-14.4205553654592));
#18416=CARTESIAN_POINT('Ctrl Pts',(15.8,0.0747832050221156,-14.4291919092927));
#18417=CARTESIAN_POINT('Ctrl Pts',(15.8,0.0755337619028261,-14.437828615706));
#18418=CARTESIAN_POINT('Ctrl Pts',(15.8,0.0762417569101966,-14.4464654837189));
#18419=CARTESIAN_POINT('Ctrl Pts',(10.0502525316942,-1.22955082275859,-9.07904823952839));
#18420=CARTESIAN_POINT('Ctrl Pts',(11.9668350211294,-2.28040731262864,-10.626255672559));
#18421=CARTESIAN_POINT('Ctrl Pts',(13.8834175105647,-3.33126380249869,-12.1734631055895));
#18422=CARTESIAN_POINT('Ctrl Pts',(15.8,-4.38212029236875,-13.7206705386201));
#18423=CARTESIAN_POINT('Ctrl Pts',(10.0502525316942,-1.23556639107773,-9.23541522932356));
#18424=CARTESIAN_POINT('Ctrl Pts',(11.9668350211294,-2.3017013472912,-10.8110857311875));
#18425=CARTESIAN_POINT('Ctrl Pts',(13.8834175105647,-3.36825415935173,-12.3868775190731));
#18426=CARTESIAN_POINT('Ctrl Pts',(15.8,-4.43438911556521,-13.962548020937));
#18427=CARTESIAN_POINT('Ctrl Pts',(10.0502525316942,-1.29909254545997,-9.54242006948553));
#18428=CARTESIAN_POINT('Ctrl Pts',(11.9668350211294,-2.40552260970754,-11.1694737466002));
#18429=CARTESIAN_POINT('Ctrl Pts',(13.8834175105647,-3.51235208206866,-12.7961532691502));
#18430=CARTESIAN_POINT('Ctrl Pts',(15.8,-4.61878214631622,-14.4232069462649));
#18431=CARTESIAN_POINT('Ctrl Pts',(10.0502525316941,-1.6154723149753,-10.0380523375239));
#18432=CARTESIAN_POINT('Ctrl Pts',(11.9668350211294,-2.82582698043839,-11.7265860195463));
#18433=CARTESIAN_POINT('Ctrl Pts',(13.8834175105647,-4.03604403376329,-13.4155069687333));
#18434=CARTESIAN_POINT('Ctrl Pts',(15.8,-5.24639869922639,-15.1040406507558));
#18435=CARTESIAN_POINT('Ctrl Pts',(10.0502525316942,-1.92675755961641,-10.3628708264469));
#18436=CARTESIAN_POINT('Ctrl Pts',(11.9668350211294,-3.22250341643877,-12.0820376211579));
#18437=CARTESIAN_POINT('Ctrl Pts',(13.8834175105647,-4.51903745819409,-13.8004759242586));
#18438=CARTESIAN_POINT('Ctrl Pts',(15.8,-5.81478331501644,-15.5196427189696));
#18439=CARTESIAN_POINT('Ctrl Pts',(10.0502525316942,-2.13832987737225,-10.5463163022605));
#18440=CARTESIAN_POINT('Ctrl Pts',(11.9668350211294,-3.48877307262933,-12.2789538289737));
#18441=CARTESIAN_POINT('Ctrl Pts',(13.8834175105647,-4.8392162678864,-14.0115913556869));
#18442=CARTESIAN_POINT('Ctrl Pts',(15.8,-6.18965946314348,-15.7442288824001));
#18443=CARTESIAN_POINT('',(10.0502525316942,-2.13832987737225,-10.5463163022605));
#18444=CARTESIAN_POINT('',(15.8,-4.38212029236875,-13.7206705386201));
#18445=CARTESIAN_POINT('Ctrl Pts',(15.8,-4.38212029236875,-13.7206705386201));
#18446=CARTESIAN_POINT('Ctrl Pts',(15.5486179127196,-4.24557960414972,-13.5237121602497));
#18447=CARTESIAN_POINT('Ctrl Pts',(15.295501875997,-4.10794026962981,-13.3249640154802));
#18448=CARTESIAN_POINT('Ctrl Pts',(15.0417466762049,-3.96976145165723,-13.1251225182518));
#18449=CARTESIAN_POINT('Ctrl Pts',(14.7869012710178,-3.83098897770061,-12.9244224444165));
#18450=CARTESIAN_POINT('Ctrl Pts',(14.5314111989065,-3.69167215691846,-12.7226197192354));
#18451=CARTESIAN_POINT('Ctrl Pts',(14.2763854175058,-3.55239975641227,-12.5204677360921));
#18452=CARTESIAN_POINT('Ctrl Pts',(14.0169028604397,-3.41069346141101,-12.3147829884013));
#18453=CARTESIAN_POINT('Ctrl Pts',(13.7579009635692,-3.26903291905704,-12.1087368195414));
#18454=CARTESIAN_POINT('Ctrl Pts',(13.5005478461999,-3.12806496166868,-11.9031704882092));
#18455=CARTESIAN_POINT('Ctrl Pts',(13.309996810504,-3.02368856803927,-11.750963754753));
#18456=CARTESIAN_POINT('Ctrl Pts',(13.1203496871994,-2.91969243162214,-11.5990211190191));
#18457=CARTESIAN_POINT('Ctrl Pts',(12.9320806449423,-2.81634921885376,-11.4476993942222));
#18458=CARTESIAN_POINT('Ctrl Pts',(12.7398362813702,-2.71082390290183,-11.2931824947393));
#18459=CARTESIAN_POINT('Ctrl Pts',(12.5465414849348,-2.6046211888686,-11.1373617066502));
#18460=CARTESIAN_POINT('Ctrl Pts',(12.3528698198632,-2.49810765643983,-10.9806026156652));
#18461=CARTESIAN_POINT('Ctrl Pts',(12.1588877119187,-2.39142338986155,-10.8235922502227));
#18462=CARTESIAN_POINT('Ctrl Pts',(11.9645275261786,-2.28442707498171,-10.6656407015677));
#18463=CARTESIAN_POINT('Ctrl Pts',(11.7704660711016,-2.17751640137217,-10.5071588397361));
#18464=CARTESIAN_POINT('Ctrl Pts',(11.5758128991787,-2.07027974418926,-10.3481937475414));
#18465=CARTESIAN_POINT('Ctrl Pts',(11.3814602824281,-1.96312905478001,-10.1886952830847));
#18466=CARTESIAN_POINT('Ctrl Pts',(11.1880912392172,-1.85649845736375,-10.029119502121));
#18467=CARTESIAN_POINT('Ctrl Pts',(10.9918630490257,-1.74829122417593,-9.86718424000794));
#18468=CARTESIAN_POINT('Ctrl Pts',(10.7966477335658,-1.64061939633818,-9.70516951171922));
#18469=CARTESIAN_POINT('Ctrl Pts',(10.603159058634,-1.53397337210466,-9.54359206502157));
#18470=CARTESIAN_POINT('Ctrl Pts',(10.4170476660417,-1.43139351779785,-9.38817519823602));
#18471=CARTESIAN_POINT('Ctrl Pts',(10.2325337582961,-1.32976299718735,-9.23316336539122));
#18472=CARTESIAN_POINT('Ctrl Pts',(10.0502525316942,-1.22955082275859,-9.07904823952839));
#18473=CARTESIAN_POINT('Ctrl Pts',(15.8,-4.38212029236875,-13.7206705386201));
#18474=CARTESIAN_POINT('Ctrl Pts',(15.8,-4.38395384756931,-13.7291554381927));
#18475=CARTESIAN_POINT('Ctrl Pts',(15.8,-4.38582790366735,-13.7376273491274));
#18476=CARTESIAN_POINT('Ctrl Pts',(15.8,-4.38774246062322,-13.7460862714518));
#18477=CARTESIAN_POINT('Ctrl Pts',(15.8,-4.38969752766812,-13.7545322021969));
#18478=CARTESIAN_POINT('Ctrl Pts',(15.8,-4.391693123397,-13.7629651342901));
#18479=CARTESIAN_POINT('Ctrl Pts',(10.0502525316942,-3.97495252086484,-8.25473589028142));
#18480=CARTESIAN_POINT('Ctrl Pts',(11.9668350211294,-5.45248982387649,-9.40148508750639));
#18481=CARTESIAN_POINT('Ctrl Pts',(13.8834175105647,-6.93002712688815,-10.5482342847314));
#18482=CARTESIAN_POINT('Ctrl Pts',(15.8,-8.40756442989979,-11.6949834819563));
#18483=CARTESIAN_POINT('Ctrl Pts',(10.0502525316942,-4.02899372351993,-8.40159082201815));
#18484=CARTESIAN_POINT('Ctrl Pts',(11.9668350211294,-5.52985728348807,-9.57068870058276));
#18485=CARTESIAN_POINT('Ctrl Pts',(13.8834175105647,-7.03115572742428,-10.7397728044506));
#18486=CARTESIAN_POINT('Ctrl Pts',(15.8,-8.53201928739242,-11.9088706830152));
#18487=CARTESIAN_POINT('Ctrl Pts',(10.0502525316942,-4.18428628311193,-8.6739375870516));
#18488=CARTESIAN_POINT('Ctrl Pts',(11.9668350211294,-5.73935104252813,-9.87945189609367));
#18489=CARTESIAN_POINT('Ctrl Pts',(13.8834175105647,-7.29468404041881,-11.0844841840221));
#18490=CARTESIAN_POINT('Ctrl Pts',(15.8,-8.84974879983501,-12.2899984930642));
#18491=CARTESIAN_POINT('Ctrl Pts',(10.0502525316941,-4.63834053369691,-9.04754461221301));
#18492=CARTESIAN_POINT('Ctrl Pts',(11.9668350211294,-6.31124182863326,-10.2794154126352));
#18493=CARTESIAN_POINT('Ctrl Pts',(13.8834175105647,-7.98413616433457,-11.5116939035746));
#18494=CARTESIAN_POINT('Ctrl Pts',(15.8,-9.65703745927091,-12.7435647039968));
#18495=CARTESIAN_POINT('Ctrl Pts',(10.0502525316942,-5.0347585282786,-9.26027499705532));
#18496=CARTESIAN_POINT('Ctrl Pts',(11.9668350211294,-6.79833782460276,-10.4948922896145));
#18497=CARTESIAN_POINT('Ctrl Pts',(13.8834175105647,-8.56244161305558,-11.7285731829415));
#18498=CARTESIAN_POINT('Ctrl Pts',(15.8,-10.3260209093797,-12.9631904755006));
#18499=CARTESIAN_POINT('Ctrl Pts',(10.0502525316942,-5.29266352931554,-9.36936257048691));
#18500=CARTESIAN_POINT('Ctrl Pts',(11.9668350211294,-7.11242577089738,-10.5998888833726));
#18501=CARTESIAN_POINT('Ctrl Pts',(13.8834175105647,-8.93218801247923,-11.8304151962582));
#18502=CARTESIAN_POINT('Ctrl Pts',(15.8,-10.7519502540611,-13.0609415091439));
#18503=CARTESIAN_POINT('',(10.0502525316942,-5.29266352931554,-9.36936257048691));
#18504=CARTESIAN_POINT('',(15.8,-8.40756442989979,-11.6949834819563));
#18505=CARTESIAN_POINT('Ctrl Pts',(15.8,-8.40756442989979,-11.6949834819563));
#18506=CARTESIAN_POINT('Ctrl Pts',(15.5486176029454,-8.21684279750569,-11.5498581470161));
#18507=CARTESIAN_POINT('Ctrl Pts',(15.295501252175,-8.02452322133501,-11.4033701387249));
#18508=CARTESIAN_POINT('Ctrl Pts',(15.0417457381091,-7.83135270226614,-11.2560089976682));
#18509=CARTESIAN_POINT('Ctrl Pts',(14.786900227078,-7.63735242672743,-11.1080148725475));
#18510=CARTESIAN_POINT('Ctrl Pts',(14.5314100499558,-7.44249371079127,-10.9591402752368));
#18511=CARTESIAN_POINT('Ctrl Pts',(14.2763841657387,-7.24756931575029,-10.8099197880108));
#18512=CARTESIAN_POINT('Ctrl Pts',(14.0169020050304,-7.04923884684419,-10.6580918487951));
#18513=CARTESIAN_POINT('Ctrl Pts',(13.7579005049334,-6.85084020761701,-10.5059060414985));
#18514=CARTESIAN_POINT('Ctrl Pts',(13.5005477794214,-6.6532485297061,-10.3539625665131));
#18515=CARTESIAN_POINT('Ctrl Pts',(13.3099967661962,-6.50694623445787,-10.2414594521442));
#18516=CARTESIAN_POINT('Ctrl Pts',(13.1203496652064,-6.36108719500292,-10.1290900041794));
#18517=CARTESIAN_POINT('Ctrl Pts',(12.9320806449423,-6.21604099337274,-10.0171093135792));
#18518=CARTESIAN_POINT('Ctrl Pts',(12.7398364624423,-6.06793224761101,-9.90276423285371));
#18519=CARTESIAN_POINT('Ctrl Pts',(12.5465418490578,-5.91877633502221,-9.78738841037967));
#18520=CARTESIAN_POINT('Ctrl Pts',(12.3528703671126,-5.76903486398375,-9.67121625884623));
#18521=CARTESIAN_POINT('Ctrl Pts',(12.158888214275,-5.61905319074317,-9.55485775408393));
#18522=CARTESIAN_POINT('Ctrl Pts',(11.9645279828276,-5.46848389786717,-9.43770055909668));
#18523=CARTESIAN_POINT('Ctrl Pts',(11.7704664817065,-5.3178321768124,-9.32001254164074));
#18524=CARTESIAN_POINT('Ctrl Pts',(11.5758141145072,-5.16672176100845,-9.20196619521737));
#18525=CARTESIAN_POINT('Ctrl Pts',(11.3814622995135,-5.01552828296833,-9.08338602074645));
#18526=CARTESIAN_POINT('Ctrl Pts',(11.1880940466175,-4.86480554216901,-8.96457159711292));
#18527=CARTESIAN_POINT('Ctrl Pts',(10.9918680747393,-4.71185532487872,-8.84400125838637));
#18528=CARTESIAN_POINT('Ctrl Pts',(10.7966549511886,-4.55938973719227,-8.72318989748018));
#18529=CARTESIAN_POINT('Ctrl Pts',(10.60316841745,-4.40803483977029,-8.60247741697936));
#18530=CARTESIAN_POINT('Ctrl Pts',(10.417053851698,-4.26244666645491,-8.4863641637459));
#18531=CARTESIAN_POINT('Ctrl Pts',(10.2325368136996,-4.11788655117373,-8.37034275782455));
#18532=CARTESIAN_POINT('Ctrl Pts',(10.0502525316942,-3.97495252086484,-8.25473589028142));
#18533=CARTESIAN_POINT('Ctrl Pts',(15.8,-8.40756442989979,-11.6949834819563));
#18534=CARTESIAN_POINT('Ctrl Pts',(15.8,-8.41193022268479,-11.7024865012679));
#18535=CARTESIAN_POINT('Ctrl Pts',(15.8,-8.41633052040236,-11.709964652185));
#18536=CARTESIAN_POINT('Ctrl Pts',(15.8,-8.4207653230234,-11.7174179347464));
#18537=CARTESIAN_POINT('Ctrl Pts',(15.8,-8.4252346384098,-11.7248463432757));
#18538=CARTESIAN_POINT('Ctrl Pts',(15.8,-8.42973848206085,-11.7322498653003));
#18539=CARTESIAN_POINT('Ctrl Pts',(10.0502525316942,-6.33125817110613,-6.62239247796685));
#18540=CARTESIAN_POINT('Ctrl Pts',(11.9668350211294,-8.09084464143287,-7.25643163809036));
#18541=CARTESIAN_POINT('Ctrl Pts',(13.8834175105647,-9.85043111175961,-7.89047079821388));
#18542=CARTESIAN_POINT('Ctrl Pts',(15.8,-11.6100175820864,-8.5245099583374));
#18543=CARTESIAN_POINT('Ctrl Pts',(10.0502525316942,-6.42803507865412,-6.74536016772823));
#18544=CARTESIAN_POINT('Ctrl Pts',(11.9668350211294,-8.21671225999593,-7.39344597705571));
#18545=CARTESIAN_POINT('Ctrl Pts',(13.8834175105647,-10.0057987839539,-8.04138429933134));
#18546=CARTESIAN_POINT('Ctrl Pts',(15.8,-11.7944759652957,-8.68947010865881));
#18547=CARTESIAN_POINT('Ctrl Pts',(10.0502525316942,-6.65988565896848,-6.95639005916883));
#18548=CARTESIAN_POINT('Ctrl Pts',(11.9668350211295,-8.51136454012837,-7.62236086025714));
#18549=CARTESIAN_POINT('Ctrl Pts',(13.8834175105647,-10.3629488876586,-8.28779124445879));
#18550=CARTESIAN_POINT('Ctrl Pts',(15.8,-12.2144277688185,-8.9537620455471));
#18551=CARTESIAN_POINT('Ctrl Pts',(10.0502525316941,-7.2071677757859,-7.17140112925234));
#18552=CARTESIAN_POINT('Ctrl Pts',(11.9668350211294,-9.17886046565844,-7.82602495118037));
#18553=CARTESIAN_POINT('Ctrl Pts',(13.8834175105647,-11.1506718004078,-8.48103967091341));
#18554=CARTESIAN_POINT('Ctrl Pts',(15.8,-13.1223644902804,-9.13566349284145));
#18555=CARTESIAN_POINT('Ctrl Pts',(10.0502525316942,-7.64992225296746,-7.2512189308223));
#18556=CARTESIAN_POINT('Ctrl Pts',(11.9668350211294,-9.70870355968973,-7.88043377854937));
#18557=CARTESIAN_POINT('Ctrl Pts',(13.8834175105647,-11.7676943247925,-8.50859598070372));
#18558=CARTESIAN_POINT('Ctrl Pts',(15.8,-13.8264756315148,-9.13781082843079));
#18559=CARTESIAN_POINT('Ctrl Pts',(10.0502525316942,-7.92891439885425,-7.2752703501265));
#18560=CARTESIAN_POINT('Ctrl Pts',(11.9668350211294,-10.0398646795257,-7.88323296009842));
#18561=CARTESIAN_POINT('Ctrl Pts',(13.8834175105647,-12.1508149601973,-8.49119557007034));
#18562=CARTESIAN_POINT('Ctrl Pts',(15.8,-14.2617652408688,-9.09915818004226));
#18563=CARTESIAN_POINT('',(10.0502525316942,-7.92891439885425,-7.2752703501265));
#18564=CARTESIAN_POINT('',(15.8,-11.6100175820864,-8.5245099583374));
#18565=CARTESIAN_POINT('Ctrl Pts',(15.8,-11.6100175820864,-8.5245099583374));
#18566=CARTESIAN_POINT('Ctrl Pts',(15.548617675428,-11.3837844012199,-8.44542381127114));
#18567=CARTESIAN_POINT('Ctrl Pts',(15.2955013981404,-11.1556103968132,-8.36553547761193));
#18568=CARTESIAN_POINT('Ctrl Pts',(15.0417459576101,-10.9263572847363,-8.2850797017454));
#18569=CARTESIAN_POINT('Ctrl Pts',(14.7869004713563,-10.6961193804757,-8.20427831565579));
#18570=CARTESIAN_POINT('Ctrl Pts',(14.5314103188166,-10.4647929695835,-8.1229048237753));
#18571=CARTESIAN_POINT('Ctrl Pts',(14.2763844586684,-10.2332972079334,-8.04122266692363));
#18572=CARTESIAN_POINT('Ctrl Pts',(14.0169022052127,-9.99775622450725,-7.95811317318572));
#18573=CARTESIAN_POINT('Ctrl Pts',(13.7579006122711,-9.76203981941543,-7.87468439208691));
#18574=CARTESIAN_POINT('Ctrl Pts',(13.5005477950648,-9.52716576583561,-7.79123671760531));
#18575=CARTESIAN_POINT('Ctrl Pts',(13.3099967765756,-9.35325863471441,-7.72944979203118));
#18576=CARTESIAN_POINT('Ctrl Pts',(13.1203496703585,-9.17981437027969,-7.66765301700902));
#18577=CARTESIAN_POINT('Ctrl Pts',(12.9320806449423,-9.00726329348628,-7.605974791296));
#18578=CARTESIAN_POINT('Ctrl Pts',(12.7398364200678,-8.83106889328649,-7.54299426293974));
#18579=CARTESIAN_POINT('Ctrl Pts',(12.5465417638457,-8.65356006118371,-7.47935703277431));
#18580=CARTESIAN_POINT('Ctrl Pts',(12.3528702390452,-8.47524825078831,-7.41514339569057));
#18581=CARTESIAN_POINT('Ctrl Pts',(12.1588880967135,-8.29665045733786,-7.35082677040841));
#18582=CARTESIAN_POINT('Ctrl Pts',(11.9645278759626,-8.11724699610012,-7.2859321298648));
#18583=CARTESIAN_POINT('Ctrl Pts',(11.7704663856167,-7.93760110830991,-7.22055811872365));
#18584=CARTESIAN_POINT('Ctrl Pts',(11.5758138300786,-7.75740806182779,-7.15498499387686));
#18585=CARTESIAN_POINT('Ctrl Pts',(11.3814618274404,-7.57697105649318,-7.08892983490284));
#18586=CARTESIAN_POINT('Ctrl Pts',(11.1880933895777,-7.3969093635474,-7.02250642528026));
#18587=CARTESIAN_POINT('Ctrl Pts',(10.9918668985605,-7.21418629579192,-6.95510125442768));
#18588=CARTESIAN_POINT('Ctrl Pts',(10.7966532620501,-7.03184966122232,-6.88731709712114));
#18589=CARTESIAN_POINT('Ctrl Pts',(10.6031662272204,-6.85059991984825,-6.81928375787452));
#18590=CARTESIAN_POINT('Ctrl Pts',(10.4170524040783,-6.67625706354084,-6.75384296552654));
#18591=CARTESIAN_POINT('Ctrl Pts',(10.2325360986482,-6.50292032538269,-6.6881718401968));
#18592=CARTESIAN_POINT('Ctrl Pts',(10.0502525316942,-6.33125817110613,-6.62239247796685));
#18593=CARTESIAN_POINT('Ctrl Pts',(15.8,-11.6100175820864,-8.5245099583374));
#18594=CARTESIAN_POINT('Ctrl Pts',(15.8,-11.6164882582397,-8.53029664958107));
#18595=CARTESIAN_POINT('Ctrl Pts',(15.8,-11.6229840657775,-8.53604902696561));
#18596=CARTESIAN_POINT('Ctrl Pts',(15.8,-11.6295050046841,-8.54176709053684));
#18597=CARTESIAN_POINT('Ctrl Pts',(15.8,-11.6360510806824,-8.54745083246671));
#18598=CARTESIAN_POINT('Ctrl Pts',(15.8,-11.642622304659,-8.55310023610356));
#18599=CARTESIAN_POINT('Ctrl Pts',(10.0502525316942,-8.06781615908999,-4.34180314898733));
#18600=CARTESIAN_POINT('Ctrl Pts',(11.9668350211294,-9.93721121325641,-4.40106810140592));
#18601=CARTESIAN_POINT('Ctrl Pts',(13.8834175105647,-11.8066062674228,-4.46033305382451));
#18602=CARTESIAN_POINT('Ctrl Pts',(15.8,-13.6760013215893,-4.51959800624309));
#18603=CARTESIAN_POINT('Ctrl Pts',(10.0502525316942,-8.19785557353568,-4.4288466625333));
#18604=CARTESIAN_POINT('Ctrl Pts',(11.9668350211294,-10.0992581912947,-4.49248124812732));
#18605=CARTESIAN_POINT('Ctrl Pts',(13.8834175105647,-12.0010045410108,-4.55584907137464));
#18606=CARTESIAN_POINT('Ctrl Pts',(15.8,-13.9024071587698,-4.61948365696866));
#18607=CARTESIAN_POINT('Ctrl Pts',(10.0502525316942,-8.48356457498288,-4.55790932427762));
#18608=CARTESIAN_POINT('Ctrl Pts',(11.9668350211294,-10.4502219249867,-4.61914675531024));
#18609=CARTESIAN_POINT('Ctrl Pts',(13.8834175105647,-12.416810143598,-4.67984453466858));
#18610=CARTESIAN_POINT('Ctrl Pts',(15.8,-14.3834674936017,-4.74108196570119));
#18611=CARTESIAN_POINT('Ctrl Pts',(10.0502525316941,-9.07050287838801,-4.59327853800037));
#18612=CARTESIAN_POINT('Ctrl Pts',(11.9668350211294,-11.1479839451212,-4.60657624071161));
#18613=CARTESIAN_POINT('Ctrl Pts',(13.8834175105647,-13.2256962639304,-4.62021662092401));
#18614=CARTESIAN_POINT('Ctrl Pts',(15.8,-15.3031773306636,-4.63351432363524));
#18615=CARTESIAN_POINT('Ctrl Pts',(10.0502525316942,-9.51625828739342,-4.5323630334273));
#18616=CARTESIAN_POINT('Ctrl Pts',(11.9668350211294,-11.668713745839,-4.49458350302914));
#18617=CARTESIAN_POINT('Ctrl Pts',(13.8834175105647,-13.8210431256713,-4.45573812100054));
#18618=CARTESIAN_POINT('Ctrl Pts',(15.8,-15.9734985841168,-4.41795859060238));
#18619=CARTESIAN_POINT('Ctrl Pts',(10.0502525316942,-9.78902788303806,-4.46902397810655));
#18620=CARTESIAN_POINT('Ctrl Pts',(11.9668350211294,-11.9845316814717,-4.39491126897609));
#18621=CARTESIAN_POINT('Ctrl Pts',(13.8834175105647,-14.1800354799052,-4.32079855984563));
#18622=CARTESIAN_POINT('Ctrl Pts',(15.8,-16.3755392783388,-4.24668585071518));
#18623=CARTESIAN_POINT('',(10.0502525316942,-9.78902788303806,-4.46902397810655));
#18624=CARTESIAN_POINT('',(15.8,-13.6760013215893,-4.51959800624309));
#18625=CARTESIAN_POINT('Ctrl Pts',(15.8,-13.6760013215893,-4.51959800624309));
#18626=CARTESIAN_POINT('Ctrl Pts',(15.5486181428671,-13.4364022627901,-4.51429251817173));
#18627=CARTESIAN_POINT('Ctrl Pts',(15.2955023394669,-13.1947094870246,-4.50882385781796));
#18628=CARTESIAN_POINT('Ctrl Pts',(15.0417473731653,-12.9518150706355,-4.50314899406863));
#18629=CARTESIAN_POINT('Ctrl Pts',(14.7869020465168,-12.7078769606235,-4.49744974598312));
#18630=CARTESIAN_POINT('Ctrl Pts',(14.5314120523244,-12.4627268269498,-4.49154276300943));
#18631=CARTESIAN_POINT('Ctrl Pts',(14.2763863472133,-12.2173202460879,-4.4853945547262));
#18632=CARTESIAN_POINT('Ctrl Pts',(14.0169034957054,-11.9676246346078,-4.47913889270852));
#18633=CARTESIAN_POINT('Ctrl Pts',(13.7579013040845,-11.7176635180538,-4.4726337773552));
#18634=CARTESIAN_POINT('Ctrl Pts',(13.5005478956174,-11.468497691795,-4.46585038850012));
#18635=CARTESIAN_POINT('Ctrl Pts',(13.3099968432927,-11.2840089349537,-4.46082779372524));
#18636=CARTESIAN_POINT('Ctrl Pts',(13.1203497034746,-11.0999573476229,-4.45565279642647));
#18637=CARTESIAN_POINT('Ctrl Pts',(12.9320806449423,-10.9167918673754,-4.45031453415308));
#18638=CARTESIAN_POINT('Ctrl Pts',(12.7398361468872,-10.7297587134111,-4.44486355054889));
#18639=CARTESIAN_POINT('Ctrl Pts',(12.5465412144993,-10.5412725252547,-4.43919418585342));
#18640=CARTESIAN_POINT('Ctrl Pts',(12.3528694134191,-10.3518445394597,-4.4332247563449));
#18641=CARTESIAN_POINT('Ctrl Pts',(12.1588873388167,-10.162113078982,-4.42724576346213));
#18642=CARTESIAN_POINT('Ctrl Pts',(11.9645271870236,-9.97143676938872,-4.42096600829024));
#18643=CARTESIAN_POINT('Ctrl Pts',(11.7704657661437,-9.78038176737598,-4.41430525673783));
#18644=CARTESIAN_POINT('Ctrl Pts',(11.5758119966794,-9.58874359350202,-4.40762417406171));
#18645=CARTESIAN_POINT('Ctrl Pts',(11.3814587845902,-9.39672444179026,-4.4005600302801));
#18646=CARTESIAN_POINT('Ctrl Pts',(11.1880891545372,-9.2049484464285,-4.39302967416941));
#18647=CARTESIAN_POINT('Ctrl Pts',(10.9918593168758,-9.01033581554701,-4.38538793354691));
#18648=CARTESIAN_POINT('Ctrl Pts',(10.7966423735553,-8.81597360566181,-4.37726632301399));
#18649=CARTESIAN_POINT('Ctrl Pts',(10.6031521084283,-8.62256814054964,-4.36857183761347));
#18650=CARTESIAN_POINT('Ctrl Pts',(10.4170430723425,-8.43654066954415,-4.36020902775276));
#18651=CARTESIAN_POINT('Ctrl Pts',(10.2325314892389,-8.25139886794607,-4.35131627654662));
#18652=CARTESIAN_POINT('Ctrl Pts',(10.0502525316942,-8.06781615908999,-4.34180314898733));
#18653=CARTESIAN_POINT('Ctrl Pts',(15.8,-13.6760013215893,-4.51959800624309));
#18654=CARTESIAN_POINT('Ctrl Pts',(15.8,-13.6839434862452,-4.52310192776169));
#18655=CARTESIAN_POINT('Ctrl Pts',(15.8,-13.6918989487026,-4.52656544883607));
#18656=CARTESIAN_POINT('Ctrl Pts',(15.8,-13.6998677089605,-4.52998856951466));
#18657=CARTESIAN_POINT('Ctrl Pts',(15.8,-13.7078497700428,-4.53337128058405));
#18658=CARTESIAN_POINT('Ctrl Pts',(15.8,-13.7158451371576,-4.53671356284346));
#18659=CARTESIAN_POINT('Ctrl Pts',(10.0502525316942,-9.01464008964162,-1.6362078766636));
#18660=CARTESIAN_POINT('Ctrl Pts',(11.9668350211294,-10.8108543149047,-1.11489735491132));
#18661=CARTESIAN_POINT('Ctrl Pts',(13.8834175105647,-12.6070685401678,-0.593586833159037));
#18662=CARTESIAN_POINT('Ctrl Pts',(15.8,-14.4032827654308,-0.0722763114067561));
#18663=CARTESIAN_POINT('Ctrl Pts',(10.0502525316942,-9.16521284706123,-1.67880678842043));
#18664=CARTESIAN_POINT('Ctrl Pts',(11.9668350211294,-10.9932183651601,-1.15176115367482));
#18665=CARTESIAN_POINT('Ctrl Pts',(13.8834175105647,-12.8214683576781,-0.624355593844837));
#18666=CARTESIAN_POINT('Ctrl Pts',(15.8,-14.6494738757771,-0.0973099590992228));
#18667=CARTESIAN_POINT('Ctrl Pts',(10.0502525316942,-9.47681709721301,-1.71327315824378));
#18668=CARTESIAN_POINT('Ctrl Pts',(11.9668350211294,-11.3661427921348,-1.16378287280497));
#18669=CARTESIAN_POINT('Ctrl Pts',(13.8834175105647,-13.2552357701884,-0.613808798404411));
#18670=CARTESIAN_POINT('Ctrl Pts',(15.8,-15.1445614651102,-0.0643185129655956));
#18671=CARTESIAN_POINT('Ctrl Pts',(10.0502525316941,-10.0459586957056,-1.56553830329486));
#18672=CARTESIAN_POINT('Ctrl Pts',(11.9668350211294,-12.025869817826,-0.936208214997369));
#18673=CARTESIAN_POINT('Ctrl Pts',(13.8834175105647,-14.0061068566225,-0.307141231238407));
#18674=CARTESIAN_POINT('Ctrl Pts',(15.8,-15.9860179787428,0.322188857059084));
#18675=CARTESIAN_POINT('Ctrl Pts',(10.0502525316942,-10.4510766569791,-1.36984786349029));
#18676=CARTESIAN_POINT('Ctrl Pts',(11.9668350211294,-12.4865089298363,-0.668772078627758));
#18677=CARTESIAN_POINT('Ctrl Pts',(13.8834175105647,-14.5214919285394,0.0332784309391876));
#18678=CARTESIAN_POINT('Ctrl Pts',(15.8,-16.5569242013966,0.734354215801724));
#18679=CARTESIAN_POINT('Ctrl Pts',(10.0502525316942,-10.6909231138624,-1.22531840158854));
#18680=CARTESIAN_POINT('Ctrl Pts',(11.9668350211294,-12.7560692212929,-0.47638504169901));
#18681=CARTESIAN_POINT('Ctrl Pts',(13.8834175105647,-14.8212153287235,0.272548318190525));
#18682=CARTESIAN_POINT('Ctrl Pts',(15.8,-16.886361436154,1.02148167808006));
#18683=CARTESIAN_POINT('',(10.0502525316942,-10.6909231138624,-1.22531840158854));
#18684=CARTESIAN_POINT('',(15.8,-14.4032827654308,-0.0722763114067561));
#18685=CARTESIAN_POINT('Ctrl Pts',(15.8,-14.4032827654308,-0.0722763114067562));
#18686=CARTESIAN_POINT('Ctrl Pts',(15.5486186601033,-14.1737715055211,-0.14127053144869));
#18687=CARTESIAN_POINT('Ctrl Pts',(15.2955033810747,-13.9422185866337,-0.210756563075385));
#18688=CARTESIAN_POINT('Ctrl Pts',(15.0417489395224,-13.7094591215774,-0.280417814422079));
#18689=CARTESIAN_POINT('Ctrl Pts',(14.7869037890753,-13.4756991900176,-0.350378489676399));
#18690=CARTESIAN_POINT('Ctrl Pts',(14.5314139696904,-13.2407223608428,-0.420516137034358));
#18691=CARTESIAN_POINT('Ctrl Pts',(14.2763884357272,-13.0054270908218,-0.490503613096571));
#18692=CARTESIAN_POINT('Ctrl Pts',(14.016904922593,-12.7660187369206,-0.561714506695313));
#18693=CARTESIAN_POINT('Ctrl Pts',(13.7579020686534,-12.5262807827901,-0.632770201644789));
#18694=CARTESIAN_POINT('Ctrl Pts',(13.5005480060758,-12.2872132071331,-0.703315478824681));
#18695=CARTESIAN_POINT('Ctrl Pts',(13.3099969165823,-12.1102018689489,-0.755548885558621));
#18696=CARTESIAN_POINT('Ctrl Pts',(13.1203497398531,-11.9335592090237,-0.807502254261612));
#18697=CARTESIAN_POINT('Ctrl Pts',(12.9320806449423,-11.7577088361878,-0.859026524117213));
#18698=CARTESIAN_POINT('Ctrl Pts',(12.7398358447897,-11.5781450060298,-0.911638839304067));
#18699=CARTESIAN_POINT('Ctrl Pts',(12.5465406070029,-11.3971317706544,-0.964492472593927));
#18700=CARTESIAN_POINT('Ctrl Pts',(12.3528685003979,-11.2151301058934,-1.0173517555325));
#18701=CARTESIAN_POINT('Ctrl Pts',(12.1588865006943,-11.032837221809,-1.0702956181623));
#18702=CARTESIAN_POINT('Ctrl Pts',(11.9645264251583,-10.8495527946037,-1.1232454100055));
#18703=CARTESIAN_POINT('Ctrl Pts',(11.7704650810977,-10.6657904772718,-1.1759498724029));
#18704=CARTESIAN_POINT('Ctrl Pts',(11.5758099697569,-10.4814659044743,-1.22881559404254));
#18705=CARTESIAN_POINT('Ctrl Pts',(11.3814554207386,-10.296660622926,-1.28143472519609));
#18706=CARTESIAN_POINT('Ctrl Pts',(11.188084472837,-10.1119425360181,-1.33353531202339));
#18707=CARTESIAN_POINT('Ctrl Pts',(10.9918509346348,-9.92448995248781,-1.38640717621227));
#18708=CARTESIAN_POINT('Ctrl Pts',(10.7966303348196,-9.73712725458383,-1.43874524883732));
#18709=CARTESIAN_POINT('Ctrl Pts',(10.6031364978028,-9.55049749194704,-1.49024279648039));
#18710=CARTESIAN_POINT('Ctrl Pts',(10.4170327545865,-9.37099566409686,-1.53977350262891));
#18711=CARTESIAN_POINT('Ctrl Pts',(10.2325263927835,-9.19217237538483,-1.58852655489952));
#18712=CARTESIAN_POINT('Ctrl Pts',(10.0502525316942,-9.01464008964162,-1.6362078766636));
#18713=CARTESIAN_POINT('Ctrl Pts',(15.8,-14.4032827654308,-0.0722763114067561));
#18714=CARTESIAN_POINT('Ctrl Pts',(15.8,-14.4119189841766,-0.0731544749487809));
#18715=CARTESIAN_POINT('Ctrl Pts',(15.8,-14.4205553654592,-0.0739901061384699));
#18716=CARTESIAN_POINT('Ctrl Pts',(15.8,-14.4291919092927,-0.0747832050221164));
#18717=CARTESIAN_POINT('Ctrl Pts',(15.8,-14.437828615706,-0.075533761902827));
#18718=CARTESIAN_POINT('Ctrl Pts',(15.8,-14.4464654837189,-0.0762417569101975));
#18719=CARTESIAN_POINT('Ctrl Pts',(10.0502525316942,-9.07904823952839,1.22955082275859));
#18720=CARTESIAN_POINT('Ctrl Pts',(11.9668350211294,-10.626255672559,2.28040731262864));
#18721=CARTESIAN_POINT('Ctrl Pts',(13.8834175105647,-12.1734631055895,3.33126380249869));
#18722=CARTESIAN_POINT('Ctrl Pts',(15.8,-13.7206705386201,4.38212029236874));
#18723=CARTESIAN_POINT('Ctrl Pts',(10.0502525316942,-9.23541522932356,1.23556639107773));
#18724=CARTESIAN_POINT('Ctrl Pts',(11.9668350211294,-10.8110857311875,2.3017013472912));
#18725=CARTESIAN_POINT('Ctrl Pts',(13.8834175105647,-12.3868775190731,3.36825415935174));
#18726=CARTESIAN_POINT('Ctrl Pts',(15.8,-13.962548020937,4.43438911556521));
#18727=CARTESIAN_POINT('Ctrl Pts',(10.0502525316942,-9.54242006948552,1.29909254545998));
#18728=CARTESIAN_POINT('Ctrl Pts',(11.9668350211295,-11.1694737466002,2.40552260970754));
#18729=CARTESIAN_POINT('Ctrl Pts',(13.8834175105647,-12.7961532691502,3.51235208206865));
#18730=CARTESIAN_POINT('Ctrl Pts',(15.8,-14.4232069462649,4.61878214631621));
#18731=CARTESIAN_POINT('Ctrl Pts',(10.0502525316941,-10.0380523375239,1.61547231497529));
#18732=CARTESIAN_POINT('Ctrl Pts',(11.9668350211294,-11.7265860195463,2.82582698043838));
#18733=CARTESIAN_POINT('Ctrl Pts',(13.8834175105647,-13.4155069687334,4.03604403376327));
#18734=CARTESIAN_POINT('Ctrl Pts',(15.8,-15.1040406507558,5.24639869922637));
#18735=CARTESIAN_POINT('Ctrl Pts',(10.0502525316942,-10.3628708264468,1.92675755961641));
#18736=CARTESIAN_POINT('Ctrl Pts',(11.9668350211294,-12.0820376211579,3.22250341643877));
#18737=CARTESIAN_POINT('Ctrl Pts',(13.8834175105647,-13.8004759242586,4.51903745819409));
#18738=CARTESIAN_POINT('Ctrl Pts',(15.8,-15.5196427189696,5.81478331501644));
#18739=CARTESIAN_POINT('Ctrl Pts',(10.0502525316942,-10.5463163022605,2.13832987737225));
#18740=CARTESIAN_POINT('Ctrl Pts',(11.9668350211294,-12.2789538289737,3.48877307262933));
#18741=CARTESIAN_POINT('Ctrl Pts',(13.8834175105647,-14.0115913556869,4.8392162678864));
#18742=CARTESIAN_POINT('Ctrl Pts',(15.8,-15.7442288824001,6.18965946314348));
#18743=CARTESIAN_POINT('',(10.0502525316942,-10.5463163022605,2.13832987737225));
#18744=CARTESIAN_POINT('',(15.8,-13.7206705386201,4.38212029236874));
#18745=CARTESIAN_POINT('Ctrl Pts',(15.8,-13.7206705386201,4.38212029236874));
#18746=CARTESIAN_POINT('Ctrl Pts',(15.5486179127188,-13.5237121602491,4.24557960414927));
#18747=CARTESIAN_POINT('Ctrl Pts',(15.2955018759953,-13.3249640154789,4.10794026962892));
#18748=CARTESIAN_POINT('Ctrl Pts',(15.0417466762024,-13.1251225182499,3.96976145165588));
#18749=CARTESIAN_POINT('Ctrl Pts',(14.7869012710154,-12.9244224444146,3.83098897769929));
#18750=CARTESIAN_POINT('Ctrl Pts',(14.5314111989041,-12.7226197192336,3.69167215691717));
#18751=CARTESIAN_POINT('Ctrl Pts',(14.2763854175035,-12.5204677360903,3.55239975641101));
#18752=CARTESIAN_POINT('Ctrl Pts',(14.0169028604367,-12.3147829883989,3.41069346140935));
#18753=CARTESIAN_POINT('Ctrl Pts',(13.7579009635655,-12.1087368195384,3.26903291905499));
#18754=CARTESIAN_POINT('Ctrl Pts',(13.5005478461955,-11.9031704882057,3.12806496166625));
#18755=CARTESIAN_POINT('Ctrl Pts',(13.3099968105011,-11.7509637547506,3.02368856803765));
#18756=CARTESIAN_POINT('Ctrl Pts',(13.1203496871979,-11.5990211190179,2.91969243162133));
#18757=CARTESIAN_POINT('Ctrl Pts',(12.9320806449423,-11.4476993942222,2.81634921885376));
#18758=CARTESIAN_POINT('Ctrl Pts',(12.7398362813706,-11.2931824947396,2.71082390290206));
#18759=CARTESIAN_POINT('Ctrl Pts',(12.5465414849356,-11.1373617066508,2.60462118886905));
#18760=CARTESIAN_POINT('Ctrl Pts',(12.3528698198645,-10.9806026156662,2.49810765644051));
#18761=CARTESIAN_POINT('Ctrl Pts',(12.1588877119198,-10.8235922502236,2.39142338986218));
#18762=CARTESIAN_POINT('Ctrl Pts',(11.9645275261796,-10.6656407015685,2.28442707498227));
#18763=CARTESIAN_POINT('Ctrl Pts',(11.7704660711025,-10.5071588397369,2.17751640137267));
#18764=CARTESIAN_POINT('Ctrl Pts',(11.5758128991794,-10.3481937475419,2.07027974418963));
#18765=CARTESIAN_POINT('Ctrl Pts',(11.3814602824285,-10.1886952830851,1.96312905478025));
#18766=CARTESIAN_POINT('Ctrl Pts',(11.1880912392174,-10.0291195021212,1.85649845736387));
#18767=CARTESIAN_POINT('Ctrl Pts',(10.9918630490259,-9.86718424000812,1.74829122417604));
#18768=CARTESIAN_POINT('Ctrl Pts',(10.796647733566,-9.7051695117194,1.6406193963383));
#18769=CARTESIAN_POINT('Ctrl Pts',(10.6031590586342,-9.54359206502174,1.53397337210477));
#18770=CARTESIAN_POINT('Ctrl Pts',(10.4170476660419,-9.38817519823614,1.43139351779793));
#18771=CARTESIAN_POINT('Ctrl Pts',(10.2325337582961,-9.23316336539128,1.32976299718739));
#18772=CARTESIAN_POINT('Ctrl Pts',(10.0502525316942,-9.07904823952839,1.22955082275859));
#18773=CARTESIAN_POINT('Ctrl Pts',(15.8,-13.7206705386201,4.38212029236874));
#18774=CARTESIAN_POINT('Ctrl Pts',(15.8,-13.7291554381927,4.38395384756931));
#18775=CARTESIAN_POINT('Ctrl Pts',(15.8,-13.7376273491274,4.38582790366735));
#18776=CARTESIAN_POINT('Ctrl Pts',(15.8,-13.7460862714518,4.38774246062322));
#18777=CARTESIAN_POINT('Ctrl Pts',(15.8,-13.7545322021969,4.38969752766811));
#18778=CARTESIAN_POINT('Ctrl Pts',(15.8,-13.7629651342901,4.39169312339699));
#18779=CARTESIAN_POINT('Ctrl Pts',(10.0502525316942,-8.25473589028142,3.97495252086484));
#18780=CARTESIAN_POINT('Ctrl Pts',(11.9668350211294,-9.40148508750639,5.45248982387649));
#18781=CARTESIAN_POINT('Ctrl Pts',(13.8834175105647,-10.5482342847314,6.93002712688815));
#18782=CARTESIAN_POINT('Ctrl Pts',(15.8,-11.6949834819563,8.40756442989979));
#18783=CARTESIAN_POINT('Ctrl Pts',(10.0502525316942,-8.40159082201815,4.02899372351993));
#18784=CARTESIAN_POINT('Ctrl Pts',(11.9668350211294,-9.57068870058276,5.52985728348807));
#18785=CARTESIAN_POINT('Ctrl Pts',(13.8834175105647,-10.7397728044506,7.03115572742428));
#18786=CARTESIAN_POINT('Ctrl Pts',(15.8,-11.9088706830152,8.53201928739242));
#18787=CARTESIAN_POINT('Ctrl Pts',(10.0502525316942,-8.6739375870516,4.18428628311193));
#18788=CARTESIAN_POINT('Ctrl Pts',(11.9668350211294,-9.87945189609367,5.73935104252813));
#18789=CARTESIAN_POINT('Ctrl Pts',(13.8834175105647,-11.0844841840221,7.29468404041881));
#18790=CARTESIAN_POINT('Ctrl Pts',(15.8,-12.2899984930642,8.84974879983501));
#18791=CARTESIAN_POINT('Ctrl Pts',(10.0502525316941,-9.04754461221301,4.63834053369691));
#18792=CARTESIAN_POINT('Ctrl Pts',(11.9668350211294,-10.2794154126352,6.31124182863326));
#18793=CARTESIAN_POINT('Ctrl Pts',(13.8834175105647,-11.5116939035746,7.98413616433457));
#18794=CARTESIAN_POINT('Ctrl Pts',(15.8,-12.7435647039968,9.65703745927091));
#18795=CARTESIAN_POINT('Ctrl Pts',(10.0502525316942,-9.26027499705532,5.0347585282786));
#18796=CARTESIAN_POINT('Ctrl Pts',(11.9668350211294,-10.4948922896145,6.79833782460276));
#18797=CARTESIAN_POINT('Ctrl Pts',(13.8834175105647,-11.7285731829415,8.56244161305558));
#18798=CARTESIAN_POINT('Ctrl Pts',(15.8,-12.9631904755006,10.3260209093797));
#18799=CARTESIAN_POINT('Ctrl Pts',(10.0502525316942,-9.36936257048691,5.29266352931554));
#18800=CARTESIAN_POINT('Ctrl Pts',(11.9668350211294,-10.5998888833726,7.11242577089738));
#18801=CARTESIAN_POINT('Ctrl Pts',(13.8834175105647,-11.8304151962582,8.93218801247923));
#18802=CARTESIAN_POINT('Ctrl Pts',(15.8,-13.0609415091439,10.7519502540611));
#18803=CARTESIAN_POINT('',(10.0502525316942,-9.36936257048691,5.29266352931554));
#18804=CARTESIAN_POINT('',(15.8,-11.6949834819563,8.40756442989979));
#18805=CARTESIAN_POINT('Ctrl Pts',(15.8,-11.6949834819563,8.40756442989979));
#18806=CARTESIAN_POINT('Ctrl Pts',(15.5486176029467,-11.5498581470169,8.2168427975067));
#18807=CARTESIAN_POINT('Ctrl Pts',(15.2955012521777,-11.4033701387264,8.02452322133705));
#18808=CARTESIAN_POINT('Ctrl Pts',(15.0417457381132,-11.2560089976705,7.83135270226922));
#18809=CARTESIAN_POINT('Ctrl Pts',(14.7869002270809,-11.1080148725492,7.63735242672965));
#18810=CARTESIAN_POINT('Ctrl Pts',(14.5314100499576,-10.9591402752378,7.44249371079261));
#18811=CARTESIAN_POINT('Ctrl Pts',(14.2763841657393,-10.8099197880111,7.24756931575076));
#18812=CARTESIAN_POINT('Ctrl Pts',(14.0169020050296,-10.6580918487946,7.04923884684354));
#18813=CARTESIAN_POINT('Ctrl Pts',(13.7579005049311,-10.5059060414972,6.85084020761523));
#18814=CARTESIAN_POINT('Ctrl Pts',(13.5005477794176,-10.3539625665109,6.65324852970321));
#18815=CARTESIAN_POINT('Ctrl Pts',(13.3099967661937,-10.2414594521427,6.50694623445595));
#18816=CARTESIAN_POINT('Ctrl Pts',(13.1203496652052,-10.1290900041786,6.36108719500196));
#18817=CARTESIAN_POINT('Ctrl Pts',(12.9320806449423,-10.0171093135792,6.21604099337274));
#18818=CARTESIAN_POINT('Ctrl Pts',(12.7398364624423,-9.9027642328537,6.06793224761101));
#18819=CARTESIAN_POINT('Ctrl Pts',(12.5465418490578,-9.78738841037966,5.9187763350222));
#18820=CARTESIAN_POINT('Ctrl Pts',(12.3528703671126,-9.67121625884623,5.76903486398374));
#18821=CARTESIAN_POINT('Ctrl Pts',(12.158888214275,-9.55485775408393,5.61905319074316));
#18822=CARTESIAN_POINT('Ctrl Pts',(11.9645279828276,-9.43770055909667,5.46848389786716));
#18823=CARTESIAN_POINT('Ctrl Pts',(11.7704664817064,-9.32001254164074,5.31783217681239));
#18824=CARTESIAN_POINT('Ctrl Pts',(11.5758141145071,-9.20196619521732,5.16672176100839));
#18825=CARTESIAN_POINT('Ctrl Pts',(11.3814622995134,-9.08338602074636,5.01552828296821));
#18826=CARTESIAN_POINT('Ctrl Pts',(11.1880940466173,-8.96457159711279,4.86480554216884));
#18827=CARTESIAN_POINT('Ctrl Pts',(10.9918680747392,-8.84400125838633,4.71185532487866));
#18828=CARTESIAN_POINT('Ctrl Pts',(10.7966549511887,-8.72318989748022,4.55938973719232));
#18829=CARTESIAN_POINT('Ctrl Pts',(10.6031684174502,-8.60247741697948,4.40803483977044));
#18830=CARTESIAN_POINT('Ctrl Pts',(10.4170538516981,-8.48636416374598,4.26244666645502));
#18831=CARTESIAN_POINT('Ctrl Pts',(10.2325368136997,-8.37034275782459,4.11788655117379));
#18832=CARTESIAN_POINT('Ctrl Pts',(10.0502525316942,-8.25473589028142,3.97495252086484));
#18833=CARTESIAN_POINT('Ctrl Pts',(15.8,-11.6949834819563,8.40756442989979));
#18834=CARTESIAN_POINT('Ctrl Pts',(15.8,-11.7024865012679,8.41193022268479));
#18835=CARTESIAN_POINT('Ctrl Pts',(15.8,-11.709964652185,8.41633052040236));
#18836=CARTESIAN_POINT('Ctrl Pts',(15.8,-11.7174179347464,8.4207653230234));
#18837=CARTESIAN_POINT('Ctrl Pts',(15.8,-11.7248463432757,8.4252346384098));
#18838=CARTESIAN_POINT('Ctrl Pts',(15.8,-11.7322498653003,8.42973848206085));
#18839=CARTESIAN_POINT('Ctrl Pts',(10.0502525316942,-6.62239247796685,6.33125817110613));
#18840=CARTESIAN_POINT('Ctrl Pts',(11.9668350211294,-7.25643163809036,8.09084464143287));
#18841=CARTESIAN_POINT('Ctrl Pts',(13.8834175105647,-7.89047079821388,9.85043111175961));
#18842=CARTESIAN_POINT('Ctrl Pts',(15.8,-8.5245099583374,11.6100175820864));
#18843=CARTESIAN_POINT('Ctrl Pts',(10.0502525316942,-6.74536016772823,6.42803507865412));
#18844=CARTESIAN_POINT('Ctrl Pts',(11.9668350211294,-7.39344597705571,8.21671225999593));
#18845=CARTESIAN_POINT('Ctrl Pts',(13.8834175105647,-8.04138429933134,10.0057987839539));
#18846=CARTESIAN_POINT('Ctrl Pts',(15.8,-8.68947010865881,11.7944759652957));
#18847=CARTESIAN_POINT('Ctrl Pts',(10.0502525316942,-6.95639005916883,6.65988565896847));
#18848=CARTESIAN_POINT('Ctrl Pts',(11.9668350211295,-7.62236086025714,8.51136454012837));
#18849=CARTESIAN_POINT('Ctrl Pts',(13.8834175105647,-8.28779124445879,10.3629488876586));
#18850=CARTESIAN_POINT('Ctrl Pts',(15.8,-8.9537620455471,12.2144277688185));
#18851=CARTESIAN_POINT('Ctrl Pts',(10.0502525316941,-7.17140112925234,7.2071677757859));
#18852=CARTESIAN_POINT('Ctrl Pts',(11.9668350211294,-7.82602495118037,9.17886046565844));
#18853=CARTESIAN_POINT('Ctrl Pts',(13.8834175105647,-8.48103967091341,11.1506718004078));
#18854=CARTESIAN_POINT('Ctrl Pts',(15.8,-9.13566349284145,13.1223644902804));
#18855=CARTESIAN_POINT('Ctrl Pts',(10.0502525316942,-7.2512189308223,7.64992225296746));
#18856=CARTESIAN_POINT('Ctrl Pts',(11.9668350211294,-7.88043377854937,9.70870355968973));
#18857=CARTESIAN_POINT('Ctrl Pts',(13.8834175105647,-8.50859598070372,11.7676943247925));
#18858=CARTESIAN_POINT('Ctrl Pts',(15.8,-9.13781082843079,13.8264756315148));
#18859=CARTESIAN_POINT('Ctrl Pts',(10.0502525316942,-7.2752703501265,7.92891439885425));
#18860=CARTESIAN_POINT('Ctrl Pts',(11.9668350211294,-7.88323296009842,10.0398646795257));
#18861=CARTESIAN_POINT('Ctrl Pts',(13.8834175105647,-8.49119557007034,12.1508149601973));
#18862=CARTESIAN_POINT('Ctrl Pts',(15.8,-9.09915818004226,14.2617652408688));
#18863=CARTESIAN_POINT('',(10.0502525316942,-7.2752703501265,7.92891439885425));
#18864=CARTESIAN_POINT('',(15.8,-8.5245099583374,11.6100175820864));
#18865=CARTESIAN_POINT('Ctrl Pts',(15.8,-8.5245099583374,11.6100175820864));
#18866=CARTESIAN_POINT('Ctrl Pts',(15.5486176754281,-8.44542381127117,11.38378440122));
#18867=CARTESIAN_POINT('Ctrl Pts',(15.2955013981405,-8.36553547761197,11.1556103968133));
#18868=CARTESIAN_POINT('Ctrl Pts',(15.0417459576102,-8.28507970174545,10.9263572847364));
#18869=CARTESIAN_POINT('Ctrl Pts',(14.7869004713576,-8.20427831565622,10.6961193804769));
#18870=CARTESIAN_POINT('Ctrl Pts',(14.5314103188191,-8.12290482377611,10.4647929695858));
#18871=CARTESIAN_POINT('Ctrl Pts',(14.2763844586721,-8.04122266692482,10.2332972079368));
#18872=CARTESIAN_POINT('Ctrl Pts',(14.0169022052159,-7.95811317318675,9.99775622451016));
#18873=CARTESIAN_POINT('Ctrl Pts',(13.7579006122738,-7.87468439208777,9.76203981941787));
#18874=CARTESIAN_POINT('Ctrl Pts',(13.5005477950669,-7.79123671760601,9.52716576583757));
#18875=CARTESIAN_POINT('Ctrl Pts',(13.309996776577,-7.72944979203165,9.35325863471571));
#18876=CARTESIAN_POINT('Ctrl Pts',(13.1203496703592,-7.66765301700925,9.17981437028034));
#18877=CARTESIAN_POINT('Ctrl Pts',(12.9320806449423,-7.60597479129601,9.00726329348628));
#18878=CARTESIAN_POINT('Ctrl Pts',(12.739836420068,-7.5429942629398,8.83106889328666));
#18879=CARTESIAN_POINT('Ctrl Pts',(12.5465417638461,-7.47935703277444,8.65356006118405));
#18880=CARTESIAN_POINT('Ctrl Pts',(12.3528702390458,-7.41514339569077,8.47524825078884));
#18881=CARTESIAN_POINT('Ctrl Pts',(12.158888096714,-7.35082677040859,8.29665045733833));
#18882=CARTESIAN_POINT('Ctrl Pts',(11.9645278759631,-7.28593212986495,8.11724699610054));
#18883=CARTESIAN_POINT('Ctrl Pts',(11.7704663856171,-7.22055811872379,7.93760110831027));
#18884=CARTESIAN_POINT('Ctrl Pts',(11.5758138300791,-7.15498499387704,7.75740806182827));
#18885=CARTESIAN_POINT('Ctrl Pts',(11.381461827441,-7.08892983490307,7.57697105649378));
#18886=CARTESIAN_POINT('Ctrl Pts',(11.1880933895784,-7.02250642528054,7.39690936354813));
#18887=CARTESIAN_POINT('Ctrl Pts',(10.9918668985614,-6.95510125442799,7.21418629579277));
#18888=CARTESIAN_POINT('Ctrl Pts',(10.7966532620511,-6.8873170971215,7.03184966122329));
#18889=CARTESIAN_POINT('Ctrl Pts',(10.6031662272216,-6.81928375787493,6.85059991984934));
#18890=CARTESIAN_POINT('Ctrl Pts',(10.417052404079,-6.75384296552681,6.67625706354156));
#18891=CARTESIAN_POINT('Ctrl Pts',(10.2325360986486,-6.68817184019694,6.50292032538305));
#18892=CARTESIAN_POINT('Ctrl Pts',(10.0502525316942,-6.62239247796685,6.33125817110613));
#18893=CARTESIAN_POINT('Ctrl Pts',(15.8,-8.5245099583374,11.6100175820864));
#18894=CARTESIAN_POINT('Ctrl Pts',(15.8,-8.53029664958107,11.6164882582397));
#18895=CARTESIAN_POINT('Ctrl Pts',(15.8,-8.53604902696561,11.6229840657775));
#18896=CARTESIAN_POINT('Ctrl Pts',(15.8,-8.54176709053684,11.6295050046841));
#18897=CARTESIAN_POINT('Ctrl Pts',(15.8,-8.54745083246671,11.6360510806824));
#18898=CARTESIAN_POINT('Ctrl Pts',(15.8,-8.55310023610356,11.642622304659));
#18899=CARTESIAN_POINT('Ctrl Pts',(10.0502525316942,-4.34180314898733,8.06781615908999));
#18900=CARTESIAN_POINT('Ctrl Pts',(11.9668350211294,-4.40106810140592,9.93721121325641));
#18901=CARTESIAN_POINT('Ctrl Pts',(13.8834175105647,-4.46033305382451,11.8066062674228));
#18902=CARTESIAN_POINT('Ctrl Pts',(15.8,-4.51959800624309,13.6760013215893));
#18903=CARTESIAN_POINT('Ctrl Pts',(10.0502525316942,-4.4288466625333,8.19785557353568));
#18904=CARTESIAN_POINT('Ctrl Pts',(11.9668350211294,-4.49248124812732,10.0992581912947));
#18905=CARTESIAN_POINT('Ctrl Pts',(13.8834175105647,-4.55584907137465,12.0010045410108));
#18906=CARTESIAN_POINT('Ctrl Pts',(15.8,-4.61948365696867,13.9024071587698));
#18907=CARTESIAN_POINT('Ctrl Pts',(10.0502525316942,-4.55790932427761,8.48356457498288));
#18908=CARTESIAN_POINT('Ctrl Pts',(11.9668350211294,-4.61914675531023,10.4502219249867));
#18909=CARTESIAN_POINT('Ctrl Pts',(13.8834175105647,-4.67984453466858,12.416810143598));
#18910=CARTESIAN_POINT('Ctrl Pts',(15.8,-4.7410819657012,14.3834674936017));
#18911=CARTESIAN_POINT('Ctrl Pts',(10.0502525316941,-4.59327853800039,9.07050287838801));
#18912=CARTESIAN_POINT('Ctrl Pts',(11.9668350211294,-4.60657624071163,11.1479839451212));
#18913=CARTESIAN_POINT('Ctrl Pts',(13.8834175105647,-4.62021662092399,13.2256962639304));
#18914=CARTESIAN_POINT('Ctrl Pts',(15.8,-4.63351432363522,15.3031773306636));
#18915=CARTESIAN_POINT('Ctrl Pts',(10.0502525316942,-4.53236303342729,9.51625828739342));
#18916=CARTESIAN_POINT('Ctrl Pts',(11.9668350211294,-4.49458350302913,11.668713745839));
#18917=CARTESIAN_POINT('Ctrl Pts',(13.8834175105647,-4.45573812100054,13.8210431256713));
#18918=CARTESIAN_POINT('Ctrl Pts',(15.8,-4.41795859060238,15.9734985841168));
#18919=CARTESIAN_POINT('Ctrl Pts',(10.0502525316942,-4.46902397810655,9.78902788303806));
#18920=CARTESIAN_POINT('Ctrl Pts',(11.9668350211294,-4.39491126897609,11.9845316814717));
#18921=CARTESIAN_POINT('Ctrl Pts',(13.8834175105647,-4.32079855984564,14.1800354799052));
#18922=CARTESIAN_POINT('Ctrl Pts',(15.8,-4.24668585071518,16.3755392783388));
#18923=CARTESIAN_POINT('',(10.0502525316942,-4.46902397810655,9.78902788303806));
#18924=CARTESIAN_POINT('',(15.8,-4.51959800624309,13.6760013215893));
#18925=CARTESIAN_POINT('Ctrl Pts',(15.8,-4.51959800624309,13.6760013215893));
#18926=CARTESIAN_POINT('Ctrl Pts',(15.5486181428668,-4.51429251817173,13.4364022627899));
#18927=CARTESIAN_POINT('Ctrl Pts',(15.2955023394664,-4.50882385781795,13.1947094870241));
#18928=CARTESIAN_POINT('Ctrl Pts',(15.0417473731645,-4.50314899406862,12.9518150706348));
#18929=CARTESIAN_POINT('Ctrl Pts',(14.7869020465161,-4.49744974598311,12.7078769606229));
#18930=CARTESIAN_POINT('Ctrl Pts',(14.531412052324,-4.49154276300942,12.4627268269494));
#18931=CARTESIAN_POINT('Ctrl Pts',(14.276386347213,-4.4853945547262,12.2173202460876));
#18932=CARTESIAN_POINT('Ctrl Pts',(14.0169034957048,-4.4791388927085,11.9676246346072));
#18933=CARTESIAN_POINT('Ctrl Pts',(13.7579013040838,-4.47263377735518,11.717663518053));
#18934=CARTESIAN_POINT('Ctrl Pts',(13.5005478956164,-4.46585038850009,11.468497691794));
#18935=CARTESIAN_POINT('Ctrl Pts',(13.309996843292,-4.46082779372523,11.2840089349531));
#18936=CARTESIAN_POINT('Ctrl Pts',(13.1203497034743,-4.45565279642646,11.0999573476226));
#18937=CARTESIAN_POINT('Ctrl Pts',(12.9320806449423,-4.45031453415308,10.9167918673754));
#18938=CARTESIAN_POINT('Ctrl Pts',(12.7398361468868,-4.44486355054888,10.7297587134107));
#18939=CARTESIAN_POINT('Ctrl Pts',(12.5465412144983,-4.43919418585339,10.5412725252538));
#18940=CARTESIAN_POINT('Ctrl Pts',(12.3528694134176,-4.43322475634486,10.3518445394583));
#18941=CARTESIAN_POINT('Ctrl Pts',(12.1588873388154,-4.42724576346209,10.1621130789808));
#18942=CARTESIAN_POINT('Ctrl Pts',(11.9645271870224,-4.4209660082902,9.97143676938756));
#18943=CARTESIAN_POINT('Ctrl Pts',(11.7704657661427,-4.41430525673779,9.78038176737493));
#18944=CARTESIAN_POINT('Ctrl Pts',(11.5758119966785,-4.40762417406168,9.58874359350119));
#18945=CARTESIAN_POINT('Ctrl Pts',(11.3814587845896,-4.40056003028007,9.39672444178965));
#18946=CARTESIAN_POINT('Ctrl Pts',(11.1880891545368,-4.39302967416939,9.2049484464281));
#18947=CARTESIAN_POINT('Ctrl Pts',(10.9918593168755,-4.3853879335469,9.01033581554672));
#18948=CARTESIAN_POINT('Ctrl Pts',(10.7966423735551,-4.37726632301398,8.81597360566162));
#18949=CARTESIAN_POINT('Ctrl Pts',(10.6031521084282,-4.36857183761346,8.62256814054954));
#18950=CARTESIAN_POINT('Ctrl Pts',(10.4170430723424,-4.36020902775276,8.43654066954408));
#18951=CARTESIAN_POINT('Ctrl Pts',(10.2325314892389,-4.35131627654661,8.25139886794604));
#18952=CARTESIAN_POINT('Ctrl Pts',(10.0502525316942,-4.34180314898733,8.06781615908999));
#18953=CARTESIAN_POINT('Ctrl Pts',(15.8,-4.51959800624309,13.6760013215893));
#18954=CARTESIAN_POINT('Ctrl Pts',(15.8,-4.52310192776169,13.6839434862452));
#18955=CARTESIAN_POINT('Ctrl Pts',(15.8,-4.52656544883607,13.6918989487026));
#18956=CARTESIAN_POINT('Ctrl Pts',(15.8,-4.52998856951466,13.6998677089605));
#18957=CARTESIAN_POINT('Ctrl Pts',(15.8,-4.53337128058405,13.7078497700428));
#18958=CARTESIAN_POINT('Ctrl Pts',(15.8,-4.53671356284346,13.7158451371576));
#18959=CARTESIAN_POINT('Ctrl Pts',(10.0502525316942,-1.6362078766636,9.01464008964162));
#18960=CARTESIAN_POINT('Ctrl Pts',(11.9668350211294,-1.11489735491132,10.8108543149047));
#18961=CARTESIAN_POINT('Ctrl Pts',(13.8834175105647,-0.593586833159038,
12.6070685401678));
#18962=CARTESIAN_POINT('Ctrl Pts',(15.8,-0.072276311406757,14.4032827654308));
#18963=CARTESIAN_POINT('Ctrl Pts',(10.0502525316942,-1.67880678842043,9.16521284706123));
#18964=CARTESIAN_POINT('Ctrl Pts',(11.9668350211294,-1.15176115367482,10.9932183651601));
#18965=CARTESIAN_POINT('Ctrl Pts',(13.8834175105647,-0.624355593844837,
12.8214683576781));
#18966=CARTESIAN_POINT('Ctrl Pts',(15.8,-0.0973099590992238,14.6494738757771));
#18967=CARTESIAN_POINT('Ctrl Pts',(10.0502525316942,-1.71327315824378,9.47681709721301));
#18968=CARTESIAN_POINT('Ctrl Pts',(11.9668350211294,-1.16378287280496,11.3661427921348));
#18969=CARTESIAN_POINT('Ctrl Pts',(13.8834175105647,-0.613808798404414,
13.2552357701884));
#18970=CARTESIAN_POINT('Ctrl Pts',(15.8,-0.064318512965597,15.1445614651102));
#18971=CARTESIAN_POINT('Ctrl Pts',(10.0502525316941,-1.56553830329486,10.0459586957056));
#18972=CARTESIAN_POINT('Ctrl Pts',(11.9668350211294,-0.936208214997367,
12.025869817826));
#18973=CARTESIAN_POINT('Ctrl Pts',(13.8834175105647,-0.307141231238408,
14.0061068566225));
#18974=CARTESIAN_POINT('Ctrl Pts',(15.8,0.322188857059081,15.9860179787428));
#18975=CARTESIAN_POINT('Ctrl Pts',(10.0502525316942,-1.36984786349029,10.4510766569791));
#18976=CARTESIAN_POINT('Ctrl Pts',(11.9668350211294,-0.668772078627758,
12.4865089298363));
#18977=CARTESIAN_POINT('Ctrl Pts',(13.8834175105647,0.0332784309391854,
14.5214919285394));
#18978=CARTESIAN_POINT('Ctrl Pts',(15.8,0.734354215801722,16.5569242013966));
#18979=CARTESIAN_POINT('Ctrl Pts',(10.0502525316942,-1.22531840158854,10.6909231138624));
#18980=CARTESIAN_POINT('Ctrl Pts',(11.9668350211294,-0.47638504169901,12.7560692212929));
#18981=CARTESIAN_POINT('Ctrl Pts',(13.8834175105647,0.272548318190524,14.8212153287235));
#18982=CARTESIAN_POINT('Ctrl Pts',(15.8,1.02148167808006,16.886361436154));
#18983=CARTESIAN_POINT('',(10.0502525316942,-1.22531840158854,10.6909231138624));
#18984=CARTESIAN_POINT('',(15.8,-0.072276311406757,14.4032827654308));
#18985=CARTESIAN_POINT('Ctrl Pts',(15.8,-0.0722763114067571,14.4032827654308));
#18986=CARTESIAN_POINT('Ctrl Pts',(15.5486186601032,-0.141270531448724,
14.173771505521));
#18987=CARTESIAN_POINT('Ctrl Pts',(15.2955033810745,-0.210756563075445,
13.9422185866335));
#18988=CARTESIAN_POINT('Ctrl Pts',(15.0417489395221,-0.28041781442216,13.7094591215771));
#18989=CARTESIAN_POINT('Ctrl Pts',(14.7869037890755,-0.350378489676339,
13.4756991900178));
#18990=CARTESIAN_POINT('Ctrl Pts',(14.5314139696912,-0.420516137034151,
13.2407223608434));
#18991=CARTESIAN_POINT('Ctrl Pts',(14.2763884357285,-0.490503613096215,
13.005427090823));
#18992=CARTESIAN_POINT('Ctrl Pts',(14.0169049225932,-0.561714506695251,
12.7660187369208));
#18993=CARTESIAN_POINT('Ctrl Pts',(13.7579020686526,-0.632770201645017,
12.5262807827893));
#18994=CARTESIAN_POINT('Ctrl Pts',(13.5005480060739,-0.703315478825194,
12.2872132071314));
#18995=CARTESIAN_POINT('Ctrl Pts',(13.3099969165811,-0.755548885558961,
12.1102018689477));
#18996=CARTESIAN_POINT('Ctrl Pts',(13.1203497398525,-0.807502254261781,
11.9335592090231));
#18997=CARTESIAN_POINT('Ctrl Pts',(12.9320806449423,-0.859026524117214,
11.7577088361878));
#18998=CARTESIAN_POINT('Ctrl Pts',(12.7398358447895,-0.911638839304132,
11.5781450060296));
#18999=CARTESIAN_POINT('Ctrl Pts',(12.5465406070024,-0.964492472594062,
11.397131770654));
#19000=CARTESIAN_POINT('Ctrl Pts',(12.3528685003971,-1.0173517555327,11.2151301058927));
#19001=CARTESIAN_POINT('Ctrl Pts',(12.1588865006936,-1.07029561816249,11.0328372218084));
#19002=CARTESIAN_POINT('Ctrl Pts',(11.9645264251577,-1.12324541000567,10.8495527946032));
#19003=CARTESIAN_POINT('Ctrl Pts',(11.7704650810972,-1.17594987240305,10.6657904772713));
#19004=CARTESIAN_POINT('Ctrl Pts',(11.5758099697562,-1.22881559404272,10.4814659044737));
#19005=CARTESIAN_POINT('Ctrl Pts',(11.3814554207379,-1.28143472519631,10.2966606229252));
#19006=CARTESIAN_POINT('Ctrl Pts',(11.1880844728361,-1.33353531202364,10.1119425360172));
#19007=CARTESIAN_POINT('Ctrl Pts',(10.991850934634,-1.38640717621249,9.92448995248705));
#19008=CARTESIAN_POINT('Ctrl Pts',(10.796630334819,-1.4387452488375,9.73712725458319));
#19009=CARTESIAN_POINT('Ctrl Pts',(10.6031364978022,-1.49024279648053,9.55049749194653));
#19010=CARTESIAN_POINT('Ctrl Pts',(10.4170327545862,-1.539773502629,9.37099566409652));
#19011=CARTESIAN_POINT('Ctrl Pts',(10.2325263927833,-1.58852655489957,9.19217237538466));
#19012=CARTESIAN_POINT('Ctrl Pts',(10.0502525316942,-1.6362078766636,9.01464008964162));
#19013=CARTESIAN_POINT('Ctrl Pts',(15.8,-0.072276311406757,14.4032827654308));
#19014=CARTESIAN_POINT('Ctrl Pts',(15.8,-0.0731544749487818,14.4119189841766));
#19015=CARTESIAN_POINT('Ctrl Pts',(15.8,-0.0739901061384708,14.4205553654592));
#19016=CARTESIAN_POINT('Ctrl Pts',(15.8,-0.0747832050221173,14.4291919092927));
#19017=CARTESIAN_POINT('Ctrl Pts',(15.8,-0.0755337619028279,14.437828615706));
#19018=CARTESIAN_POINT('Ctrl Pts',(15.8,-0.0762417569101984,14.4464654837189));
#19019=CARTESIAN_POINT('Ctrl Pts',(10.0502525316942,1.22955082275859,9.07904823952839));
#19020=CARTESIAN_POINT('Ctrl Pts',(11.9668350211294,2.28040731262864,10.626255672559));
#19021=CARTESIAN_POINT('Ctrl Pts',(13.8834175105647,3.33126380249869,12.1734631055895));
#19022=CARTESIAN_POINT('Ctrl Pts',(15.8,4.38212029236874,13.7206705386201));
#19023=CARTESIAN_POINT('Ctrl Pts',(10.0502525316942,1.23556639107773,9.23541522932356));
#19024=CARTESIAN_POINT('Ctrl Pts',(11.9668350211294,2.3017013472912,10.8110857311875));
#19025=CARTESIAN_POINT('Ctrl Pts',(13.8834175105647,3.36825415935174,12.386877519073));
#19026=CARTESIAN_POINT('Ctrl Pts',(15.8,4.43438911556521,13.962548020937));
#19027=CARTESIAN_POINT('Ctrl Pts',(10.0502525316942,1.29909254545998,9.54242006948551));
#19028=CARTESIAN_POINT('Ctrl Pts',(11.9668350211295,2.40552260970754,11.1694737466002));
#19029=CARTESIAN_POINT('Ctrl Pts',(13.8834175105647,3.51235208206865,12.7961532691502));
#19030=CARTESIAN_POINT('Ctrl Pts',(15.8,4.61878214631621,14.4232069462649));
#19031=CARTESIAN_POINT('Ctrl Pts',(10.0502525316941,1.61547231497529,10.0380523375239));
#19032=CARTESIAN_POINT('Ctrl Pts',(11.9668350211294,2.82582698043838,11.7265860195464));
#19033=CARTESIAN_POINT('Ctrl Pts',(13.8834175105647,4.03604403376328,13.4155069687334));
#19034=CARTESIAN_POINT('Ctrl Pts',(15.8,5.24639869922637,15.1040406507558));
#19035=CARTESIAN_POINT('Ctrl Pts',(10.0502525316942,1.92675755961642,10.3628708264469));
#19036=CARTESIAN_POINT('Ctrl Pts',(11.9668350211294,3.22250341643878,12.0820376211579));
#19037=CARTESIAN_POINT('Ctrl Pts',(13.8834175105647,4.51903745819409,13.8004759242586));
#19038=CARTESIAN_POINT('Ctrl Pts',(15.8,5.81478331501644,15.5196427189696));
#19039=CARTESIAN_POINT('Ctrl Pts',(10.0502525316942,2.13832987737225,10.5463163022605));
#19040=CARTESIAN_POINT('Ctrl Pts',(11.9668350211294,3.48877307262933,12.2789538289737));
#19041=CARTESIAN_POINT('Ctrl Pts',(13.8834175105647,4.8392162678864,14.0115913556869));
#19042=CARTESIAN_POINT('Ctrl Pts',(15.8,6.18965946314348,15.7442288824001));
#19043=CARTESIAN_POINT('',(10.0502525316942,2.13832987737225,10.5463163022605));
#19044=CARTESIAN_POINT('',(15.8,4.38212029236874,13.7206705386201));
#19045=CARTESIAN_POINT('Ctrl Pts',(15.8,4.38212029236874,13.7206705386201));
#19046=CARTESIAN_POINT('Ctrl Pts',(15.54861791272,4.24557960414993,13.5237121602501));
#19047=CARTESIAN_POINT('Ctrl Pts',(15.2955018759977,4.10794026963023,13.3249640154808));
#19048=CARTESIAN_POINT('Ctrl Pts',(15.041746676206,3.96976145165784,13.1251225182527));
#19049=CARTESIAN_POINT('Ctrl Pts',(14.7869012710187,3.83098897770111,12.9244224444172));
#19050=CARTESIAN_POINT('Ctrl Pts',(14.5314111989072,3.69167215691884,12.722619719236));
#19051=CARTESIAN_POINT('Ctrl Pts',(14.2763854175063,3.55239975641252,12.5204677360925));
#19052=CARTESIAN_POINT('Ctrl Pts',(14.0169028604397,3.41069346141102,12.3147829884014));
#19053=CARTESIAN_POINT('Ctrl Pts',(13.7579009635688,3.26903291905679,12.1087368195411));
#19054=CARTESIAN_POINT('Ctrl Pts',(13.500547846199,3.12806496166819,11.9031704882085));
#19055=CARTESIAN_POINT('Ctrl Pts',(13.3099968105034,3.02368856803894,11.7509637547525));
#19056=CARTESIAN_POINT('Ctrl Pts',(13.1203496871991,2.91969243162197,11.5990211190189));
#19057=CARTESIAN_POINT('Ctrl Pts',(12.9320806449423,2.81634921885376,11.4476993942222));
#19058=CARTESIAN_POINT('Ctrl Pts',(12.7398362813703,2.71082390290191,11.2931824947394));
#19059=CARTESIAN_POINT('Ctrl Pts',(12.5465414849351,2.60462118886877,11.1373617066504));
#19060=CARTESIAN_POINT('Ctrl Pts',(12.3528698198637,2.49810765644009,10.9806026156656));
#19061=CARTESIAN_POINT('Ctrl Pts',(12.1588877119191,2.39142338986178,10.8235922502231));
#19062=CARTESIAN_POINT('Ctrl Pts',(11.9645275261789,2.28442707498191,10.665640701568));
#19063=CARTESIAN_POINT('Ctrl Pts',(11.7704660711019,2.17751640137234,10.5071588397364));
#19064=CARTESIAN_POINT('Ctrl Pts',(11.5758128991788,2.07027974418934,10.3481937475415));
#19065=CARTESIAN_POINT('Ctrl Pts',(11.381460282428,1.96312905477998,10.1886952830847));
#19066=CARTESIAN_POINT('Ctrl Pts',(11.188091239217,1.85649845736363,10.0291195021208));
#19067=CARTESIAN_POINT('Ctrl Pts',(10.9918630490254,1.74829122417577,9.86718424000771));
#19068=CARTESIAN_POINT('Ctrl Pts',(10.7966477335654,1.64061939633799,9.70516951171893));
#19069=CARTESIAN_POINT('Ctrl Pts',(10.6031590586335,1.53397337210443,9.54359206502122));
#19070=CARTESIAN_POINT('Ctrl Pts',(10.4170476660415,1.4313935177977,9.38817519823579));
#19071=CARTESIAN_POINT('Ctrl Pts',(10.2325337582959,1.32976299718728,9.23316336539111));
#19072=CARTESIAN_POINT('Ctrl Pts',(10.0502525316942,1.22955082275859,9.07904823952839));
#19073=CARTESIAN_POINT('Ctrl Pts',(15.8,4.38212029236874,13.7206705386201));
#19074=CARTESIAN_POINT('Ctrl Pts',(15.8,4.38395384756931,13.7291554381927));
#19075=CARTESIAN_POINT('Ctrl Pts',(15.8,4.38582790366735,13.7376273491274));
#19076=CARTESIAN_POINT('Ctrl Pts',(15.8,4.38774246062322,13.7460862714518));
#19077=CARTESIAN_POINT('Ctrl Pts',(15.8,4.38969752766811,13.7545322021969));
#19078=CARTESIAN_POINT('Ctrl Pts',(15.8,4.39169312339699,13.7629651342901));
#19079=CARTESIAN_POINT('Ctrl Pts',(10.0502525316942,3.97495252086484,8.25473589028142));
#19080=CARTESIAN_POINT('Ctrl Pts',(11.9668350211294,5.45248982387649,9.40148508750639));
#19081=CARTESIAN_POINT('Ctrl Pts',(13.8834175105647,6.93002712688814,10.5482342847314));
#19082=CARTESIAN_POINT('Ctrl Pts',(15.8,8.40756442989979,11.6949834819563));
#19083=CARTESIAN_POINT('Ctrl Pts',(10.0502525316942,4.02899372351994,8.40159082201815));
#19084=CARTESIAN_POINT('Ctrl Pts',(11.9668350211294,5.52985728348808,9.57068870058276));
#19085=CARTESIAN_POINT('Ctrl Pts',(13.8834175105647,7.03115572742427,10.7397728044506));
#19086=CARTESIAN_POINT('Ctrl Pts',(15.8,8.53201928739241,11.9088706830152));
#19087=CARTESIAN_POINT('Ctrl Pts',(10.0502525316942,4.18428628311196,8.6739375870516));
#19088=CARTESIAN_POINT('Ctrl Pts',(11.9668350211294,5.73935104252815,9.87945189609366));
#19089=CARTESIAN_POINT('Ctrl Pts',(13.8834175105647,7.2946840404188,11.0844841840221));
#19090=CARTESIAN_POINT('Ctrl Pts',(15.8,8.84974879983499,12.2899984930642));
#19091=CARTESIAN_POINT('Ctrl Pts',(10.0502525316941,4.63834053369693,9.04754461221299));
#19092=CARTESIAN_POINT('Ctrl Pts',(11.9668350211294,6.31124182863328,10.2794154126352));
#19093=CARTESIAN_POINT('Ctrl Pts',(13.8834175105647,7.98413616433457,11.5116939035747));
#19094=CARTESIAN_POINT('Ctrl Pts',(15.8,9.65703745927091,12.7435647039969));
#19095=CARTESIAN_POINT('Ctrl Pts',(10.0502525316942,5.0347585282786,9.26027499705535));
#19096=CARTESIAN_POINT('Ctrl Pts',(11.9668350211294,6.79833782460276,10.4948922896145));
#19097=CARTESIAN_POINT('Ctrl Pts',(13.8834175105647,8.56244161305558,11.7285731829415));
#19098=CARTESIAN_POINT('Ctrl Pts',(15.8,10.3260209093797,12.9631904755006));
#19099=CARTESIAN_POINT('Ctrl Pts',(10.0502525316942,5.29266352931554,9.36936257048691));
#19100=CARTESIAN_POINT('Ctrl Pts',(11.9668350211294,7.11242577089738,10.5998888833726));
#19101=CARTESIAN_POINT('Ctrl Pts',(13.8834175105647,8.93218801247923,11.8304151962582));
#19102=CARTESIAN_POINT('Ctrl Pts',(15.8,10.7519502540611,13.0609415091439));
#19103=CARTESIAN_POINT('',(10.0502525316942,5.29266352931554,9.36936257048691));
#19104=CARTESIAN_POINT('',(15.8,8.40756442989979,11.6949834819563));
#19105=CARTESIAN_POINT('Ctrl Pts',(15.8,8.40756442989979,11.6949834819563));
#19106=CARTESIAN_POINT('Ctrl Pts',(15.5486176029462,8.21684279750629,11.5498581470166));
#19107=CARTESIAN_POINT('Ctrl Pts',(15.2955012521766,8.02452322133619,11.4033701387258));
#19108=CARTESIAN_POINT('Ctrl Pts',(15.0417457381114,7.83135270226788,11.2560089976695));
#19109=CARTESIAN_POINT('Ctrl Pts',(14.7869002270796,7.63735242672867,11.1080148725485));
#19110=CARTESIAN_POINT('Ctrl Pts',(14.5314100499567,7.44249371079197,10.9591402752373));
#19111=CARTESIAN_POINT('Ctrl Pts',(14.2763841657389,7.24756931575045,10.8099197880109));
#19112=CARTESIAN_POINT('Ctrl Pts',(14.0169020050304,7.04923884684417,10.6580918487951));
#19113=CARTESIAN_POINT('Ctrl Pts',(13.7579005049332,6.8508402076168,10.5059060414984));
#19114=CARTESIAN_POINT('Ctrl Pts',(13.5005477794209,6.6532485297057,10.3539625665128));
#19115=CARTESIAN_POINT('Ctrl Pts',(13.3099967661958,6.50694623445761,10.241459452144));
#19116=CARTESIAN_POINT('Ctrl Pts',(13.1203496652063,6.36108719500278,10.1290900041793));
#19117=CARTESIAN_POINT('Ctrl Pts',(12.9320806449423,6.21604099337274,10.0171093135792));
#19118=CARTESIAN_POINT('Ctrl Pts',(12.7398364624423,6.06793224761099,9.90276423285369));
#19119=CARTESIAN_POINT('Ctrl Pts',(12.5465418490578,5.91877633502217,9.78738841037964));
#19120=CARTESIAN_POINT('Ctrl Pts',(12.3528703671126,5.76903486398371,9.6712162588462));
#19121=CARTESIAN_POINT('Ctrl Pts',(12.158888214275,5.61905319074313,9.5548577540839));
#19122=CARTESIAN_POINT('Ctrl Pts',(11.9645279828276,5.46848389786713,9.43770055909665));
#19123=CARTESIAN_POINT('Ctrl Pts',(11.7704664817064,5.31783217681237,9.32001254164072));
#19124=CARTESIAN_POINT('Ctrl Pts',(11.5758141145067,5.16672176100811,9.20196619521711));
#19125=CARTESIAN_POINT('Ctrl Pts',(11.3814622995127,5.01552828296769,9.08338602074594));
#19126=CARTESIAN_POINT('Ctrl Pts',(11.1880940466163,4.86480554216807,8.96457159711218));
#19127=CARTESIAN_POINT('Ctrl Pts',(10.9918680747382,4.71185532487785,8.84400125838568));
#19128=CARTESIAN_POINT('Ctrl Pts',(10.7966549511876,4.55938973719146,8.72318989747954));
#19129=CARTESIAN_POINT('Ctrl Pts',(10.603168417449,4.40803483976955,8.60247741697877));
#19130=CARTESIAN_POINT('Ctrl Pts',(10.4170538516974,4.26244666645443,8.48636416374551));
#19131=CARTESIAN_POINT('Ctrl Pts',(10.2325368136993,4.1178865511735,8.37034275782436));
#19132=CARTESIAN_POINT('Ctrl Pts',(10.0502525316942,3.97495252086484,8.25473589028142));
#19133=CARTESIAN_POINT('Ctrl Pts',(15.8,8.40756442989979,11.6949834819563));
#19134=CARTESIAN_POINT('Ctrl Pts',(15.8,8.41193022268479,11.7024865012679));
#19135=CARTESIAN_POINT('Ctrl Pts',(15.8,8.41633052040235,11.709964652185));
#19136=CARTESIAN_POINT('Ctrl Pts',(15.8,8.4207653230234,11.7174179347465));
#19137=CARTESIAN_POINT('Ctrl Pts',(15.8,8.4252346384098,11.7248463432758));
#19138=CARTESIAN_POINT('Ctrl Pts',(15.8,8.42973848206085,11.7322498653004));
#19139=CARTESIAN_POINT('Ctrl Pts',(10.0502525316942,6.33125817110613,6.62239247796685));
#19140=CARTESIAN_POINT('Ctrl Pts',(11.9668350211294,8.09084464143287,7.25643163809036));
#19141=CARTESIAN_POINT('Ctrl Pts',(13.8834175105647,9.85043111175961,7.89047079821388));
#19142=CARTESIAN_POINT('Ctrl Pts',(15.8,11.6100175820863,8.5245099583374));
#19143=CARTESIAN_POINT('Ctrl Pts',(10.0502525316942,6.42803507865412,6.74536016772823));
#19144=CARTESIAN_POINT('Ctrl Pts',(11.9668350211294,8.21671225999592,7.39344597705571));
#19145=CARTESIAN_POINT('Ctrl Pts',(13.8834175105647,10.0057987839539,8.04138429933134));
#19146=CARTESIAN_POINT('Ctrl Pts',(15.8,11.7944759652957,8.68947010865881));
#19147=CARTESIAN_POINT('Ctrl Pts',(10.0502525316942,6.65988565896844,6.95639005916882));
#19148=CARTESIAN_POINT('Ctrl Pts',(11.9668350211295,8.51136454012834,7.62236086025713));
#19149=CARTESIAN_POINT('Ctrl Pts',(13.8834175105647,10.3629488876587,8.28779124445879));
#19150=CARTESIAN_POINT('Ctrl Pts',(15.8,12.2144277688186,8.9537620455471));
#19151=CARTESIAN_POINT('Ctrl Pts',(10.0502525316941,7.20716777578592,7.17140112925233));
#19152=CARTESIAN_POINT('Ctrl Pts',(11.9668350211294,9.17886046565845,7.82602495118037));
#19153=CARTESIAN_POINT('Ctrl Pts',(13.8834175105647,11.1506718004079,8.48103967091341));
#19154=CARTESIAN_POINT('Ctrl Pts',(15.8,13.1223644902804,9.13566349284145));
#19155=CARTESIAN_POINT('Ctrl Pts',(10.0502525316942,7.64992225296743,7.2512189308223));
#19156=CARTESIAN_POINT('Ctrl Pts',(11.9668350211294,9.70870355968971,7.88043377854937));
#19157=CARTESIAN_POINT('Ctrl Pts',(13.8834175105647,11.7676943247925,8.50859598070372));
#19158=CARTESIAN_POINT('Ctrl Pts',(15.8,13.8264756315148,9.13781082843079));
#19159=CARTESIAN_POINT('Ctrl Pts',(10.0502525316942,7.92891439885425,7.2752703501265));
#19160=CARTESIAN_POINT('Ctrl Pts',(11.9668350211294,10.0398646795257,7.88323296009842));
#19161=CARTESIAN_POINT('Ctrl Pts',(13.8834175105647,12.1508149601973,8.49119557007034));
#19162=CARTESIAN_POINT('Ctrl Pts',(15.8,14.2617652408688,9.09915818004226));
#19163=CARTESIAN_POINT('',(10.0502525316942,7.92891439885425,7.2752703501265));
#19164=CARTESIAN_POINT('',(15.8,11.6100175820863,8.5245099583374));
#19165=CARTESIAN_POINT('Ctrl Pts',(15.8,11.6100175820863,8.5245099583374));
#19166=CARTESIAN_POINT('Ctrl Pts',(15.548617675428,11.3837844012199,8.44542381127114));
#19167=CARTESIAN_POINT('Ctrl Pts',(15.2955013981403,11.1556103968132,8.36553547761191));
#19168=CARTESIAN_POINT('Ctrl Pts',(15.0417459576099,10.9263572847362,8.28507970174537));
#19169=CARTESIAN_POINT('Ctrl Pts',(14.786900471357,10.6961193804763,8.20427831565601));
#19170=CARTESIAN_POINT('Ctrl Pts',(14.5314103188181,10.4647929695849,8.12290482377579));
#19171=CARTESIAN_POINT('Ctrl Pts',(14.2763844586707,10.2332972079355,8.04122266692438));
#19172=CARTESIAN_POINT('Ctrl Pts',(14.0169022052158,9.99775622451002,7.9581131731867));
#19173=CARTESIAN_POINT('Ctrl Pts',(13.7579006122748,9.76203981941886,7.87468439208812));
#19174=CARTESIAN_POINT('Ctrl Pts',(13.5005477950692,9.52716576583967,7.79123671760675));
#19175=CARTESIAN_POINT('Ctrl Pts',(13.3099967765785,9.35325863471711,7.72944979203215));
#19176=CARTESIAN_POINT('Ctrl Pts',(13.1203496703599,9.17981437028103,7.6676530170095));
#19177=CARTESIAN_POINT('Ctrl Pts',(12.9320806449423,9.00726329348628,7.605974791296));
#19178=CARTESIAN_POINT('Ctrl Pts',(12.7398364200685,8.83106889328712,7.54299426293996));
#19179=CARTESIAN_POINT('Ctrl Pts',(12.5465417638471,8.65356006118498,7.47935703277477));
#19180=CARTESIAN_POINT('Ctrl Pts',(12.3528702390473,8.47524825079023,7.41514339569127));
#19181=CARTESIAN_POINT('Ctrl Pts',(12.1588880967154,8.29665045733962,7.35082677040905));
#19182=CARTESIAN_POINT('Ctrl Pts',(11.9645278759643,8.11724699610171,7.28593212986538));
#19183=CARTESIAN_POINT('Ctrl Pts',(11.7704663856183,7.93760110831134,7.22055811872417));
#19184=CARTESIAN_POINT('Ctrl Pts',(11.5758138300802,7.75740806182931,7.15498499387742));
#19185=CARTESIAN_POINT('Ctrl Pts',(11.3814618274421,7.57697105649479,7.08892983490344));
#19186=CARTESIAN_POINT('Ctrl Pts',(11.1880933895795,7.39690936354911,7.0225064252809));
#19187=CARTESIAN_POINT('Ctrl Pts',(10.9918668985623,7.21418629579357,6.95510125442829));
#19188=CARTESIAN_POINT('Ctrl Pts',(10.7966532620518,7.03184966122392,6.88731709712173));
#19189=CARTESIAN_POINT('Ctrl Pts',(10.6031662272221,6.85059991984979,6.8192837578751));
#19190=CARTESIAN_POINT('Ctrl Pts',(10.4170524040794,6.67625706354185,6.75384296552693));
#19191=CARTESIAN_POINT('Ctrl Pts',(10.2325360986488,6.50292032538319,6.68817184019699));
#19192=CARTESIAN_POINT('Ctrl Pts',(10.0502525316942,6.33125817110613,6.62239247796685));
#19193=CARTESIAN_POINT('Ctrl Pts',(15.8,11.6100175820863,8.5245099583374));
#19194=CARTESIAN_POINT('Ctrl Pts',(15.8,11.6164882582397,8.53029664958107));
#19195=CARTESIAN_POINT('Ctrl Pts',(15.8,11.6229840657775,8.53604902696561));
#19196=CARTESIAN_POINT('Ctrl Pts',(15.8,11.6295050046841,8.54176709053684));
#19197=CARTESIAN_POINT('Ctrl Pts',(15.8,11.6360510806824,8.54745083246671));
#19198=CARTESIAN_POINT('Ctrl Pts',(15.8,11.642622304659,8.55310023610356));
#19199=CARTESIAN_POINT('Ctrl Pts',(10.0502525316942,8.06781615908999,4.34180314898733));
#19200=CARTESIAN_POINT('Ctrl Pts',(11.9668350211294,9.93721121325641,4.40106810140592));
#19201=CARTESIAN_POINT('Ctrl Pts',(13.8834175105647,11.8066062674228,4.46033305382451));
#19202=CARTESIAN_POINT('Ctrl Pts',(15.8,13.6760013215893,4.51959800624309));
#19203=CARTESIAN_POINT('Ctrl Pts',(10.0502525316942,8.19785557353568,4.4288466625333));
#19204=CARTESIAN_POINT('Ctrl Pts',(11.9668350211294,10.0992581912947,4.49248124812732));
#19205=CARTESIAN_POINT('Ctrl Pts',(13.8834175105647,12.0010045410108,4.55584907137465));
#19206=CARTESIAN_POINT('Ctrl Pts',(15.8,13.9024071587698,4.61948365696866));
#19207=CARTESIAN_POINT('Ctrl Pts',(10.0502525316942,8.48356457498289,4.55790932427761));
#19208=CARTESIAN_POINT('Ctrl Pts',(11.9668350211294,10.4502219249867,4.61914675531023));
#19209=CARTESIAN_POINT('Ctrl Pts',(13.8834175105647,12.416810143598,4.67984453466857));
#19210=CARTESIAN_POINT('Ctrl Pts',(15.8,14.3834674936017,4.74108196570119));
#19211=CARTESIAN_POINT('Ctrl Pts',(10.0502525316941,9.07050287838801,4.59327853800039));
#19212=CARTESIAN_POINT('Ctrl Pts',(11.9668350211294,11.1479839451212,4.60657624071163));
#19213=CARTESIAN_POINT('Ctrl Pts',(13.8834175105647,13.2256962639304,4.62021662092402));
#19214=CARTESIAN_POINT('Ctrl Pts',(15.8,15.3031773306636,4.63351432363526));
#19215=CARTESIAN_POINT('Ctrl Pts',(10.0502525316942,9.51625828739344,4.53236303342729));
#19216=CARTESIAN_POINT('Ctrl Pts',(11.9668350211294,11.668713745839,4.49458350302913));
#19217=CARTESIAN_POINT('Ctrl Pts',(13.8834175105647,13.8210431256712,4.45573812100054));
#19218=CARTESIAN_POINT('Ctrl Pts',(15.8,15.9734985841168,4.41795859060239));
#19219=CARTESIAN_POINT('Ctrl Pts',(10.0502525316942,9.78902788303806,4.46902397810655));
#19220=CARTESIAN_POINT('Ctrl Pts',(11.9668350211294,11.9845316814717,4.39491126897609));
#19221=CARTESIAN_POINT('Ctrl Pts',(13.8834175105647,14.1800354799052,4.32079855984564));
#19222=CARTESIAN_POINT('Ctrl Pts',(15.8,16.3755392783388,4.24668585071518));
#19223=CARTESIAN_POINT('',(10.0502525316942,9.78902788303806,4.46902397810655));
#19224=CARTESIAN_POINT('',(15.8,13.6760013215893,4.51959800624309));
#19225=CARTESIAN_POINT('Ctrl Pts',(15.8,13.6760013215893,4.51959800624309));
#19226=CARTESIAN_POINT('Ctrl Pts',(15.5486181428676,13.4364022627906,4.51429251817174));
#19227=CARTESIAN_POINT('Ctrl Pts',(15.2955023394679,13.1947094870255,4.50882385781798));
#19228=CARTESIAN_POINT('Ctrl Pts',(15.0417473731668,12.9518150706369,4.50314899406867));
#19229=CARTESIAN_POINT('Ctrl Pts',(14.7869020465191,12.7078769606257,4.49744974598318));
#19230=CARTESIAN_POINT('Ctrl Pts',(14.5314120523275,12.4627268269528,4.49154276300951));
#19231=CARTESIAN_POINT('Ctrl Pts',(14.2763863472172,12.2173202460916,4.4853945547263));
#19232=CARTESIAN_POINT('Ctrl Pts',(14.01690349571,11.9676246346122,4.47913889270863));
#19233=CARTESIAN_POINT('Ctrl Pts',(13.7579013040899,11.7176635180589,4.47263377735534));
#19234=CARTESIAN_POINT('Ctrl Pts',(13.5005478956234,11.4684976918008,4.46585038850028));
#19235=CARTESIAN_POINT('Ctrl Pts',(13.3099968432967,11.2840089349576,4.46082779372536));
#19236=CARTESIAN_POINT('Ctrl Pts',(13.1203497034766,11.0999573476248,4.45565279642653));
#19237=CARTESIAN_POINT('Ctrl Pts',(12.9320806449423,10.9167918673754,4.45031453415308));
#19238=CARTESIAN_POINT('Ctrl Pts',(12.7398361468874,10.7297587134113,4.4448635505489));
#19239=CARTESIAN_POINT('Ctrl Pts',(12.5465412144996,10.5412725252551,4.43919418585343));
#19240=CARTESIAN_POINT('Ctrl Pts',(12.3528694134196,10.3518445394602,4.43322475634492));
#19241=CARTESIAN_POINT('Ctrl Pts',(12.1588873388172,10.1621130789825,4.42724576346214));
#19242=CARTESIAN_POINT('Ctrl Pts',(11.964527187024,9.97143676938913,4.42096600829026));
#19243=CARTESIAN_POINT('Ctrl Pts',(11.7704657661441,9.78038176737634,4.41430525673784));
#19244=CARTESIAN_POINT('Ctrl Pts',(11.5758119966797,9.58874359350238,4.40762417406172));
#19245=CARTESIAN_POINT('Ctrl Pts',(11.3814587845906,9.39672444179062,4.40056003028011));
#19246=CARTESIAN_POINT('Ctrl Pts',(11.1880891545376,9.20494844642885,4.39302967416942));
#19247=CARTESIAN_POINT('Ctrl Pts',(10.9918593168763,9.01033581554755,4.38538793354694));
#19248=CARTESIAN_POINT('Ctrl Pts',(10.796642373556,8.81597360566253,4.37726632301402));
#19249=CARTESIAN_POINT('Ctrl Pts',(10.6031521084292,8.62256814055053,4.36857183761351));
#19250=CARTESIAN_POINT('Ctrl Pts',(10.4170430723431,8.43654066954474,4.36020902775279));
#19251=CARTESIAN_POINT('Ctrl Pts',(10.2325314892392,8.25139886794637,4.35131627654663));
#19252=CARTESIAN_POINT('Ctrl Pts',(10.0502525316942,8.06781615908999,4.34180314898733));
#19253=CARTESIAN_POINT('Ctrl Pts',(15.8,13.6760013215893,4.51959800624309));
#19254=CARTESIAN_POINT('Ctrl Pts',(15.8,13.6839434862452,4.52310192776169));
#19255=CARTESIAN_POINT('Ctrl Pts',(15.8,13.6918989487026,4.52656544883607));
#19256=CARTESIAN_POINT('Ctrl Pts',(15.8,13.6998677089605,4.52998856951466));
#19257=CARTESIAN_POINT('Ctrl Pts',(15.8,13.7078497700428,4.53337128058406));
#19258=CARTESIAN_POINT('Ctrl Pts',(15.8,13.7158451371576,4.53671356284346));
#19259=CARTESIAN_POINT('Ctrl Pts',(10.0502525316942,9.01464008964162,1.6362078766636));
#19260=CARTESIAN_POINT('Ctrl Pts',(11.9668350211294,10.8108543149047,1.11489735491132));
#19261=CARTESIAN_POINT('Ctrl Pts',(13.8834175105647,12.6070685401678,0.593586833159039));
#19262=CARTESIAN_POINT('Ctrl Pts',(15.8,14.4032827654308,0.0722763114067579));
#19263=CARTESIAN_POINT('Ctrl Pts',(10.0502525316942,9.16521284706123,1.67880678842043));
#19264=CARTESIAN_POINT('Ctrl Pts',(11.9668350211294,10.9932183651601,1.15176115367482));
#19265=CARTESIAN_POINT('Ctrl Pts',(13.8834175105647,12.8214683576781,0.624355593844838));
#19266=CARTESIAN_POINT('Ctrl Pts',(15.8,14.6494738757771,0.0973099590992247));
#19267=CARTESIAN_POINT('Ctrl Pts',(10.0502525316942,9.47681709721301,1.71327315824379));
#19268=CARTESIAN_POINT('Ctrl Pts',(11.9668350211294,11.3661427921348,1.16378287280497));
#19269=CARTESIAN_POINT('Ctrl Pts',(13.8834175105647,13.2552357701884,0.613808798404414));
#19270=CARTESIAN_POINT('Ctrl Pts',(15.8,15.1445614651102,0.0643185129655977));
#19271=CARTESIAN_POINT('Ctrl Pts',(10.0502525316941,10.0459586957056,1.56553830329485));
#19272=CARTESIAN_POINT('Ctrl Pts',(11.9668350211294,12.025869817826,0.936208214997364));
#19273=CARTESIAN_POINT('Ctrl Pts',(13.8834175105647,14.0061068566225,0.307141231238409));
#19274=CARTESIAN_POINT('Ctrl Pts',(15.8,15.9860179787428,-0.32218885705908));
#19275=CARTESIAN_POINT('Ctrl Pts',(10.0502525316942,10.4510766569791,1.3698478634903));
#19276=CARTESIAN_POINT('Ctrl Pts',(11.9668350211294,12.4865089298363,0.668772078627759));
#19277=CARTESIAN_POINT('Ctrl Pts',(13.8834175105647,14.5214919285394,-0.0332784309391845));
#19278=CARTESIAN_POINT('Ctrl Pts',(15.8,16.5569242013966,-0.734354215801722));
#19279=CARTESIAN_POINT('Ctrl Pts',(10.0502525316942,10.6909231138624,1.22531840158854));
#19280=CARTESIAN_POINT('Ctrl Pts',(11.9668350211294,12.7560692212929,0.476385041699011));
#19281=CARTESIAN_POINT('Ctrl Pts',(13.8834175105647,14.8212153287235,-0.272548318190523));
#19282=CARTESIAN_POINT('Ctrl Pts',(15.8,16.886361436154,-1.02148167808006));
#19283=CARTESIAN_POINT('',(10.0502525316942,10.6909231138624,1.22531840158854));
#19284=CARTESIAN_POINT('',(15.8,14.4032827654308,0.0722763114067579));
#19285=CARTESIAN_POINT('Ctrl Pts',(15.8,14.4032827654308,0.0722763114067579));
#19286=CARTESIAN_POINT('Ctrl Pts',(15.5486186601037,14.1737715055214,0.141270531448591));
#19287=CARTESIAN_POINT('Ctrl Pts',(15.2955033810755,13.9422185866344,0.210756563075182));
#19288=CARTESIAN_POINT('Ctrl Pts',(15.0417489395235,13.7094591215784,0.280417814421773));
#19289=CARTESIAN_POINT('Ctrl Pts',(14.7869037890761,13.4756991900184,0.350378489676167));
#19290=CARTESIAN_POINT('Ctrl Pts',(14.531413969691,13.2407223608433,0.4205161370342));
#19291=CARTESIAN_POINT('Ctrl Pts',(14.2763884357275,13.0054270908221,0.490503613096486));
#19292=CARTESIAN_POINT('Ctrl Pts',(14.0169049225932,12.7660187369208,0.56171450669525));
#19293=CARTESIAN_POINT('Ctrl Pts',(13.7579020686536,12.5262807827902,0.632770201644749));
#19294=CARTESIAN_POINT('Ctrl Pts',(13.5005480060759,12.2872132071332,0.703315478824662));
#19295=CARTESIAN_POINT('Ctrl Pts',(13.3099969165824,12.1102018689489,0.755548885558609));
#19296=CARTESIAN_POINT('Ctrl Pts',(13.1203497398532,11.9335592090237,0.807502254261607));
#19297=CARTESIAN_POINT('Ctrl Pts',(12.9320806449423,11.7577088361878,0.859026524117214));
#19298=CARTESIAN_POINT('Ctrl Pts',(12.7398358447892,11.5781450060293,0.911638839304226));
#19299=CARTESIAN_POINT('Ctrl Pts',(12.5465406070018,11.3971317706534,0.964492472594246));
#19300=CARTESIAN_POINT('Ctrl Pts',(12.3528685003961,11.2151301058918,1.01735175553297));
#19301=CARTESIAN_POINT('Ctrl Pts',(12.1588865006927,11.0328372218075,1.07029561816274));
#19302=CARTESIAN_POINT('Ctrl Pts',(11.9645264251569,10.8495527946024,1.1232454100059));
#19303=CARTESIAN_POINT('Ctrl Pts',(11.7704650810964,10.6657904772706,1.17594987240326));
#19304=CARTESIAN_POINT('Ctrl Pts',(11.5758099697556,10.4814659044731,1.2288155940429));
#19305=CARTESIAN_POINT('Ctrl Pts',(11.3814554207373,10.2966606229247,1.28143472519645));
#19306=CARTESIAN_POINT('Ctrl Pts',(11.1880844728357,10.1119425360169,1.33353531202374));
#19307=CARTESIAN_POINT('Ctrl Pts',(10.9918509346335,9.92448995248661,1.38640717621261));
#19308=CARTESIAN_POINT('Ctrl Pts',(10.7966303348184,9.73712725458267,1.43874524883765));
#19309=CARTESIAN_POINT('Ctrl Pts',(10.6031364978016,9.55049749194593,1.49024279648069));
#19310=CARTESIAN_POINT('Ctrl Pts',(10.4170327545858,9.37099566409612,1.53977350262911));
#19311=CARTESIAN_POINT('Ctrl Pts',(10.2325263927831,9.19217237538446,1.58852655489962));
#19312=CARTESIAN_POINT('Ctrl Pts',(10.0502525316942,9.01464008964162,1.6362078766636));
#19313=CARTESIAN_POINT('Ctrl Pts',(15.8,14.4032827654308,0.0722763114067579));
#19314=CARTESIAN_POINT('Ctrl Pts',(15.8,14.4119189841766,0.0731544749487826));
#19315=CARTESIAN_POINT('Ctrl Pts',(15.8,14.4205553654592,0.0739901061384717));
#19316=CARTESIAN_POINT('Ctrl Pts',(15.8,14.4291919092927,0.0747832050221182));
#19317=CARTESIAN_POINT('Ctrl Pts',(15.8,14.437828615706,0.0755337619028287));
#19318=CARTESIAN_POINT('Ctrl Pts',(15.8,14.4464654837189,0.0762417569101993));
#19319=CARTESIAN_POINT('Ctrl Pts',(10.0502525316942,10.5463163022605,-2.13832987737225));
#19320=CARTESIAN_POINT('Ctrl Pts',(11.9668350211294,12.2789538289737,-3.48877307262933));
#19321=CARTESIAN_POINT('Ctrl Pts',(13.8834175105647,14.0115913556869,-4.8392162678864));
#19322=CARTESIAN_POINT('Ctrl Pts',(15.8,15.7442288824001,-6.18965946314348));
#19323=CARTESIAN_POINT('Ctrl Pts',(10.0502525316942,10.4407180108925,-2.39160131057558));
#19324=CARTESIAN_POINT('Ctrl Pts',(11.9668350211294,12.1359573145141,-3.77416649083142));
#19325=CARTESIAN_POINT('Ctrl Pts',(13.8834175105647,13.8309364798931,-5.15732892266062));
#19326=CARTESIAN_POINT('Ctrl Pts',(15.8,15.5261757835147,-6.53989410291646));
#19327=CARTESIAN_POINT('Ctrl Pts',(10.0502525316942,10.2391038402362,-2.76042111194549));
#19328=CARTESIAN_POINT('Ctrl Pts',(11.9668350211294,11.8698223691572,-4.18872035504581));
#19329=CARTESIAN_POINT('Ctrl Pts',(13.8834175105647,13.5008577836237,-5.61629814839675));
#19330=CARTESIAN_POINT('Ctrl Pts',(15.8,15.1315763125447,-7.04459739149707));
#19331=CARTESIAN_POINT('Ctrl Pts',(10.0502525316942,10.0106660065973,-2.88380634898391));
#19332=CARTESIAN_POINT('Ctrl Pts',(11.9668350211294,11.5875472242667,-4.31947109051328));
#19333=CARTESIAN_POINT('Ctrl Pts',(13.8834175105647,13.1642822866715,-5.75550424110767));
#19334=CARTESIAN_POINT('Ctrl Pts',(15.8,14.7411635043409,-7.19116898263704));
#19335=CARTESIAN_POINT('Ctrl Pts',(10.0502525316942,9.83366631411429,-2.90441220847246));
#19336=CARTESIAN_POINT('Ctrl Pts',(11.9668350211294,11.3745625747195,-4.33027001363173));
#19337=CARTESIAN_POINT('Ctrl Pts',(13.8834175105647,12.9152995332973,-5.75638324902558));
#19338=CARTESIAN_POINT('Ctrl Pts',(15.8,14.4561957939025,-7.18224105418485));
#19339=CARTESIAN_POINT('Ctrl Pts',(10.0502525316941,9.65650945139357,-2.93414649567711));
#19340=CARTESIAN_POINT('Ctrl Pts',(11.9668350211294,11.1613433397504,-4.34899924292337));
#19341=CARTESIAN_POINT('Ctrl Pts',(13.8834175105647,12.6660861533134,-5.76416819477548));
#19342=CARTESIAN_POINT('Ctrl Pts',(15.8,14.1709200416702,-7.17902094202175));
#19343=CARTESIAN_POINT('Ctrl Pts',(10.0502525316942,9.38996734645582,-3.00074150798573));
#19344=CARTESIAN_POINT('Ctrl Pts',(11.9668350211294,10.8390518176275,-4.40343923355922));
#19345=CARTESIAN_POINT('Ctrl Pts',(13.8834175105647,12.2880463890101,-5.80619247524443));
#19346=CARTESIAN_POINT('Ctrl Pts',(15.8,13.7371308601818,-7.20889020081793));
#19347=CARTESIAN_POINT('Ctrl Pts',(10.0502525316942,9.13374448664767,-2.99092345166593));
#19348=CARTESIAN_POINT('Ctrl Pts',(11.9668350211294,10.5342467491227,-4.37002011593522));
#19349=CARTESIAN_POINT('Ctrl Pts',(13.8834175105647,11.9347028120052,-5.74920012742634));
#19350=CARTESIAN_POINT('Ctrl Pts',(15.8,13.3352050744803,-7.12829679169563));
#19351=CARTESIAN_POINT('Ctrl Pts',(10.0502525316942,8.89063737063807,-2.94970615383952));
#19352=CARTESIAN_POINT('Ctrl Pts',(11.9668350211294,10.2485256494886,-4.29832412978306));
#19353=CARTESIAN_POINT('Ctrl Pts',(13.8834175105647,11.6063785007713,-5.64703889510257));
#19354=CARTESIAN_POINT('Ctrl Pts',(15.8,12.9642667796218,-6.99565687104612));
#19355=CARTESIAN_POINT('Ctrl Pts',(10.0502525316942,8.77435756124985,-2.90932499072146));
#19356=CARTESIAN_POINT('Ctrl Pts',(11.9668350211294,10.113663592731,-4.23975104071156));
#19357=CARTESIAN_POINT('Ctrl Pts',(13.8834175105647,11.4529271015425,-5.57015841015681));
#19358=CARTESIAN_POINT('Ctrl Pts',(15.8,12.7922331330237,-6.90058446014691));
#19359=CARTESIAN_POINT('Ctrl Pts',(10.0502525316942,8.69919410795919,-2.87487982939776));
#19360=CARTESIAN_POINT('Ctrl Pts',(11.9668350211294,10.0272667966845,-4.19183584103558));
#19361=CARTESIAN_POINT('Ctrl Pts',(13.8834175105647,11.3553394854098,-5.5087918526734));
#19362=CARTESIAN_POINT('Ctrl Pts',(15.8,12.6834121741351,-6.82574786431123));
#19363=CARTESIAN_POINT('',(15.8,12.6834121741351,-6.82574786431123));
#19364=CARTESIAN_POINT('Ctrl Pts',(15.8,12.7194492253464,-6.84994811524973));
#19365=CARTESIAN_POINT('Ctrl Pts',(15.8,12.7121990649934,-6.84519519909218));
#19366=CARTESIAN_POINT('Ctrl Pts',(15.8,12.7049702849691,-6.84039870583253));
#19367=CARTESIAN_POINT('Ctrl Pts',(15.8,12.6977628786185,-6.83555864794507));
#19368=CARTESIAN_POINT('Ctrl Pts',(15.8,12.6905768416977,-6.83067503400497));
#19369=CARTESIAN_POINT('Ctrl Pts',(15.8,12.6834121741351,-6.82574786431123));
#19370=CARTESIAN_POINT('Ctrl Pts',(10.0502525316942,8.69919410795919,-2.87487982939776));
#19371=CARTESIAN_POINT('Ctrl Pts',(10.2643339107007,8.85499138412423,-3.02539831429572));
#19372=CARTESIAN_POINT('Ctrl Pts',(10.4809652372448,9.01135162140509,-3.17730962520325));
#19373=CARTESIAN_POINT('Ctrl Pts',(10.6991643144455,9.16765819773425,-3.32988591467729));
#19374=CARTESIAN_POINT('Ctrl Pts',(10.8996105956421,9.31124758570826,-3.47004851397053));
#19375=CARTESIAN_POINT('Ctrl Pts',(11.1013798991828,9.45479172976614,-3.61077172321218));
#19376=CARTESIAN_POINT('Ctrl Pts',(11.3037107883209,9.59785289528413,-3.75150991597921));
#19377=CARTESIAN_POINT('Ctrl Pts',(11.5002306637608,9.73680529423647,-3.88820605876814));
#19378=CARTESIAN_POINT('Ctrl Pts',(11.6972803301583,9.8753020317765,-4.02491580697293));
#19379=CARTESIAN_POINT('Ctrl Pts',(11.894162090759,10.0129819298195,-4.16116553050558));
#19380=CARTESIAN_POINT('Ctrl Pts',(12.0857947176331,10.146991095774,-4.29378265233427));
#19381=CARTESIAN_POINT('Ctrl Pts',(12.2772682725492,10.280226529135,-4.42596360023171));
#19382=CARTESIAN_POINT('Ctrl Pts',(12.4679393887634,10.4123927004731,-4.55730333099484));
#19383=CARTESIAN_POINT('Ctrl Pts',(12.6135640193747,10.5133343127246,-4.65761375113995));
#19384=CARTESIAN_POINT('Ctrl Pts',(12.7587205789995,10.6136529851627,-4.757434090911));
#19385=CARTESIAN_POINT('Ctrl Pts',(12.9031224463839,10.7132315216404,-4.85659852260819));
#19386=CARTESIAN_POINT('Ctrl Pts',(13.1606459493128,10.8908179614475,-5.03344645594301));
#19387=CARTESIAN_POINT('Ctrl Pts',(13.420203670549,11.0690158561354,-5.21120255608668));
#19388=CARTESIAN_POINT('Ctrl Pts',(13.6810302954762,11.2473763358668,-5.38931783262601));
#19389=CARTESIAN_POINT('Ctrl Pts',(13.9372302778023,11.4225729890751,-5.56427363215042));
#19390=CARTESIAN_POINT('Ctrl Pts',(14.1946545464806,11.597926588913,-5.73957562566718));
#19391=CARTESIAN_POINT('Ctrl Pts',(14.4525777950785,11.7730460975266,-5.91473898239817));
#19392=CARTESIAN_POINT('Ctrl Pts',(14.7061840816198,11.9452345625907,-6.08697056167663));
#19393=CARTESIAN_POINT('Ctrl Pts',(14.9602727846218,12.1171968581013,-6.25906787671161));
#19394=CARTESIAN_POINT('Ctrl Pts',(15.2141544107006,12.288593051788,-6.43060890607443));
#19395=CARTESIAN_POINT('Ctrl Pts',(15.4096640347459,12.4205821441381,-6.56270953374516));
#19396=CARTESIAN_POINT('Ctrl Pts',(15.6050508567907,12.5522361783515,-6.69448102850577));
#19397=CARTESIAN_POINT('Ctrl Pts',(15.8,12.6834121741351,-6.82574786431123));
#19398=CARTESIAN_POINT('Origin',(15.8,13.8493757942074,-5.91473145421246));
#19399=CARTESIAN_POINT('Origin',(15.8,0.,0.));
#19400=CARTESIAN_POINT('Origin',(13.3251262658471,0.,0.));
#19401=CARTESIAN_POINT('',(15.8,-14.4034641071566,-1.76391562154631E-15));
#19402=CARTESIAN_POINT('',(13.3251262658471,-12.1473403730037,-1.48762015059523E-15));
#19403=CARTESIAN_POINT('Origin',(15.8,0.,0.));
#19404=CARTESIAN_POINT('',(15.8,-14.2731699260464,-1.93297660315714));
#19405=CARTESIAN_POINT('Ctrl Pts',(10.0502525316942,-8.7276078365385,-2.78743136471945));
#19406=CARTESIAN_POINT('Ctrl Pts',(10.264173513818,-8.94196230434565,-2.75725731809585));
#19407=CARTESIAN_POINT('Ctrl Pts',(10.4806406238999,-9.15758913317086,-2.72628853993994));
#19408=CARTESIAN_POINT('Ctrl Pts',(10.698673871089,-9.37356359805418,-2.69475079541967));
#19409=CARTESIAN_POINT('Ctrl Pts',(10.8990914864417,-9.57208876697697,-2.66576109026303));
#19410=CARTESIAN_POINT('Ctrl Pts',(11.1008323950981,-9.77090736500581,-2.63629114159475));
#19411=CARTESIAN_POINT('Ctrl Pts',(11.3031354623541,-9.96934472627367,-2.60652505174282));
#19412=CARTESIAN_POINT('Ctrl Pts',(11.4996395060418,-10.1620938745527,-2.57761220776072));
#19413=CARTESIAN_POINT('Ctrl Pts',(11.6966739416593,-10.3544829963081,-2.54842037280583));
#19414=CARTESIAN_POINT('Ctrl Pts',(11.8935412300419,-10.5459415641124,-2.5191204383414));
#19415=CARTESIAN_POINT('Ctrl Pts',(12.0851664387448,-10.7323020728332,-2.49060068728038));
#19416=CARTESIAN_POINT('Ctrl Pts',(12.2766332831207,-10.917780824147,-2.4619788790975));
#19417=CARTESIAN_POINT('Ctrl Pts',(12.4672984745904,-11.1019006568504,-2.43340900722588));
#19418=CARTESIAN_POINT('Ctrl Pts',(12.6131381170064,-11.2427337599258,-2.41155593658665));
#19419=CARTESIAN_POINT('Ctrl Pts',(12.7585087357906,-11.3827727814342,-2.38973321279001));
#19420=CARTESIAN_POINT('Ctrl Pts',(12.9031224463839,-11.5218245801365,-2.36800640134832));
#19421=CARTESIAN_POINT('Ctrl Pts',(13.1606049656126,-11.7694041995674,-2.3293221429757));
#19422=CARTESIAN_POINT('Ctrl Pts',(13.4201210557269,-12.0180119304344,-2.29026279587101));
#19423=CARTESIAN_POINT('Ctrl Pts',(13.6809057674413,-12.2669622736816,-2.25100860979293));
#19424=CARTESIAN_POINT('Ctrl Pts',(13.9370407316157,-12.5114738741878,-2.21245431924917));
#19425=CARTESIAN_POINT('Ctrl Pts',(14.1943994820694,-12.7563158348609,-2.17371241026527));
#19426=CARTESIAN_POINT('Ctrl Pts',(14.452257261065,-13.0008872910739,-2.13494510077695));
#19427=CARTESIAN_POINT('Ctrl Pts',(14.7057618952069,-13.2413299016104,-2.09683225947821));
#19428=CARTESIAN_POINT('Ctrl Pts',(14.959748850954,-13.4815110518464,-2.0586951448823));
#19429=CARTESIAN_POINT('Ctrl Pts',(15.2135294603815,-13.7209083223233,-2.02067503134479));
#19430=CARTESIAN_POINT('Ctrl Pts',(15.409247662674,-13.9055339464685,-1.99135353081995));
#19431=CARTESIAN_POINT('Ctrl Pts',(15.6048431373525,-14.0896943197621,-1.96210138794136));
#19432=CARTESIAN_POINT('Ctrl Pts',(15.8,-14.2731699260464,-1.93297660315714));
#19433=CARTESIAN_POINT('Origin',(15.8,0.,0.));
#19434=CARTESIAN_POINT('',(15.8,-12.9772686462497,-6.24902206502841));
#19435=CARTESIAN_POINT('Ctrl Pts',(10.0502525316942,-7.43908464225652,-5.34798390487229));
#19436=CARTESIAN_POINT('Ctrl Pts',(10.2641844717857,-7.65228306925312,-5.38552777764328));
#19437=CARTESIAN_POINT('Ctrl Pts',(10.4806628006896,-7.86693728638341,-5.42270898514184));
#19438=CARTESIAN_POINT('Ctrl Pts',(10.698707376949,-8.08209794888593,-5.45945645263813));
#19439=CARTESIAN_POINT('Ctrl Pts',(10.8991296001348,-8.27986933609797,-5.49323399142585));
#19440=CARTESIAN_POINT('Ctrl Pts',(11.1008751331079,-8.47806817158807,-5.52664544938455));
#19441=CARTESIAN_POINT('Ctrl Pts',(11.3031827903456,-8.67599588377849,-5.55965742743711));
#19442=CARTESIAN_POINT('Ctrl Pts',(11.4996891833036,-8.86824792860982,-5.59172277197272));
#19443=CARTESIAN_POINT('Ctrl Pts',(11.6967259244118,-9.06024373107554,-5.62341151149102));
#19444=CARTESIAN_POINT('Ctrl Pts',(11.8935954503941,-9.25138786392987,-5.6547098697144));
#19445=CARTESIAN_POINT('Ctrl Pts',(12.0852214237498,-9.43744093804922,-5.68517460684961));
#19446=CARTESIAN_POINT('Ctrl Pts',(12.2766889707919,-9.62268689886093,-5.71526979467393));
#19447=CARTESIAN_POINT('Ctrl Pts',(12.4673547949393,-9.80662434960534,-5.74499444015009));
#19448=CARTESIAN_POINT('Ctrl Pts',(12.6131755431569,-9.94729925457443,-5.76772777509996));
#19449=CARTESIAN_POINT('Ctrl Pts',(12.7585273514378,-10.0872097382665,-5.79024463999435));
#19450=CARTESIAN_POINT('Ctrl Pts',(12.9031224463839,-10.2261519303672,-5.8125477073404));
#19451=CARTESIAN_POINT('Ctrl Pts',(13.1606063925815,-10.4735696171757,-5.85226331314787));
#19452=CARTESIAN_POINT('Ctrl Pts',(13.4201239322048,-10.7220810242639,-5.89193988397439));
#19453=CARTESIAN_POINT('Ctrl Pts',(13.6809101032503,-10.9709784873109,-5.93153701929334));
#19454=CARTESIAN_POINT('Ctrl Pts',(13.9370453939768,-11.2154370941575,-5.97042797630306));
#19455=CARTESIAN_POINT('Ctrl Pts',(14.1944044698815,-11.4602678697434,-6.00924257976788));
#19456=CARTESIAN_POINT('Ctrl Pts',(14.4522625705723,-11.7048492224773,-6.04794943640073));
#19457=CARTESIAN_POINT('Ctrl Pts',(14.7057648093973,-11.9452989904962,-6.0860024383736));
#19458=CARTESIAN_POINT('Ctrl Pts',(14.9597493558793,-12.1855075942054,-6.12395156273417));
#19459=CARTESIAN_POINT('Ctrl Pts',(15.2135275616695,-12.4249345376281,-6.161769739539));
#19460=CARTESIAN_POINT('Ctrl Pts',(15.4092463976598,-12.6095853925961,-6.19093587506459));
#19461=CARTESIAN_POINT('Ctrl Pts',(15.6048425062638,-12.7937723284765,-6.22002420721651));
#19462=CARTESIAN_POINT('Ctrl Pts',(15.8,-12.9772686462497,-6.24902206502841));
#19463=CARTESIAN_POINT('Origin',(15.8,0.,0.));
#19464=CARTESIAN_POINT('',(15.8,-10.4110618934108,-9.95336970767779));
#19465=CARTESIAN_POINT('Ctrl Pts',(10.0502525316942,-5.42237201204004,-7.38503851882133));
#19466=CARTESIAN_POINT('Ctrl Pts',(10.2643288579052,-5.61366308893708,-7.48669536435437));
#19467=CARTESIAN_POINT('Ctrl Pts',(10.4809550112864,-5.80645273316172,-7.58845719931412));
#19468=CARTESIAN_POINT('Ctrl Pts',(10.6991488645012,-5.99985821934016,-7.68996252980186));
#19469=CARTESIAN_POINT('Ctrl Pts',(10.8995930832247,-6.17753055521342,-7.78321060423707));
#19470=CARTESIAN_POINT('Ctrl Pts',(11.1013603175266,-6.35572208965081,-7.87624242157236));
#19471=CARTESIAN_POINT('Ctrl Pts',(11.3036891533892,-6.53377864760382,-7.96881028742162));
#19472=CARTESIAN_POINT('Ctrl Pts',(11.5002079767431,-6.70672218830172,-8.05872000295732));
#19473=CARTESIAN_POINT('Ctrl Pts',(11.6972566111945,-6.87953788100752,-8.14819216766752));
#19474=CARTESIAN_POINT('Ctrl Pts',(11.8941373707806,-7.05166367276733,-8.23702964306178));
#19475=CARTESIAN_POINT('Ctrl Pts',(12.0857696450343,-7.21920090191052,-8.3234988718709));
#19476=CARTESIAN_POINT('Ctrl Pts',(12.2772428756022,-7.38608422872214,-8.40936703342021));
#19477=CARTESIAN_POINT('Ctrl Pts',(12.4679136994295,-7.55183711206722,-8.49447822756625));
#19478=CARTESIAN_POINT('Ctrl Pts',(12.6135469482004,-7.67843818511105,-8.55948565482468));
#19479=CARTESIAN_POINT('Ctrl Pts',(12.7587120877915,-7.80438059757197,-8.62405202694648));
#19480=CARTESIAN_POINT('Ctrl Pts',(12.9031224463839,-7.92947038823661,-8.6881171163106));
#19481=CARTESIAN_POINT('Ctrl Pts',(13.1606452635188,-8.15253939520241,-8.80236253785699));
#19482=CARTESIAN_POINT('Ctrl Pts',(13.4202022881267,-8.3766610601629,-8.91690884941369));
#19483=CARTESIAN_POINT('Ctrl Pts',(13.6810282117054,-8.60117456124536,-9.0314987989449));
#19484=CARTESIAN_POINT('Ctrl Pts',(13.937228015869,-8.82170599546866,-9.14405633243777));
#19485=CARTESIAN_POINT('Ctrl Pts',(14.1946521067119,-9.04261517808339,-9.25665615329598));
#19486=CARTESIAN_POINT('Ctrl Pts',(14.4525751792582,-9.26332017445258,-9.36907618196659));
#19487=CARTESIAN_POINT('Ctrl Pts',(14.7061825726142,-9.48033224040404,-9.47961515062375));
#19488=CARTESIAN_POINT('Ctrl Pts',(14.9602723890249,-9.69714672451326,-9.58998050800325));
#19489=CARTESIAN_POINT('Ctrl Pts',(15.214155126052,-9.91325721198007,-9.69997936662343));
#19490=CARTESIAN_POINT('Ctrl Pts',(15.4096645113473,-10.0796790374861,-9.78468701348377));
#19491=CARTESIAN_POINT('Ctrl Pts',(15.6050510945576,-10.245684303594,-9.86917770785167));
#19492=CARTESIAN_POINT('Ctrl Pts',(15.8,-10.4110618934108,-9.95336970767779));
#19493=CARTESIAN_POINT('Origin',(15.8,0.,0.));
#19494=CARTESIAN_POINT('',(15.8,-6.82574786431122,-12.6834121741351));
#19495=CARTESIAN_POINT('Ctrl Pts',(10.0502525316942,-2.87487982939776,-8.69919410795919));
#19496=CARTESIAN_POINT('Ctrl Pts',(10.2643339107008,-3.0253983142958,-8.8549913841243));
#19497=CARTESIAN_POINT('Ctrl Pts',(10.480965237245,-3.1773096252034,-9.01135162140524));
#19498=CARTESIAN_POINT('Ctrl Pts',(10.6991643144458,-3.32988591467752,-9.16765819773448));
#19499=CARTESIAN_POINT('Ctrl Pts',(10.8996105956425,-3.47004851397084,-9.31124758570858));
#19500=CARTESIAN_POINT('Ctrl Pts',(11.1013798991834,-3.61077172321258,-9.45479172976655));
#19501=CARTESIAN_POINT('Ctrl Pts',(11.3037107883216,-3.7515099159797,-9.59785289528462));
#19502=CARTESIAN_POINT('Ctrl Pts',(11.5002306637614,-3.88820605876857,-9.73680529423691));
#19503=CARTESIAN_POINT('Ctrl Pts',(11.6972803301588,-4.0249158069733,-9.87530203177688));
#19504=CARTESIAN_POINT('Ctrl Pts',(11.8941620907594,-4.16116553050589,-10.0129819298199));
#19505=CARTESIAN_POINT('Ctrl Pts',(12.0857947176337,-4.29378265233467,-10.1469910957744));
#19506=CARTESIAN_POINT('Ctrl Pts',(12.2772682725499,-4.42596360023219,-10.2802265291355));
#19507=CARTESIAN_POINT('Ctrl Pts',(12.4679393887642,-4.5573033309954,-10.4123927004737));
#19508=CARTESIAN_POINT('Ctrl Pts',(12.6135640193753,-4.65761375114032,-10.513334312725));
#19509=CARTESIAN_POINT('Ctrl Pts',(12.7587205789998,-4.75743409091118,-10.6136529851628));
#19510=CARTESIAN_POINT('Ctrl Pts',(12.9031224463839,-4.85659852260819,-10.7132315216404));
#19511=CARTESIAN_POINT('Ctrl Pts',(13.1606459493135,-5.03344645594353,-10.890817961448));
#19512=CARTESIAN_POINT('Ctrl Pts',(13.4202036705505,-5.21120255608771,-11.0690158561365));
#19513=CARTESIAN_POINT('Ctrl Pts',(13.6810302954785,-5.38931783262757,-11.2473763358684));
#19514=CARTESIAN_POINT('Ctrl Pts',(13.9372302778055,-5.56427363215257,-11.4225729890772));
#19515=CARTESIAN_POINT('Ctrl Pts',(14.1946545464847,-5.73957562566993,-11.5979265889158));
#19516=CARTESIAN_POINT('Ctrl Pts',(14.4525777950835,-5.91473898240153,-11.77304609753));
#19517=CARTESIAN_POINT('Ctrl Pts',(14.7061840816238,-6.08697056167934,-11.9452345625935));
#19518=CARTESIAN_POINT('Ctrl Pts',(14.9602727846248,-6.25906787671367,-12.1171968581034));
#19519=CARTESIAN_POINT('Ctrl Pts',(15.2141544107027,-6.43060890607586,-12.2885930517895));
#19520=CARTESIAN_POINT('Ctrl Pts',(15.4096640347473,-6.5627095337461,-12.420582144139));
#19521=CARTESIAN_POINT('Ctrl Pts',(15.6050508567914,-6.69448102850624,-12.5522361783519));
#19522=CARTESIAN_POINT('Ctrl Pts',(15.8,-6.82574786431122,-12.6834121741351));
#19523=CARTESIAN_POINT('Origin',(15.8,0.,0.));
#19524=CARTESIAN_POINT('',(15.8,-2.57228207647107,-14.1719138864591));
#19525=CARTESIAN_POINT('Ctrl Pts',(10.0502525316942,-0.0459743785884374,
-9.16181196696065));
#19526=CARTESIAN_POINT('Ctrl Pts',(10.264326876663,-0.140978836812287,-9.35649035475255));
#19527=CARTESIAN_POINT('Ctrl Pts',(10.4809510016056,-0.237133935918953,
-9.5521345005741));
#19528=CARTESIAN_POINT('Ctrl Pts',(10.6991428064537,-0.333938024044761,
-9.74793311715205));
#19529=CARTESIAN_POINT('Ctrl Pts',(10.8995862170308,-0.422867769115888,
-9.92780487044956));
#19530=CARTESIAN_POINT('Ctrl Pts',(11.1013526405408,-0.512344667508658,
-10.1078068504782));
#19531=CARTESIAN_POINT('Ctrl Pts',(11.3036806718717,-0.601985074146152,
-10.2873541596189));
#19532=CARTESIAN_POINT('Ctrl Pts',(11.5001990829626,-0.68905155804391,-10.4617459711532));
#19533=CARTESIAN_POINT('Ctrl Pts',(11.6972473130473,-0.776271799836001,
-10.6357086581847));
#19534=CARTESIAN_POINT('Ctrl Pts',(11.8941276803915,-0.863306965607525,
-10.8087523681166));
#19535=CARTESIAN_POINT('Ctrl Pts',(12.085759816357,-0.948022038755198,-10.9771832594084));
#19536=CARTESIAN_POINT('Ctrl Pts',(12.2772329197195,-1.03256139616049,-11.1447435310826));
#19537=CARTESIAN_POINT('Ctrl Pts',(12.4679036288711,-1.11663114425741,-11.3110269536994));
#19538=CARTESIAN_POINT('Ctrl Pts',(12.6135402560747,-1.18084464940027,-11.4380362722128));
#19539=CARTESIAN_POINT('Ctrl Pts',(12.7587087591266,-1.24478452215388,-11.5643015880921));
#19540=CARTESIAN_POINT('Ctrl Pts',(12.9031224463839,-1.30832923723674,-11.6896601572689));
#19541=CARTESIAN_POINT('Ctrl Pts',(13.1606449942899,-1.42164395999531,-11.9132030828002));
#19542=CARTESIAN_POINT('Ctrl Pts',(13.4202017454155,-1.53563343890944,-12.1376081682871));
#19543=CARTESIAN_POINT('Ctrl Pts',(13.6810273936587,-1.64991426889728,-12.362278873202));
#19544=CARTESIAN_POINT('Ctrl Pts',(13.9372271276778,-1.7621682532871,-12.5829648955651));
#19545=CARTESIAN_POINT('Ctrl Pts',(14.1946511485027,-1.87470298591064,-12.8039071645252));
#19546=CARTESIAN_POINT('Ctrl Pts',(14.4525741517311,-1.98717820849243,-13.0245839618714));
#19547=CARTESIAN_POINT('Ctrl Pts',(14.706181979136,-2.09777166653541,-13.2415687303223));
#19548=CARTESIAN_POINT('Ctrl Pts',(14.9602722321832,-2.208307324337,-13.4582969085261));
#19549=CARTESIAN_POINT('Ctrl Pts',(15.2141554048834,-2.31848885998534,-13.6743147818034));
#19550=CARTESIAN_POINT('Ctrl Pts',(15.4096646971182,-2.40333699632634,-13.8406649225605));
#19551=CARTESIAN_POINT('Ctrl Pts',(15.605051187235,-2.48797565175804,-14.006594698047));
#19552=CARTESIAN_POINT('Ctrl Pts',(15.8,-2.57228207647107,-14.1719138864591));
#19553=CARTESIAN_POINT('Origin',(15.8,0.,0.));
#19554=CARTESIAN_POINT('',(15.8,1.93297660315714,-14.2731699260464));
#19555=CARTESIAN_POINT('Ctrl Pts',(10.0502525316942,2.78743136471945,-8.7276078365385));
#19556=CARTESIAN_POINT('Ctrl Pts',(10.2641735138176,2.75725731809591,-8.94196230434529));
#19557=CARTESIAN_POINT('Ctrl Pts',(10.4806406238992,2.72628853994005,-9.15758913317012));
#19558=CARTESIAN_POINT('Ctrl Pts',(10.6986738710879,2.69475079541983,-9.37356359805307));
#19559=CARTESIAN_POINT('Ctrl Pts',(10.8990914864407,2.66576109026318,-9.57208876697593));
#19560=CARTESIAN_POINT('Ctrl Pts',(11.1008323950971,2.6362911415949,-9.77090736500485));
#19561=CARTESIAN_POINT('Ctrl Pts',(11.3031354623532,2.60652505174295,-9.96934472627279));
#19562=CARTESIAN_POINT('Ctrl Pts',(11.4996395060404,2.57761220776094,-10.1620938745513));
#19563=CARTESIAN_POINT('Ctrl Pts',(11.6966739416573,2.54842037280613,-10.3544829963061));
#19564=CARTESIAN_POINT('Ctrl Pts',(11.8935412300393,2.51912043834178,-10.5459415641099));
#19565=CARTESIAN_POINT('Ctrl Pts',(12.0851664387422,2.49060068728077,-10.7323020728307));
#19566=CARTESIAN_POINT('Ctrl Pts',(12.2766332831182,2.46197887909788,-10.9177808241445));
#19567=CARTESIAN_POINT('Ctrl Pts',(12.4672984745878,2.43340900722626,-11.1019006568479));
#19568=CARTESIAN_POINT('Ctrl Pts',(12.6131381170047,2.41155593658691,-11.2427337599242));
#19569=CARTESIAN_POINT('Ctrl Pts',(12.7585087357897,2.38973321279013,-11.3827727814334));
#19570=CARTESIAN_POINT('Ctrl Pts',(12.9031224463839,2.36800640134832,-11.5218245801365));
#19571=CARTESIAN_POINT('Ctrl Pts',(13.1606049656123,2.32932214297574,-11.7694041995672));
#19572=CARTESIAN_POINT('Ctrl Pts',(13.4201210557264,2.29026279587107,-12.0180119304339));
#19573=CARTESIAN_POINT('Ctrl Pts',(13.6809057674406,2.25100860979303,-12.2669622736809));
#19574=CARTESIAN_POINT('Ctrl Pts',(13.9370407316146,2.21245431924935,-12.5114738741867));
#19575=CARTESIAN_POINT('Ctrl Pts',(14.1943994820677,2.17371241026553,-12.7563158348593));
#19576=CARTESIAN_POINT('Ctrl Pts',(14.4522572610628,2.13494510077728,-13.0008872910718));
#19577=CARTESIAN_POINT('Ctrl Pts',(14.7057618952057,2.09683225947839,-13.2413299016093));
#19578=CARTESIAN_POINT('Ctrl Pts',(14.9597488509538,2.05869514488233,-13.4815110518462));
#19579=CARTESIAN_POINT('Ctrl Pts',(15.2135294603822,2.02067503134467,-13.720908322324));
#19580=CARTESIAN_POINT('Ctrl Pts',(15.4092476626745,1.99135353081987,-13.905533946469));
#19581=CARTESIAN_POINT('Ctrl Pts',(15.6048431373528,1.96210138794132,-14.0896943197624));
#19582=CARTESIAN_POINT('Ctrl Pts',(15.8,1.93297660315714,-14.2731699260464));
#19583=CARTESIAN_POINT('Origin',(15.8,0.,0.));
#19584=CARTESIAN_POINT('',(15.8,6.24902206502841,-12.9772686462497));
#19585=CARTESIAN_POINT('Ctrl Pts',(10.0502525316942,5.34798390487229,-7.43908464225652));
#19586=CARTESIAN_POINT('Ctrl Pts',(10.2641844717853,5.3855277776432,-7.65228306925269));
#19587=CARTESIAN_POINT('Ctrl Pts',(10.4806628006887,5.42270898514168,-7.86693728638252));
#19588=CARTESIAN_POINT('Ctrl Pts',(10.6987073769477,5.4594564526379,-8.0820979488846));
#19589=CARTESIAN_POINT('Ctrl Pts',(10.8991296001334,5.49323399142562,-8.27986933609663));
#19590=CARTESIAN_POINT('Ctrl Pts',(11.1008751331065,5.52664544938432,-8.47806817158671));
#19591=CARTESIAN_POINT('Ctrl Pts',(11.3031827903442,5.55965742743688,-8.67599588377713));
#19592=CARTESIAN_POINT('Ctrl Pts',(11.4996891833017,5.59172277197241,-8.86824792860798));
#19593=CARTESIAN_POINT('Ctrl Pts',(11.6967259244095,5.62341151149064,-9.06024373107324));
#19594=CARTESIAN_POINT('Ctrl Pts',(11.8935954503913,5.65470986971394,-9.25138786392711));
#19595=CARTESIAN_POINT('Ctrl Pts',(12.085221423747,5.68517460684917,-9.43744093804651));
#19596=CARTESIAN_POINT('Ctrl Pts',(12.2766889707892,5.7152697946735,-9.62268689885829));
#19597=CARTESIAN_POINT('Ctrl Pts',(12.4673547949366,5.74499444014967,-9.80662434960277));
#19598=CARTESIAN_POINT('Ctrl Pts',(12.6131755431551,5.76772777509968,-9.94729925457273));
#19599=CARTESIAN_POINT('Ctrl Pts',(12.758527351437,5.79024463999421,-10.0872097382657));
#19600=CARTESIAN_POINT('Ctrl Pts',(12.9031224463839,5.8125477073404,-10.2261519303672));
#19601=CARTESIAN_POINT('Ctrl Pts',(13.1606063925803,5.85226331314768,-10.4735696171746));
#19602=CARTESIAN_POINT('Ctrl Pts',(13.4201239322024,5.89193988397403,-10.7220810242616));
#19603=CARTESIAN_POINT('Ctrl Pts',(13.6809101032468,5.9315370192928,-10.9709784873075));
#19604=CARTESIAN_POINT('Ctrl Pts',(13.9370453939728,5.97042797630244,-11.2154370941536));
#19605=CARTESIAN_POINT('Ctrl Pts',(14.1944044698769,6.00924257976718,-11.460267869739));
#19606=CARTESIAN_POINT('Ctrl Pts',(14.4522625705671,6.04794943639995,-11.7048492224724));
#19607=CARTESIAN_POINT('Ctrl Pts',(14.7057648093914,6.08600243837271,-11.9452989904906));
#19608=CARTESIAN_POINT('Ctrl Pts',(14.9597493558726,6.12395156273317,-12.1855075941991));
#19609=CARTESIAN_POINT('Ctrl Pts',(15.2135275616621,6.1617697395379,-12.4249345376211));
#19610=CARTESIAN_POINT('Ctrl Pts',(15.4092463976549,6.19093587506385,-12.6095853925914));
#19611=CARTESIAN_POINT('Ctrl Pts',(15.6048425062613,6.22002420721614,-12.7937723284742));
#19612=CARTESIAN_POINT('Ctrl Pts',(15.8,6.24902206502841,-12.9772686462497));
#19613=CARTESIAN_POINT('Origin',(15.8,0.,0.));
#19614=CARTESIAN_POINT('',(15.8,9.95336970767779,-10.4110618934108));
#19615=CARTESIAN_POINT('Ctrl Pts',(10.0502525316942,7.38503851882133,-5.42237201204004));
#19616=CARTESIAN_POINT('Ctrl Pts',(10.264328857905,7.48669536435428,-5.6136630889369));
#19617=CARTESIAN_POINT('Ctrl Pts',(10.480955011286,7.58845719931394,-5.80645273316137));
#19618=CARTESIAN_POINT('Ctrl Pts',(10.6991488645006,7.68996252980158,-5.99985821933963));
#19619=CARTESIAN_POINT('Ctrl Pts',(10.899593083224,7.78321060423679,-6.17753055521289));
#19620=CARTESIAN_POINT('Ctrl Pts',(11.101360317526,7.87624242157207,-6.35572208965026));
#19621=CARTESIAN_POINT('Ctrl Pts',(11.3036891533886,7.96881028742134,-6.53377864760327));
#19622=CARTESIAN_POINT('Ctrl Pts',(11.500207976743,8.05872000295729,-6.70672218830166));
#19623=CARTESIAN_POINT('Ctrl Pts',(11.697256611195,8.14819216766774,-6.87953788100794));
#19624=CARTESIAN_POINT('Ctrl Pts',(11.8941373707816,8.23702964306225,-7.05166367276824));
#19625=CARTESIAN_POINT('Ctrl Pts',(12.0857696450356,8.32349887187146,-7.21920090191162));
#19626=CARTESIAN_POINT('Ctrl Pts',(12.2772428756036,8.40936703342087,-7.38608422872343));
#19627=CARTESIAN_POINT('Ctrl Pts',(12.4679136994312,8.494478227567,-7.55183711206869));
#19628=CARTESIAN_POINT('Ctrl Pts',(12.6135469482015,8.55948565482517,-7.67843818511202));
#19629=CARTESIAN_POINT('Ctrl Pts',(12.7587120877921,8.62405202694672,-7.80438059757245));
#19630=CARTESIAN_POINT('Ctrl Pts',(12.9031224463839,8.6881171163106,-7.92947038823661));
#19631=CARTESIAN_POINT('Ctrl Pts',(13.1606452635172,8.80236253785629,-8.15253939520104));
#19632=CARTESIAN_POINT('Ctrl Pts',(13.4202022881236,8.9169088494123,-8.37666106016016));
#19633=CARTESIAN_POINT('Ctrl Pts',(13.6810282117006,9.0314987989428,-8.60117456124125));
#19634=CARTESIAN_POINT('Ctrl Pts',(13.9372280158639,9.14405633243554,-8.82170599546428));
#19635=CARTESIAN_POINT('Ctrl Pts',(14.1946521067064,9.2566561532936,-9.04261517807873));
#19636=CARTESIAN_POINT('Ctrl Pts',(14.4525751792524,9.36907618196407,-9.26332017444764));
#19637=CARTESIAN_POINT('Ctrl Pts',(14.7061825726071,9.47961515062067,-9.480332240398));
#19638=CARTESIAN_POINT('Ctrl Pts',(14.9602723890165,9.58998050799961,-9.69714672450612));
#19639=CARTESIAN_POINT('Ctrl Pts',(15.2141551260423,9.69997936661923,-9.91325721197182));
#19640=CARTESIAN_POINT('Ctrl Pts',(15.4096645113409,9.78468701348098,-10.0796790374807));
#19641=CARTESIAN_POINT('Ctrl Pts',(15.6050510945544,9.86917770785029,-10.2456843035913));
#19642=CARTESIAN_POINT('Ctrl Pts',(15.8,9.95336970767779,-10.4110618934108));
#19643=CARTESIAN_POINT('Origin',(15.8,0.,0.));
#19644=CARTESIAN_POINT('',(15.8,14.1719138864591,-2.57228207647107));
#19645=CARTESIAN_POINT('Ctrl Pts',(10.0502525316942,9.16181196696065,-0.0459743785884358));
#19646=CARTESIAN_POINT('Ctrl Pts',(10.2643268766626,9.35649035475223,-0.14097883681213));
#19647=CARTESIAN_POINT('Ctrl Pts',(10.4809510016049,9.55213450057347,-0.237133935918637));
#19648=CARTESIAN_POINT('Ctrl Pts',(10.6991428064526,9.74793311715109,-0.333938024044286));
#19649=CARTESIAN_POINT('Ctrl Pts',(10.8995862170298,9.92780487044862,-0.42286776911542));
#19650=CARTESIAN_POINT('Ctrl Pts',(11.1013526405398,10.1078068504773,-0.512344667508198));
#19651=CARTESIAN_POINT('Ctrl Pts',(11.3036806718707,10.287354159618,-0.601985074145701));
#19652=CARTESIAN_POINT('Ctrl Pts',(11.5001990829614,10.4617459711522,-0.689051558043394));
#19653=CARTESIAN_POINT('Ctrl Pts',(11.6972473130459,10.6357086581835,-0.776271799835421));
#19654=CARTESIAN_POINT('Ctrl Pts',(11.8941276803901,10.8087523681153,-0.863306965606881));
#19655=CARTESIAN_POINT('Ctrl Pts',(12.0857598163557,10.9771832594073,-0.948022038754629));
#19656=CARTESIAN_POINT('Ctrl Pts',(12.2772329197184,11.1447435310816,-1.03256139615999));
#19657=CARTESIAN_POINT('Ctrl Pts',(12.4679036288701,11.3110269536986,-1.11663114425699));
#19658=CARTESIAN_POINT('Ctrl Pts',(12.6135402560741,11.4380362722123,-1.18084464939999));
#19659=CARTESIAN_POINT('Ctrl Pts',(12.7587087591263,11.5643015880918,-1.24478452215374));
#19660=CARTESIAN_POINT('Ctrl Pts',(12.9031224463839,11.6896601572689,-1.30832923723674));
#19661=CARTESIAN_POINT('Ctrl Pts',(13.1606449942899,11.9132030828002,-1.42164395999531));
#19662=CARTESIAN_POINT('Ctrl Pts',(13.4202017454155,12.1376081682871,-1.53563343890943));
#19663=CARTESIAN_POINT('Ctrl Pts',(13.6810273936587,12.362278873202,-1.64991426889727));
#19664=CARTESIAN_POINT('Ctrl Pts',(13.9372271276793,12.5829648955663,-1.76216825328775));
#19665=CARTESIAN_POINT('Ctrl Pts',(14.1946511485057,12.8039071645278,-1.87470298591195));
#19666=CARTESIAN_POINT('Ctrl Pts',(14.4525741517356,13.0245839618753,-1.98717820849441));
#19667=CARTESIAN_POINT('Ctrl Pts',(14.7061819791402,13.2415687303259,-2.09777166653724));
#19668=CARTESIAN_POINT('Ctrl Pts',(14.9602722321871,13.4582969085294,-2.20830732433869));
#19669=CARTESIAN_POINT('Ctrl Pts',(15.214155404887,13.6743147818064,-2.31848885998689));
#19670=CARTESIAN_POINT('Ctrl Pts',(15.4096646971206,13.8406649225625,-2.40333699632737));
#19671=CARTESIAN_POINT('Ctrl Pts',(15.6050511872361,14.006594698048,-2.48797565175855));
#19672=CARTESIAN_POINT('Ctrl Pts',(15.8,14.1719138864591,-2.57228207647107));
#19673=CARTESIAN_POINT('Origin',(15.8,0.,0.));
#19674=CARTESIAN_POINT('',(15.8,14.2731699260464,1.93297660315714));
#19675=CARTESIAN_POINT('Ctrl Pts',(10.0502525316942,8.7276078365385,2.78743136471945));
#19676=CARTESIAN_POINT('Ctrl Pts',(10.2641735138176,8.94196230434521,2.75725731809592));
#19677=CARTESIAN_POINT('Ctrl Pts',(10.480640623899,9.15758913316998,2.72628853994007));
#19678=CARTESIAN_POINT('Ctrl Pts',(10.6986738710877,9.37356359805285,2.69475079541987));
#19679=CARTESIAN_POINT('Ctrl Pts',(10.8990914864403,9.57208876697557,2.66576109026324));
#19680=CARTESIAN_POINT('Ctrl Pts',(11.1008323950966,9.77090736500434,2.63629114159498));
#19681=CARTESIAN_POINT('Ctrl Pts',(11.3031354623526,9.96934472627213,2.60652505174305));
#19682=CARTESIAN_POINT('Ctrl Pts',(11.4996395060398,10.1620938745508,2.57761220776102));
#19683=CARTESIAN_POINT('Ctrl Pts',(11.6966739416569,10.3544829963057,2.54842037280618));
#19684=CARTESIAN_POINT('Ctrl Pts',(11.8935412300391,10.5459415641097,2.51912043834181));
#19685=CARTESIAN_POINT('Ctrl Pts',(12.0851664387418,10.7323020728303,2.49060068728083));
#19686=CARTESIAN_POINT('Ctrl Pts',(12.2766332831176,10.9177808241439,2.46197887909798));
#19687=CARTESIAN_POINT('Ctrl Pts',(12.467298474587,11.1019006568471,2.43340900722639));
#19688=CARTESIAN_POINT('Ctrl Pts',(12.6131381170041,11.2427337599237,2.41155593658699));
#19689=CARTESIAN_POINT('Ctrl Pts',(12.7585087357895,11.3827727814331,2.38973321279018));
#19690=CARTESIAN_POINT('Ctrl Pts',(12.9031224463839,11.5218245801365,2.36800640134832));
#19691=CARTESIAN_POINT('Ctrl Pts',(13.1606049656125,11.7694041995673,2.32932214297571));
#19692=CARTESIAN_POINT('Ctrl Pts',(13.4201210557268,12.0180119304343,2.29026279587103));
#19693=CARTESIAN_POINT('Ctrl Pts',(13.6809057674411,12.2669622736814,2.25100860979295));
#19694=CARTESIAN_POINT('Ctrl Pts',(13.9370407316154,12.5114738741875,2.21245431924923));
#19695=CARTESIAN_POINT('Ctrl Pts',(14.1943994820688,12.7563158348603,2.17371241026536));
#19696=CARTESIAN_POINT('Ctrl Pts',(14.4522572610642,13.0008872910732,2.13494510077707));
#19697=CARTESIAN_POINT('Ctrl Pts',(14.7057618952067,13.2413299016102,2.09683225947825));
#19698=CARTESIAN_POINT('Ctrl Pts',(14.9597488509542,13.4815110518466,2.05869514488227));
#19699=CARTESIAN_POINT('Ctrl Pts',(15.2135294603822,13.720908322324,2.02067503134468));
#19700=CARTESIAN_POINT('Ctrl Pts',(15.4092476626745,13.9055339464689,1.99135353081988));
#19701=CARTESIAN_POINT('Ctrl Pts',(15.6048431373528,14.0896943197624,1.96210138794133));
#19702=CARTESIAN_POINT('Ctrl Pts',(15.8,14.2731699260464,1.93297660315714));
#19703=CARTESIAN_POINT('Origin',(15.8,0.,0.));
#19704=CARTESIAN_POINT('',(15.8,12.9772686462497,6.24902206502841));
#19705=CARTESIAN_POINT('Ctrl Pts',(10.0502525316942,7.43908464225652,5.34798390487229));
#19706=CARTESIAN_POINT('Ctrl Pts',(10.2641844717852,7.65228306925265,5.3855277776432));
#19707=CARTESIAN_POINT('Ctrl Pts',(10.4806628006887,7.86693728638245,5.42270898514167));
#19708=CARTESIAN_POINT('Ctrl Pts',(10.6987073769475,8.08209794888449,5.45945645263788));
#19709=CARTESIAN_POINT('Ctrl Pts',(10.8991296001334,8.27986933609659,5.49323399142561));
#19710=CARTESIAN_POINT('Ctrl Pts',(11.1008751331065,8.47806817158674,5.52664544938433));
#19711=CARTESIAN_POINT('Ctrl Pts',(11.3031827903443,8.67599588377722,5.5596574274369));
#19712=CARTESIAN_POINT('Ctrl Pts',(11.4996891833021,8.86824792860831,5.59172277197247));
#19713=CARTESIAN_POINT('Ctrl Pts',(11.69672592441,9.06024373107381,5.62341151149074));
#19714=CARTESIAN_POINT('Ctrl Pts',(11.8935954503921,9.25138786392791,5.65470986971407));
#19715=CARTESIAN_POINT('Ctrl Pts',(12.0852214237475,9.43744093804696,5.68517460684925));
#19716=CARTESIAN_POINT('Ctrl Pts',(12.2766889707893,9.62268689885838,5.71526979467352));
#19717=CARTESIAN_POINT('Ctrl Pts',(12.4673547949364,9.80662434960252,5.74499444014963));
#19718=CARTESIAN_POINT('Ctrl Pts',(12.613175543155,9.94729925457255,5.76772777509965));
#19719=CARTESIAN_POINT('Ctrl Pts',(12.7585273514369,10.0872097382656,5.7902446399942));
#19720=CARTESIAN_POINT('Ctrl Pts',(12.9031224463839,10.2261519303672,5.8125477073404));
#19721=CARTESIAN_POINT('Ctrl Pts',(13.1606063925802,10.4735696171745,5.85226331314767));
#19722=CARTESIAN_POINT('Ctrl Pts',(13.4201239322022,10.7220810242614,5.891939883974));
#19723=CARTESIAN_POINT('Ctrl Pts',(13.6809101032465,10.9709784873072,5.93153701929276));
#19724=CARTESIAN_POINT('Ctrl Pts',(13.9370453939728,11.2154370941536,5.97042797630245));
#19725=CARTESIAN_POINT('Ctrl Pts',(14.1944044698772,11.4602678697393,6.00924257976723));
#19726=CARTESIAN_POINT('Ctrl Pts',(14.4522625705678,11.704849222473,6.04794943640006));
#19727=CARTESIAN_POINT('Ctrl Pts',(14.705764809393,11.9452989904921,6.08600243837295));
#19728=CARTESIAN_POINT('Ctrl Pts',(14.9597493558751,12.1855075942015,6.12395156273355));
#19729=CARTESIAN_POINT('Ctrl Pts',(15.2135275616656,12.4249345376244,6.16176973953841));
#19730=CARTESIAN_POINT('Ctrl Pts',(15.4092463976572,12.6095853925936,6.19093587506419));
#19731=CARTESIAN_POINT('Ctrl Pts',(15.6048425062625,12.7937723284753,6.22002420721631));
#19732=CARTESIAN_POINT('Ctrl Pts',(15.8,12.9772686462497,6.24902206502841));
#19733=CARTESIAN_POINT('Origin',(15.8,0.,0.));
#19734=CARTESIAN_POINT('',(15.8,10.4110618934108,9.9533697076778));
#19735=CARTESIAN_POINT('Ctrl Pts',(10.0502525316942,5.42237201204004,7.38503851882133));
#19736=CARTESIAN_POINT('Ctrl Pts',(10.2643288579058,5.6136630889376,7.48669536435465));
#19737=CARTESIAN_POINT('Ctrl Pts',(10.4809550112876,5.80645273316278,7.58845719931468));
#19738=CARTESIAN_POINT('Ctrl Pts',(10.699148864503,5.99985821934175,7.68996252980269));
#19739=CARTESIAN_POINT('Ctrl Pts',(10.8995930832264,6.17753055521495,7.78321060423786));
#19740=CARTESIAN_POINT('Ctrl Pts',(11.1013603175282,6.35572208965226,7.87624242157312));
#19741=CARTESIAN_POINT('Ctrl Pts',(11.3036891533908,6.5337786476052,7.96881028742234));
#19742=CARTESIAN_POINT('Ctrl Pts',(11.5002079767454,6.70672218830375,8.05872000295837));
#19743=CARTESIAN_POINT('Ctrl Pts',(11.6972566111975,6.87953788101019,8.1481921676689));
#19744=CARTESIAN_POINT('Ctrl Pts',(11.8941373707844,7.05166367277064,8.23702964306349));
#19745=CARTESIAN_POINT('Ctrl Pts',(12.0857696450381,7.21920090191376,8.32349887187257));
#19746=CARTESIAN_POINT('Ctrl Pts',(12.2772428756058,7.38608422872531,8.40936703342184));
#19747=CARTESIAN_POINT('Ctrl Pts',(12.467913699433,7.55183711207031,8.49447822756784));
#19748=CARTESIAN_POINT('Ctrl Pts',(12.6135469482027,7.6784381851131,8.55948565482573));
#19749=CARTESIAN_POINT('Ctrl Pts',(12.7587120877927,7.80438059757298,8.624052026947));
#19750=CARTESIAN_POINT('Ctrl Pts',(12.9031224463839,7.92947038823661,8.6881171163106));
#19751=CARTESIAN_POINT('Ctrl Pts',(13.1606452635176,8.15253939520139,8.80236253785647));
#19752=CARTESIAN_POINT('Ctrl Pts',(13.4202022881244,8.37666106016085,8.91690884941265));
#19753=CARTESIAN_POINT('Ctrl Pts',(13.6810282117018,8.60117456124228,9.03149879894333));
#19754=CARTESIAN_POINT('Ctrl Pts',(13.9372280158653,8.82170599546549,9.14405633243615));
#19755=CARTESIAN_POINT('Ctrl Pts',(14.1946521067081,9.04261517808011,9.25665615329431));
#19756=CARTESIAN_POINT('Ctrl Pts',(14.4525751792543,9.26332017444921,9.36907618196487));
#19757=CARTESIAN_POINT('Ctrl Pts',(14.7061825726096,9.48033224040016,9.47961515062177));
#19758=CARTESIAN_POINT('Ctrl Pts',(14.9602723890198,9.69714672450887,9.58998050800102));
#19759=CARTESIAN_POINT('Ctrl Pts',(15.2141551260462,9.91325721197517,9.69997936662094));
#19760=CARTESIAN_POINT('Ctrl Pts',(15.4096645113435,10.0796790374829,9.78468701348212));
#19761=CARTESIAN_POINT('Ctrl Pts',(15.6050510945557,10.2456843035924,9.86917770785085));
#19762=CARTESIAN_POINT('Ctrl Pts',(15.8,10.4110618934108,9.9533697076778));
#19763=CARTESIAN_POINT('Origin',(15.8,0.,0.));
#19764=CARTESIAN_POINT('',(15.8,6.82574786431122,12.6834121741351));
#19765=CARTESIAN_POINT('Ctrl Pts',(10.0502525316942,2.87487982939776,8.69919410795919));
#19766=CARTESIAN_POINT('Ctrl Pts',(10.2643339107001,3.02539831429527,8.85499138412376));
#19767=CARTESIAN_POINT('Ctrl Pts',(10.4809652372435,3.17730962520234,9.01135162140416));
#19768=CARTESIAN_POINT('Ctrl Pts',(10.6991643144436,3.32988591467592,9.16765819773286));
#19769=CARTESIAN_POINT('Ctrl Pts',(10.8996105956403,3.47004851396928,9.31124758570699));
#19770=CARTESIAN_POINT('Ctrl Pts',(11.1013798991812,3.61077172321105,9.45479172976499));
#19771=CARTESIAN_POINT('Ctrl Pts',(11.3037107883194,3.7515099159782,9.5978528952831));
#19772=CARTESIAN_POINT('Ctrl Pts',(11.5002306637591,3.88820605876695,9.73680529423527));
#19773=CARTESIAN_POINT('Ctrl Pts',(11.6972803301563,4.02491580697157,9.87530203177513));
#19774=CARTESIAN_POINT('Ctrl Pts',(11.8941620907568,4.16116553050405,10.012981929818));
#19775=CARTESIAN_POINT('Ctrl Pts',(12.085794717631,4.29378265233282,10.1469910957725));
#19776=CARTESIAN_POINT('Ctrl Pts',(12.2772682725472,4.42596360023034,10.2802265291336));
#19777=CARTESIAN_POINT('Ctrl Pts',(12.4679393887615,4.55730333099355,10.4123927004718));
#19778=CARTESIAN_POINT('Ctrl Pts',(12.6135640193735,4.6576137511391,10.5133343127237));
#19779=CARTESIAN_POINT('Ctrl Pts',(12.7587205789989,4.75743409091057,10.6136529851622));
#19780=CARTESIAN_POINT('Ctrl Pts',(12.9031224463839,4.85659852260819,10.7132315216404));
#19781=CARTESIAN_POINT('Ctrl Pts',(13.1606459493138,5.03344645594371,10.8908179614482));
#19782=CARTESIAN_POINT('Ctrl Pts',(13.4202036705511,5.21120255608808,11.0690158561368));
#19783=CARTESIAN_POINT('Ctrl Pts',(13.6810302954793,5.38931783262812,11.2473763358689));
#19784=CARTESIAN_POINT('Ctrl Pts',(13.937230277807,5.56427363215361,11.4225729890783));
#19785=CARTESIAN_POINT('Ctrl Pts',(14.1946545464869,5.73957562567147,11.5979265889173));
#19786=CARTESIAN_POINT('Ctrl Pts',(14.4525777950865,5.91473898240356,11.773046097532));
#19787=CARTESIAN_POINT('Ctrl Pts',(14.7061840816275,6.08697056168185,11.945234562596));
#19788=CARTESIAN_POINT('Ctrl Pts',(14.9602727846292,6.25906787671666,12.1171968581064));
#19789=CARTESIAN_POINT('Ctrl Pts',(15.2141544107078,6.43060890607932,12.2885930517929));
#19790=CARTESIAN_POINT('Ctrl Pts',(15.4096640347508,6.56270953374841,12.4205821441413));
#19791=CARTESIAN_POINT('Ctrl Pts',(15.6050508567931,6.69448102850738,12.5522361783531));
#19792=CARTESIAN_POINT('Ctrl Pts',(15.8,6.82574786431122,12.6834121741351));
#19793=CARTESIAN_POINT('Origin',(15.8,0.,0.));
#19794=CARTESIAN_POINT('',(15.8,2.57228207647107,14.1719138864591));
#19795=CARTESIAN_POINT('Ctrl Pts',(10.0502525316942,0.0459743785884363,
9.16181196696065));
#19796=CARTESIAN_POINT('Ctrl Pts',(10.2643268766632,0.140978836812379,9.35649035475274));
#19797=CARTESIAN_POINT('Ctrl Pts',(10.4809510016061,0.23713393591914,9.55213450057449));
#19798=CARTESIAN_POINT('Ctrl Pts',(10.6991428064543,0.333938024045044,9.74793311715262));
#19799=CARTESIAN_POINT('Ctrl Pts',(10.8995862170315,0.422867769116193,9.92780487045018));
#19800=CARTESIAN_POINT('Ctrl Pts',(11.1013526405416,0.512344667508983,10.1078068504789));
#19801=CARTESIAN_POINT('Ctrl Pts',(11.3036806718725,0.601985074146499,10.2873541596196));
#19802=CARTESIAN_POINT('Ctrl Pts',(11.5001990829629,0.689051558044051,10.4617459711535));
#19803=CARTESIAN_POINT('Ctrl Pts',(11.6972473130471,0.776271799835937,10.6357086581846));
#19804=CARTESIAN_POINT('Ctrl Pts',(11.8941276803909,0.863306965607256,10.8087523681161));
#19805=CARTESIAN_POINT('Ctrl Pts',(12.0857598163565,0.948022038754971,10.9771832594079));
#19806=CARTESIAN_POINT('Ctrl Pts',(12.2772329197191,1.0325613961603,11.1447435310822));
#19807=CARTESIAN_POINT('Ctrl Pts',(12.4679036288708,1.11663114425727,11.3110269536992));
#19808=CARTESIAN_POINT('Ctrl Pts',(12.6135402560745,1.18084464940017,11.4380362722126));
#19809=CARTESIAN_POINT('Ctrl Pts',(12.7587087591265,1.24478452215383,11.564301588092));
#19810=CARTESIAN_POINT('Ctrl Pts',(12.9031224463839,1.30832923723674,11.6896601572689));
#19811=CARTESIAN_POINT('Ctrl Pts',(13.1606449942899,1.42164395999532,11.9132030828002));
#19812=CARTESIAN_POINT('Ctrl Pts',(13.4202017454155,1.53563343890945,12.1376081682871));
#19813=CARTESIAN_POINT('Ctrl Pts',(13.6810273936588,1.64991426889729,12.362278873202));
#19814=CARTESIAN_POINT('Ctrl Pts',(13.9372271276791,1.76216825328766,12.5829648955662));
#19815=CARTESIAN_POINT('Ctrl Pts',(14.1946511485052,1.87470298591175,12.8039071645274));
#19816=CARTESIAN_POINT('Ctrl Pts',(14.4525741517349,1.9871782084941,13.0245839618747));
#19817=CARTESIAN_POINT('Ctrl Pts',(14.7061819791395,2.09777166653694,13.2415687303253));
#19818=CARTESIAN_POINT('Ctrl Pts',(14.9602722321865,2.20830732433841,13.4582969085288));
#19819=CARTESIAN_POINT('Ctrl Pts',(15.2141554048864,2.31848885998662,13.6743147818059));
#19820=CARTESIAN_POINT('Ctrl Pts',(15.4096646971202,2.40333699632719,13.8406649225621));
#19821=CARTESIAN_POINT('Ctrl Pts',(15.6050511872359,2.48797565175846,14.0065946980479));
#19822=CARTESIAN_POINT('Ctrl Pts',(15.8,2.57228207647107,14.1719138864591));
#19823=CARTESIAN_POINT('Origin',(15.8,0.,0.));
#19824=CARTESIAN_POINT('',(15.8,-1.93297660315714,14.2731699260464));
#19825=CARTESIAN_POINT('Ctrl Pts',(10.0502525316942,-2.78743136471945,8.7276078365385));
#19826=CARTESIAN_POINT('Ctrl Pts',(10.2641735138177,-2.75725731809589,8.94196230434538));
#19827=CARTESIAN_POINT('Ctrl Pts',(10.4806406238994,-2.72628853994002,9.15758913317033));
#19828=CARTESIAN_POINT('Ctrl Pts',(10.6986738710882,-2.69475079541979,9.37356359805338));
#19829=CARTESIAN_POINT('Ctrl Pts',(10.899091486441,-2.66576109026313,9.57208876697628));
#19830=CARTESIAN_POINT('Ctrl Pts',(11.1008323950975,-2.63629114159484,9.77090736500523));
#19831=CARTESIAN_POINT('Ctrl Pts',(11.3031354623537,-2.60652505174289,9.9693447262732));
#19832=CARTESIAN_POINT('Ctrl Pts',(11.4996395060412,-2.57761220776082,10.1620938745521));
#19833=CARTESIAN_POINT('Ctrl Pts',(11.6966739416585,-2.54842037280596,10.3544829963072));
#19834=CARTESIAN_POINT('Ctrl Pts',(11.8935412300409,-2.51912043834155,10.5459415641114));
#19835=CARTESIAN_POINT('Ctrl Pts',(12.0851664387437,-2.49060068728054,10.7323020728322));
#19836=CARTESIAN_POINT('Ctrl Pts',(12.2766332831197,-2.46197887909766,10.9177808241459));
#19837=CARTESIAN_POINT('Ctrl Pts',(12.4672984745893,-2.43340900722605,11.1019006568493));
#19838=CARTESIAN_POINT('Ctrl Pts',(12.6131381170056,-2.41155593658676,11.2427337599251));
#19839=CARTESIAN_POINT('Ctrl Pts',(12.7585087357902,-2.38973321279006,11.3827727814338));
#19840=CARTESIAN_POINT('Ctrl Pts',(12.9031224463839,-2.36800640134832,11.5218245801365));
#19841=CARTESIAN_POINT('Ctrl Pts',(13.1606049656133,-2.3293221429756,11.769404199568));
#19842=CARTESIAN_POINT('Ctrl Pts',(13.4201210557283,-2.2902627958708,12.0180119304357));
#19843=CARTESIAN_POINT('Ctrl Pts',(13.6809057674434,-2.25100860979261,12.2669622736836));
#19844=CARTESIAN_POINT('Ctrl Pts',(13.9370407316176,-2.21245431924889,12.5114738741896));
#19845=CARTESIAN_POINT('Ctrl Pts',(14.194399482071,-2.17371241026503,12.7563158348624));
#19846=CARTESIAN_POINT('Ctrl Pts',(14.4522572610663,-2.13494510077675,13.0008872910752));
#19847=CARTESIAN_POINT('Ctrl Pts',(14.7057618952085,-2.09683225947798,13.2413299016119));
#19848=CARTESIAN_POINT('Ctrl Pts',(14.9597488509557,-2.05869514488204,13.481511051848));
#19849=CARTESIAN_POINT('Ctrl Pts',(15.2135294603834,-2.0206750313445,13.7209083223251));
#19850=CARTESIAN_POINT('Ctrl Pts',(15.4092476626753,-1.99135353081976,13.9055339464697));
#19851=CARTESIAN_POINT('Ctrl Pts',(15.6048431373532,-1.96210138794127,14.0896943197627));
#19852=CARTESIAN_POINT('Ctrl Pts',(15.8,-1.93297660315714,14.2731699260464));
#19853=CARTESIAN_POINT('Origin',(15.8,0.,0.));
#19854=CARTESIAN_POINT('',(15.8,-6.24902206502841,12.9772686462497));
#19855=CARTESIAN_POINT('Ctrl Pts',(10.0502525316942,-5.34798390487229,7.43908464225652));
#19856=CARTESIAN_POINT('Ctrl Pts',(10.2641844717849,-5.38552777764315,7.65228306925236));
#19857=CARTESIAN_POINT('Ctrl Pts',(10.4806628006881,-5.42270898514157,7.86693728638186));
#19858=CARTESIAN_POINT('Ctrl Pts',(10.6987073769466,-5.45945645263773,8.08209794888361));
#19859=CARTESIAN_POINT('Ctrl Pts',(10.8991296001323,-5.49323399142543,8.27986933609552));
#19860=CARTESIAN_POINT('Ctrl Pts',(11.1008751331052,-5.52664544938412,8.47806817158548));
#19861=CARTESIAN_POINT('Ctrl Pts',(11.3031827903428,-5.55965742743666,8.67599588377579));
#19862=CARTESIAN_POINT('Ctrl Pts',(11.4996891833007,-5.59172277197224,8.86824792860694));
#19863=CARTESIAN_POINT('Ctrl Pts',(11.6967259244087,-5.62341151149052,9.0602437310725));
#19864=CARTESIAN_POINT('Ctrl Pts',(11.8935954503908,-5.65470986971387,9.25138786392667));
#19865=CARTESIAN_POINT('Ctrl Pts',(12.0852214237466,-5.68517460684912,9.43744093804618));
#19866=CARTESIAN_POINT('Ctrl Pts',(12.2766889707889,-5.71526979467347,9.62268689885806));
#19867=CARTESIAN_POINT('Ctrl Pts',(12.4673547949365,-5.74499444014965,9.80662434960265));
#19868=CARTESIAN_POINT('Ctrl Pts',(12.613175543155,-5.76772777509967,9.94729925457264));
#19869=CARTESIAN_POINT('Ctrl Pts',(12.7585273514369,-5.79024463999421,10.0872097382656));
#19870=CARTESIAN_POINT('Ctrl Pts',(12.9031224463839,-5.8125477073404,10.2261519303672));
#19871=CARTESIAN_POINT('Ctrl Pts',(13.1606063925794,-5.85226331314755,10.4735696171738));
#19872=CARTESIAN_POINT('Ctrl Pts',(13.4201239322007,-5.89193988397376,10.7220810242599));
#19873=CARTESIAN_POINT('Ctrl Pts',(13.6809101032441,-5.93153701929241,10.970978487305));
#19874=CARTESIAN_POINT('Ctrl Pts',(13.9370453939694,-5.97042797630194,11.2154370941504));
#19875=CARTESIAN_POINT('Ctrl Pts',(14.1944044698729,-6.00924257976658,11.4602678697352));
#19876=CARTESIAN_POINT('Ctrl Pts',(14.4522625705624,-6.04794943639925,11.7048492224679));
#19877=CARTESIAN_POINT('Ctrl Pts',(14.7057648093879,-6.08600243837219,11.9452989904873));
#19878=CARTESIAN_POINT('Ctrl Pts',(14.9597493558704,-6.12395156273284,12.185507594197));
#19879=CARTESIAN_POINT('Ctrl Pts',(15.213527561661,-6.16176973953774,12.4249345376201));
#19880=CARTESIAN_POINT('Ctrl Pts',(15.4092463976542,-6.19093587506375,12.6095853925908));
#19881=CARTESIAN_POINT('Ctrl Pts',(15.604842506261,-6.22002420721609,12.7937723284739));
#19882=CARTESIAN_POINT('Ctrl Pts',(15.8,-6.24902206502841,12.9772686462497));
#19883=CARTESIAN_POINT('Origin',(15.8,0.,0.));
#19884=CARTESIAN_POINT('',(15.8,-9.95336970767779,10.4110618934108));
#19885=CARTESIAN_POINT('Ctrl Pts',(10.0502525316942,-7.38503851882133,5.42237201204004));
#19886=CARTESIAN_POINT('Ctrl Pts',(10.2643288579052,-7.48669536435435,5.61366308893702));
#19887=CARTESIAN_POINT('Ctrl Pts',(10.4809550112863,-7.58845719931407,5.80645273316162));
#19888=CARTESIAN_POINT('Ctrl Pts',(10.699148864501,-7.68996252980178,5.99985821934));
#19889=CARTESIAN_POINT('Ctrl Pts',(10.8995930832245,-7.78321060423697,6.17753055521325));
#19890=CARTESIAN_POINT('Ctrl Pts',(11.1013603175263,-7.87624242157225,6.35572208965061));
#19891=CARTESIAN_POINT('Ctrl Pts',(11.3036891533889,-7.96881028742151,6.5337786476036));
#19892=CARTESIAN_POINT('Ctrl Pts',(11.5002079767434,-8.05872000295745,6.70672218830198));
#19893=CARTESIAN_POINT('Ctrl Pts',(11.6972566111953,-8.14819216766789,6.87953788100824));
#19894=CARTESIAN_POINT('Ctrl Pts',(11.8941373707819,-8.23702964306239,7.05166367276852));
#19895=CARTESIAN_POINT('Ctrl Pts',(12.0857696450361,-8.32349887187168,7.21920090191204));
#19896=CARTESIAN_POINT('Ctrl Pts',(12.2772428756043,-8.40936703342116,7.38608422872399));
#19897=CARTESIAN_POINT('Ctrl Pts',(12.467913699432,-8.49447822756735,7.55183711206938));
#19898=CARTESIAN_POINT('Ctrl Pts',(12.613546948202,-8.55948565482541,7.67843818511248));
#19899=CARTESIAN_POINT('Ctrl Pts',(12.7587120877923,-8.62405202694684,7.80438059757268));
#19900=CARTESIAN_POINT('Ctrl Pts',(12.9031224463839,-8.6881171163106,7.92947038823661));
#19901=CARTESIAN_POINT('Ctrl Pts',(13.1606452635168,-8.80236253785607,8.15253939520062));
#19902=CARTESIAN_POINT('Ctrl Pts',(13.4202022881226,-8.91690884941186,8.37666106015931));
#19903=CARTESIAN_POINT('Ctrl Pts',(13.6810282116991,-9.03149879894215,8.60117456123998));
#19904=CARTESIAN_POINT('Ctrl Pts',(13.9372280158629,-9.14405633243508,8.82170599546338));
#19905=CARTESIAN_POINT('Ctrl Pts',(14.1946521067058,-9.25665615329334,9.04261517807822));
#19906=CARTESIAN_POINT('Ctrl Pts',(14.4525751792523,-9.36907618196402,9.26332017444753));
#19907=CARTESIAN_POINT('Ctrl Pts',(14.7061825726078,-9.47961515062096,9.48033224039856));
#19908=CARTESIAN_POINT('Ctrl Pts',(14.960272389018,-9.58998050800025,9.69714672450736));
#19909=CARTESIAN_POINT('Ctrl Pts',(15.2141551260446,-9.69997936662022,9.91325721197376));
#19910=CARTESIAN_POINT('Ctrl Pts',(15.4096645113424,-9.78468701348163,10.0796790374819));
#19911=CARTESIAN_POINT('Ctrl Pts',(15.6050510945551,-9.86917770785061,10.2456843035919));
#19912=CARTESIAN_POINT('Ctrl Pts',(15.8,-9.95336970767779,10.4110618934108));
#19913=CARTESIAN_POINT('Origin',(15.8,0.,0.));
#19914=CARTESIAN_POINT('',(15.8,-12.6834121741351,6.82574786431122));
#19915=CARTESIAN_POINT('Ctrl Pts',(10.0502525316942,-8.69919410795919,2.87487982939776));
#19916=CARTESIAN_POINT('Ctrl Pts',(10.264333910701,-8.85499138412439,3.02539831429588));
#19917=CARTESIAN_POINT('Ctrl Pts',(10.4809652372453,-9.01135162140542,3.17730962520357));
#19918=CARTESIAN_POINT('Ctrl Pts',(10.6991643144462,-9.16765819773475,3.32988591467777));
#19919=CARTESIAN_POINT('Ctrl Pts',(10.8996105956429,-9.31124758570884,3.47004851397109));
#19920=CARTESIAN_POINT('Ctrl Pts',(11.1013798991838,-9.4547917297668,3.61077172321283));
#19921=CARTESIAN_POINT('Ctrl Pts',(11.3037107883219,-9.59785289528487,3.75150991597994));
#19922=CARTESIAN_POINT('Ctrl Pts',(11.5002306637619,-9.73680529423722,3.88820605876887));
#19923=CARTESIAN_POINT('Ctrl Pts',(11.6972803301593,-9.87530203177726,4.02491580697367));
#19924=CARTESIAN_POINT('Ctrl Pts',(11.8941620907601,-10.0129819298203,4.16116553050634));
#19925=CARTESIAN_POINT('Ctrl Pts',(12.0857947176342,-10.1469910957747,4.29378265233503));
#19926=CARTESIAN_POINT('Ctrl Pts',(12.2772682725503,-10.2802265291358,4.42596360023247));
#19927=CARTESIAN_POINT('Ctrl Pts',(12.4679393887645,-10.4123927004739,4.55730333099561));
#19928=CARTESIAN_POINT('Ctrl Pts',(12.6135640193755,-10.5133343127251,4.65761375114046));
#19929=CARTESIAN_POINT('Ctrl Pts',(12.7587205789999,-10.6136529851629,4.75743409091125));
#19930=CARTESIAN_POINT('Ctrl Pts',(12.9031224463839,-10.7132315216404,4.85659852260819));
#19931=CARTESIAN_POINT('Ctrl Pts',(13.1606459493129,-10.8908179614476,5.03344645594312));
#19932=CARTESIAN_POINT('Ctrl Pts',(13.4202036705494,-11.0690158561357,5.2112025560869));
#19933=CARTESIAN_POINT('Ctrl Pts',(13.6810302954767,-11.2473763358671,5.38931783262634));
#19934=CARTESIAN_POINT('Ctrl Pts',(13.9372302778033,-11.4225729890757,5.56427363215107));
#19935=CARTESIAN_POINT('Ctrl Pts',(14.1946545464821,-11.597926588914,5.73957562566816));
#19936=CARTESIAN_POINT('Ctrl Pts',(14.4525777950805,-11.7730460975279,5.91473898239949));
#19937=CARTESIAN_POINT('Ctrl Pts',(14.7061840816217,-11.9452345625921,6.08697056167794));
#19938=CARTESIAN_POINT('Ctrl Pts',(14.9602727846237,-12.1171968581026,6.25906787671289));
#19939=CARTESIAN_POINT('Ctrl Pts',(15.2141544107024,-12.2885930517893,6.43060890607568));
#19940=CARTESIAN_POINT('Ctrl Pts',(15.4096640347472,-12.4205821441389,6.562709533746));
#19941=CARTESIAN_POINT('Ctrl Pts',(15.6050508567913,-12.5522361783519,6.69448102850619));
#19942=CARTESIAN_POINT('Ctrl Pts',(15.8,-12.6834121741351,6.82574786431122));
#19943=CARTESIAN_POINT('Origin',(15.8,0.,0.));
#19944=CARTESIAN_POINT('',(15.8,-14.1719138864591,2.57228207647107));
#19945=CARTESIAN_POINT('Ctrl Pts',(10.0502525316942,-9.16181196696065,0.0459743785884369));
#19946=CARTESIAN_POINT('Ctrl Pts',(10.2643268766627,-9.35649035475233,0.14097883681218));
#19947=CARTESIAN_POINT('Ctrl Pts',(10.4809510016051,-9.55213450057367,0.237133935918737));
#19948=CARTESIAN_POINT('Ctrl Pts',(10.699142806453,-9.74793311715139,0.333938024044436));
#19949=CARTESIAN_POINT('Ctrl Pts',(10.8995862170302,-9.92780487044902,0.422867769115622));
#19950=CARTESIAN_POINT('Ctrl Pts',(11.1013526405404,-10.1078068504778,0.512344667508452));
#19951=CARTESIAN_POINT('Ctrl Pts',(11.3036806718714,-10.2873541596186,0.601985074146008));
#19952=CARTESIAN_POINT('Ctrl Pts',(11.5001990829621,-10.4617459711528,0.68905155804369));
#19953=CARTESIAN_POINT('Ctrl Pts',(11.6972473130466,-10.6357086581841,0.776271799835705));
#19954=CARTESIAN_POINT('Ctrl Pts',(11.8941276803907,-10.8087523681159,0.863306965607153));
#19955=CARTESIAN_POINT('Ctrl Pts',(12.0857598163563,-10.9771832594078,0.948022038754891));
#19956=CARTESIAN_POINT('Ctrl Pts',(12.2772329197189,-11.1447435310821,1.03256139616025));
#19957=CARTESIAN_POINT('Ctrl Pts',(12.4679036288707,-11.3110269536991,1.11663114425723));
#19958=CARTESIAN_POINT('Ctrl Pts',(12.6135402560745,-11.4380362722126,1.18084464940015));
#19959=CARTESIAN_POINT('Ctrl Pts',(12.7587087591265,-11.564301588092,1.24478452215382));
#19960=CARTESIAN_POINT('Ctrl Pts',(12.9031224463839,-11.6896601572689,1.30832923723674));
#19961=CARTESIAN_POINT('Ctrl Pts',(13.1606449942899,-11.9132030828002,1.42164395999532));
#19962=CARTESIAN_POINT('Ctrl Pts',(13.4202017454155,-12.1376081682871,1.53563343890945));
#19963=CARTESIAN_POINT('Ctrl Pts',(13.6810273936588,-12.362278873202,1.64991426889729));
#19964=CARTESIAN_POINT('Ctrl Pts',(13.9372271276793,-12.5829648955663,1.76216825328774));
#19965=CARTESIAN_POINT('Ctrl Pts',(14.1946511485056,-12.8039071645277,1.8747029859119));
#19966=CARTESIAN_POINT('Ctrl Pts',(14.4525741517354,-13.0245839618751,1.98717820849432));
#19967=CARTESIAN_POINT('Ctrl Pts',(14.70618197914,-13.2415687303257,2.09777166653716));
#19968=CARTESIAN_POINT('Ctrl Pts',(14.9602722321869,-13.4582969085292,2.20830732433861));
#19969=CARTESIAN_POINT('Ctrl Pts',(15.2141554048868,-13.6743147818063,2.31848885998681));
#19970=CARTESIAN_POINT('Ctrl Pts',(15.4096646971205,-13.8406649225624,2.40333699632732));
#19971=CARTESIAN_POINT('Ctrl Pts',(15.6050511872361,-14.006594698048,2.48797565175852));
#19972=CARTESIAN_POINT('Ctrl Pts',(15.8,-14.1719138864591,2.57228207647107));
#19973=CARTESIAN_POINT('Origin',(15.8,0.,0.));
#19974=CARTESIAN_POINT('Ctrl Pts',(10.0502525316942,9.36936257048691,-5.29266352931554));
#19975=CARTESIAN_POINT('Ctrl Pts',(11.9668350211294,10.5998888833726,-7.11242577089739));
#19976=CARTESIAN_POINT('Ctrl Pts',(13.8834175105647,11.8304151962582,-8.93218801247923));
#19977=CARTESIAN_POINT('Ctrl Pts',(15.8,13.0609415091439,-10.7519502540611));
#19978=CARTESIAN_POINT('Ctrl Pts',(10.0502525316942,9.19066745032221,-5.50090730964532));
#19979=CARTESIAN_POINT('Ctrl Pts',(11.9668350211294,10.3756997001811,-7.33966268788185));
#19980=CARTESIAN_POINT('Ctrl Pts',(13.8834175105647,11.5602999829831,-9.17890569898124));
#19981=CARTESIAN_POINT('Ctrl Pts',(15.8,12.745332232842,-11.0176610772178));
#19982=CARTESIAN_POINT('Ctrl Pts',(10.0502525316942,8.88494866314842,-5.78937538435654));
#19983=CARTESIAN_POINT('Ctrl Pts',(11.9668350211294,9.99448540715111,-7.65168842520524));
#19984=CARTESIAN_POINT('Ctrl Pts',(13.8834175105647,11.104545703274,-9.51341402508185));
#19985=CARTESIAN_POINT('Ctrl Pts',(15.8,12.2140824472767,-11.3757270659305));
#19986=CARTESIAN_POINT('Ctrl Pts',(10.0502525316942,8.62956238511758,-5.83613263565859));
#19987=CARTESIAN_POINT('Ctrl Pts',(11.9668350211294,9.68562073924798,-7.68881403767578));
#19988=CARTESIAN_POINT('Ctrl Pts',(13.8834175105647,10.7414245752752,-9.54180236671467));
#19989=CARTESIAN_POINT('Ctrl Pts',(15.8,11.7974829294057,-11.3944837687319));
#19990=CARTESIAN_POINT('Ctrl Pts',(10.0502525316942,8.45485763321061,-5.80103525788047));
#19991=CARTESIAN_POINT('Ctrl Pts',(11.9668350211294,9.47972276943763,-7.63326974588331));
#19992=CARTESIAN_POINT('Ctrl Pts',(13.8834175105647,10.5043553237743,-9.46570011434023));
#19993=CARTESIAN_POINT('Ctrl Pts',(15.8,11.5292204600013,-11.2979346023431));
#19994=CARTESIAN_POINT('Ctrl Pts',(10.0502525316941,8.27718317134364,-5.77456941285603));
#19995=CARTESIAN_POINT('Ctrl Pts',(11.9668350211294,9.27115170336996,-7.58519358293628));
#19996=CARTESIAN_POINT('Ctrl Pts',(13.8834175105647,10.2649338319875,-9.39609248134292));
#19997=CARTESIAN_POINT('Ctrl Pts',(15.8,11.2589023640139,-11.2067166514232));
#19998=CARTESIAN_POINT('Ctrl Pts',(10.0502525316942,8.0031076613001,-5.75553891274797));
#19999=CARTESIAN_POINT('Ctrl Pts',(11.9668350211295,8.94781145509674,-7.53737545292391));
#20000=CARTESIAN_POINT('Ctrl Pts',(13.8834175105647,9.89241088219743,-9.31923862861202));
#20001=CARTESIAN_POINT('Ctrl Pts',(15.8,10.8371146759941,-11.101075168788));
#20002=CARTESIAN_POINT('Ctrl Pts',(10.0502525316942,7.76245969237558,-5.66702291215723));
#20003=CARTESIAN_POINT('Ctrl Pts',(11.9668350211294,8.66825218904355,-7.4114007810768));
#20004=CARTESIAN_POINT('Ctrl Pts',(13.8834175105647,9.57397375447812,-9.15584481177961));
#20005=CARTESIAN_POINT('Ctrl Pts',(15.8,10.4797662511461,-10.9002226806992));
#20006=CARTESIAN_POINT('Ctrl Pts',(10.0502525316942,7.54398815168985,-5.55269814935976));
#20007=CARTESIAN_POINT('Ctrl Pts',(11.9668350211294,8.41867077420535,-7.25492061800101));
#20008=CARTESIAN_POINT('Ctrl Pts',(13.8834175105647,9.29328875951754,-8.95722517253277));
#20009=CARTESIAN_POINT('Ctrl Pts',(15.8,10.167971382033,-10.659447641174));
#20010=CARTESIAN_POINT('Ctrl Pts',(10.0502525316942,7.44587907063767,-5.47835809159451));
#20011=CARTESIAN_POINT('Ctrl Pts',(11.9668350211294,8.30851053998513,-7.15753678028296));
#20012=CARTESIAN_POINT('Ctrl Pts',(13.8834175105647,9.17110734047641,-8.83668456248994));
#20013=CARTESIAN_POINT('Ctrl Pts',(15.8,10.0337388098239,-10.5158632511784));
#20014=CARTESIAN_POINT('Ctrl Pts',(10.0502525316942,7.38503851882133,-5.42237201204004));
#20015=CARTESIAN_POINT('Ctrl Pts',(11.9668350211294,8.24114891510682,-7.08526863916361));
#20016=CARTESIAN_POINT('Ctrl Pts',(13.8834175105647,9.09725931139231,-8.74816526628719));
#20017=CARTESIAN_POINT('Ctrl Pts',(15.8,9.95336970767779,-10.4110618934108));
#20018=CARTESIAN_POINT('Ctrl Pts',(15.8,9.9801646912522,-10.4452137610133));
#20019=CARTESIAN_POINT('Ctrl Pts',(15.8,9.97473811086981,-10.4384530463692));
#20020=CARTESIAN_POINT('Ctrl Pts',(15.8,9.96934533045351,-10.4316574943231));
#20021=CARTESIAN_POINT('Ctrl Pts',(15.8,9.96398633981914,-10.4248271146823));
#20022=CARTESIAN_POINT('Ctrl Pts',(15.8,9.95866113228077,-10.4179619142908));
#20023=CARTESIAN_POINT('Ctrl Pts',(15.8,9.95336970767779,-10.4110618934108));
#20024=CARTESIAN_POINT('Origin',(15.8,11.3437865591856,-9.90493637355978));
#20025=CARTESIAN_POINT('Ctrl Pts',(10.0502525316942,7.27527035012649,-7.92891439885425));
#20026=CARTESIAN_POINT('Ctrl Pts',(11.9668350211294,7.88323296009842,-10.0398646795257));
#20027=CARTESIAN_POINT('Ctrl Pts',(13.8834175105647,8.49119557007034,-12.1508149601973));
#20028=CARTESIAN_POINT('Ctrl Pts',(15.8,9.09915818004226,-14.2617652408688));
#20029=CARTESIAN_POINT('Ctrl Pts',(10.0502525316942,7.04097032456894,-8.07174617417206));
#20030=CARTESIAN_POINT('Ctrl Pts',(11.9668350211294,7.59972129962697,-10.186749261509));
#20031=CARTESIAN_POINT('Ctrl Pts',(13.8834175105647,8.15813578620935,-12.3019395333854));
#20032=CARTESIAN_POINT('Ctrl Pts',(15.8,8.71688676126738,-14.4169426207224));
#20033=CARTESIAN_POINT('Ctrl Pts',(10.0502525316942,6.66138127597021,-8.25126590443755));
#20034=CARTESIAN_POINT('Ctrl Pts',(11.9668350211294,7.14127838379809,-10.365200404417));
#20035=CARTESIAN_POINT('Ctrl Pts',(13.8834175105647,7.62165928459737,-12.4788866778492));
#20036=CARTESIAN_POINT('Ctrl Pts',(15.8,8.10155639242524,-14.5928211778287));
#20037=CARTESIAN_POINT('Ctrl Pts',(10.0502525316942,6.42930419296208,-8.22079862024226));
#20038=CARTESIAN_POINT('Ctrl Pts',(11.9668350211294,6.86580395314969,-10.3118069242151));
#20039=CARTESIAN_POINT('Ctrl Pts',(13.8834175105647,7.30234839548018,-12.4027801127282));
#20040=CARTESIAN_POINT('Ctrl Pts',(15.8,7.73884815566778,-14.493788416701));
#20041=CARTESIAN_POINT('Ctrl Pts',(10.0502525316942,6.30697938690418,-8.16221173215364));
#20042=CARTESIAN_POINT('Ctrl Pts',(11.9668350211294,6.72434771418859,-10.2323186327506));
#20043=CARTESIAN_POINT('Ctrl Pts',(13.8834175105647,7.14137150628508,-12.3026176380752));
#20044=CARTESIAN_POINT('Ctrl Pts',(15.8,7.55873983356949,-14.3727245386721));
#20045=CARTESIAN_POINT('Ctrl Pts',(10.0502525316942,6.22815403351084,-8.12000643506485));
#20046=CARTESIAN_POINT('Ctrl Pts',(11.9668350211294,6.63375833246635,-10.1755454476056));
#20047=CARTESIAN_POINT('Ctrl Pts',(13.8834175105647,7.03916552489902,-12.2311493413123));
#20048=CARTESIAN_POINT('Ctrl Pts',(15.8,7.44476982385453,-14.2866883538531));
#20049=CARTESIAN_POINT('Ctrl Pts',(10.0502525316942,6.08789997184504,-8.04942040067478));
#20050=CARTESIAN_POINT('Ctrl Pts',(11.9668350211294,6.47376321403758,-10.0785454407991));
#20051=CARTESIAN_POINT('Ctrl Pts',(13.8834175105647,6.85942462405721,-12.1078515605739));
#20052=CARTESIAN_POINT('Ctrl Pts',(15.8,7.24528786624975,-14.1369766006982));
#20053=CARTESIAN_POINT('Ctrl Pts',(10.0502525316942,5.83267830770084,-7.94713925110582));
#20054=CARTESIAN_POINT('Ctrl Pts',(11.9668350211294,6.18048893841472,-9.93371906448111));
#20055=CARTESIAN_POINT('Ctrl Pts',(13.8834175105647,6.52817426230452,-11.920292369998));
#20056=CARTESIAN_POINT('Ctrl Pts',(15.8,6.8759848930184,-13.9068721833733));
#20057=CARTESIAN_POINT('Ctrl Pts',(10.0502525316942,5.63138575926581,-7.78832910259187));
#20058=CARTESIAN_POINT('Ctrl Pts',(11.9668350211294,5.95382183425817,-9.7272251121909));
#20059=CARTESIAN_POINT('Ctrl Pts',(13.8834175105647,6.27616146093386,-11.6661698490829));
#20060=CARTESIAN_POINT('Ctrl Pts',(15.8,6.59859753592622,-13.605065858682));
#20061=CARTESIAN_POINT('Ctrl Pts',(10.0502525316942,5.45884429554415,-7.61219406851115));
#20062=CARTESIAN_POINT('Ctrl Pts',(11.9668350211294,5.7646862128331,-9.50140467053762));
#20063=CARTESIAN_POINT('Ctrl Pts',(13.8834175105647,6.07045912241827,-11.3906602079427));
#20064=CARTESIAN_POINT('Ctrl Pts',(15.8,6.37630103970722,-13.2798708099692));
#20065=CARTESIAN_POINT('Ctrl Pts',(10.0502525316942,5.38854605810145,-7.51113133249701));
#20066=CARTESIAN_POINT('Ctrl Pts',(11.9668350211294,5.69007333772413,-9.37468648227302));
#20067=CARTESIAN_POINT('Ctrl Pts',(13.8834175105647,5.99154494312677,-11.238220929081));
#20068=CARTESIAN_POINT('Ctrl Pts',(15.8,6.29307222274945,-13.101776078857));
#20069=CARTESIAN_POINT('Ctrl Pts',(10.0502525316942,5.34798390487229,-7.43908464225652));
#20070=CARTESIAN_POINT('Ctrl Pts',(11.9668350211294,5.64832995825766,-9.28514597692092));
#20071=CARTESIAN_POINT('Ctrl Pts',(13.8834175105647,5.94867601164304,-11.1312073115853));
#20072=CARTESIAN_POINT('Ctrl Pts',(15.8,6.24902206502841,-12.9772686462497));
#20073=CARTESIAN_POINT('Ctrl Pts',(15.8,6.26395210128206,-13.0180291077652));
#20074=CARTESIAN_POINT('Ctrl Pts',(15.8,6.26088029236732,-13.0099223804886));
#20075=CARTESIAN_POINT('Ctrl Pts',(15.8,6.25785139447984,-13.0017929656379));
#20076=CARTESIAN_POINT('Ctrl Pts',(15.8,6.2548653949033,-12.993640869393));
#20077=CARTESIAN_POINT('Ctrl Pts',(15.8,6.25192228516408,-12.985466096197));
#20078=CARTESIAN_POINT('Ctrl Pts',(15.8,6.24902206502841,-12.9772686462497));
#20079=CARTESIAN_POINT('Origin',(15.8,7.7277884589423,-12.9255771089134));
#20080=CARTESIAN_POINT('Ctrl Pts',(10.0502525316942,4.46902397810654,-9.78902788303806));
#20081=CARTESIAN_POINT('Ctrl Pts',(11.9668350211294,4.39491126897609,-11.9845316814717));
#20082=CARTESIAN_POINT('Ctrl Pts',(13.8834175105647,4.32079855984563,-14.1800354799052));
#20083=CARTESIAN_POINT('Ctrl Pts',(15.8,4.24668585071518,-16.3755392783388));
#20084=CARTESIAN_POINT('Ctrl Pts',(10.0502525316942,4.20205396612197,-9.8524662840083));
#20085=CARTESIAN_POINT('Ctrl Pts',(11.9668350211294,4.07988582479457,-12.036617299121));
#20086=CARTESIAN_POINT('Ctrl Pts',(13.8834175105647,3.95733982070598,-14.2208423566523));
#20087=CARTESIAN_POINT('Ctrl Pts',(15.8,3.83517167937858,-16.404993371765));
#20088=CARTESIAN_POINT('Ctrl Pts',(10.0502525316942,3.7855656109216,-9.90590216992165));
#20089=CARTESIAN_POINT('Ctrl Pts',(11.9668350211295,3.58873319698334,-12.0646697130184));
#20090=CARTESIAN_POINT('Ctrl Pts',(13.8834175105647,3.39243568541408,-14.2233509855394));
#20091=CARTESIAN_POINT('Ctrl Pts',(15.8,3.19560327147581,-16.3821185286362));
#20092=CARTESIAN_POINT('Ctrl Pts',(10.0502525316942,3.57425782911966,-9.80521299123422));
#20093=CARTESIAN_POINT('Ctrl Pts',(11.9668350211295,3.34323666910061,-11.9287659082934));
#20094=CARTESIAN_POINT('Ctrl Pts',(13.8834175105647,3.11226431322855,-14.0522999619539));
#20095=CARTESIAN_POINT('Ctrl Pts',(15.8,2.8812431532095,-16.1758528790132));
#20096=CARTESIAN_POINT('Ctrl Pts',(10.0502525316942,3.47602249721152,-9.71169428155716));
#20097=CARTESIAN_POINT('Ctrl Pts',(11.9668350211295,3.23326515211326,-11.8094568448422));
#20098=CARTESIAN_POINT('Ctrl Pts',(13.8834175105647,2.99011502771357,-13.9072965714997));
#20099=CARTESIAN_POINT('Ctrl Pts',(15.8,2.74735768261531,-16.0050591347847));
#20100=CARTESIAN_POINT('Ctrl Pts',(10.0502525316942,3.414097226746,-9.64719632995103));
#20101=CARTESIAN_POINT('Ctrl Pts',(11.9668350211295,3.16465335082917,-11.7274687236956));
#20102=CARTESIAN_POINT('Ctrl Pts',(13.8834175105647,2.91499625447087,-13.8077428217682));
#20103=CARTESIAN_POINT('Ctrl Pts',(15.8,2.66555237855405,-15.8880152155128));
#20104=CARTESIAN_POINT('Ctrl Pts',(10.0502525316942,3.30251999207182,-9.53672408685997));
#20105=CARTESIAN_POINT('Ctrl Pts',(11.9668350211294,3.04246362184766,-11.5857749779899));
#20106=CARTESIAN_POINT('Ctrl Pts',(13.8834175105647,2.78215337892879,-13.6349367240444));
#20107=CARTESIAN_POINT('Ctrl Pts',(15.8,2.52209700870463,-15.6839876151744));
#20108=CARTESIAN_POINT('Ctrl Pts',(10.0502525316942,3.09139659750779,-9.36058107581316));
#20109=CARTESIAN_POINT('Ctrl Pts',(11.9668350211295,2.80829724126977,-11.357410148179));
#20110=CARTESIAN_POINT('Ctrl Pts',(13.8834175105647,2.52507603204706,-13.3541948572957));
#20111=CARTESIAN_POINT('Ctrl Pts',(15.8,2.24197667580905,-15.3510239296616));
#20112=CARTESIAN_POINT('Ctrl Pts',(10.0502525316942,2.94903314862294,-9.14733948977135));
#20113=CARTESIAN_POINT('Ctrl Pts',(11.9668350211294,2.65653626154119,-11.0909774008914));
#20114=CARTESIAN_POINT('Ctrl Pts',(13.8834175105647,2.36392896441619,-13.0346322911662));
#20115=CARTESIAN_POINT('Ctrl Pts',(15.8,2.07143207733444,-14.9782702022863));
#20116=CARTESIAN_POINT('Ctrl Pts',(10.0502525316942,2.83936642791008,-8.92650608260145));
#20117=CARTESIAN_POINT('Ctrl Pts',(11.9668350211294,2.54644119432443,-10.8177624863471));
#20118=CARTESIAN_POINT('Ctrl Pts',(13.8834175105648,2.2534334908895,-12.7090406610097));
#20119=CARTESIAN_POINT('Ctrl Pts',(15.8,1.96050825730386,-14.6002970647553));
#20120=CARTESIAN_POINT('Ctrl Pts',(10.0502525316942,2.80374461319022,-8.80866270544546));
#20121=CARTESIAN_POINT('Ctrl Pts',(11.9668350211294,2.51464388608039,-10.6741860277864));
#20122=CARTESIAN_POINT('Ctrl Pts',(13.8834175105647,2.22549660720977,-12.5396724561545));
#20123=CARTESIAN_POINT('Ctrl Pts',(15.8,1.93639588009993,-14.4051957784954));
#20124=CARTESIAN_POINT('Ctrl Pts',(10.0502525316942,2.78743136471945,-8.7276078365385));
#20125=CARTESIAN_POINT('Ctrl Pts',(11.9668350211294,2.50261311086535,-10.5761285330411));
#20126=CARTESIAN_POINT('Ctrl Pts',(13.8834175105647,2.21779485701124,-12.4246492295437));
#20127=CARTESIAN_POINT('Ctrl Pts',(15.8,1.93297660315714,-14.2731699260464));
#20128=CARTESIAN_POINT('Ctrl Pts',(15.8,1.93458023611785,-14.3165490635069));
#20129=CARTESIAN_POINT('Ctrl Pts',(15.8,1.93416388872989,-14.3078898665466));
#20130=CARTESIAN_POINT('Ctrl Pts',(15.8,1.93379536300002,-14.2992223526576));
#20131=CARTESIAN_POINT('Ctrl Pts',(15.8,1.93347464492456,-14.2905465237881));
#20132=CARTESIAN_POINT('Ctrl Pts',(15.8,1.93320172507161,-14.2818623815451));
#20133=CARTESIAN_POINT('Ctrl Pts',(15.8,1.93297660315714,-14.2731699260464));
#20134=CARTESIAN_POINT('Origin',(15.8,3.35534058166952,-14.6809722990553));
#20135=CARTESIAN_POINT('Ctrl Pts',(10.0502525316942,1.22531840158854,-10.6909231138624));
#20136=CARTESIAN_POINT('Ctrl Pts',(11.9668350211294,0.476385041699009,-12.7560692212929));
#20137=CARTESIAN_POINT('Ctrl Pts',(13.8834175105647,-0.272548318190526,
-14.8212153287235));
#20138=CARTESIAN_POINT('Ctrl Pts',(15.8,-1.02148167808006,-16.886361436154));
#20139=CARTESIAN_POINT('Ctrl Pts',(10.0502525316942,0.951811288039437,-10.6687583477967));
#20140=CARTESIAN_POINT('Ctrl Pts',(11.9668350211294,0.160771418505766,-12.7082628707158));
#20141=CARTESIAN_POINT('Ctrl Pts',(13.8834175105647,-0.630916858166454,
-14.7477045483503));
#20142=CARTESIAN_POINT('Ctrl Pts',(15.8,-1.42195672770012,-16.7872090712694));
#20143=CARTESIAN_POINT('Ctrl Pts',(10.0502525316942,0.53873797019293,-10.5909841198542));
#20144=CARTESIAN_POINT('Ctrl Pts',(11.9668350211294,-0.315735593698357,
-12.5832583421986));
#20145=CARTESIAN_POINT('Ctrl Pts',(13.8834175105647,-1.16942659814004,-14.5756107736058));
#20146=CARTESIAN_POINT('Ctrl Pts',(15.8,-2.02390016203133,-16.5678849959503));
#20147=CARTESIAN_POINT('Ctrl Pts',(10.0502525316942,0.350797420983484,-10.4118557126012));
#20148=CARTESIAN_POINT('Ctrl Pts',(11.9668350211294,-0.527317792292718,
-12.3552036734465));
#20149=CARTESIAN_POINT('Ctrl Pts',(13.8834175105647,-1.40583184426592,-14.2985259967778));
#20150=CARTESIAN_POINT('Ctrl Pts',(15.8,-2.28394705754213,-16.2418739576232));
#20151=CARTESIAN_POINT('Ctrl Pts',(10.0502525316942,0.276502431596342,-10.2498870013208));
#20152=CARTESIAN_POINT('Ctrl Pts',(11.9668350211294,-0.603405794214882,
-12.1559807242605));
#20153=CARTESIAN_POINT('Ctrl Pts',(13.8834175105647,-1.48361038150706,-14.0620012424206));
#20154=CARTESIAN_POINT('Ctrl Pts',(15.8,-2.36351860731828,-15.9680949653604));
#20155=CARTESIAN_POINT('Ctrl Pts',(10.0502525316942,0.193479460458701,-10.0905890686414));
#20156=CARTESIAN_POINT('Ctrl Pts',(11.9668350211294,-0.687106219194378,
-11.9589846875421));
#20157=CARTESIAN_POINT('Ctrl Pts',(13.8834175105647,-1.56802487912709,-13.8273908205778));
#20158=CARTESIAN_POINT('Ctrl Pts',(15.8,-2.44861055878017,-15.6957864394785));
#20159=CARTESIAN_POINT('Ctrl Pts',(10.0502525316942,0.0477779613143522,
-9.85767148446325));
#20160=CARTESIAN_POINT('Ctrl Pts',(11.9668350211294,-0.83847512310783,-11.6692901486065));
#20161=CARTESIAN_POINT('Ctrl Pts',(13.8834175105647,-1.72481200902093,-13.4808398643785));
#20162=CARTESIAN_POINT('Ctrl Pts',(15.8,-2.61106509344311,-15.2924585285217));
#20163=CARTESIAN_POINT('Ctrl Pts',(10.0502525316942,-0.0220599042734183,
-9.6109546595346));
#20164=CARTESIAN_POINT('Ctrl Pts',(11.9668350211294,-0.900879773662289,
-11.3690757684926));
#20165=CARTESIAN_POINT('Ctrl Pts',(13.8834175105647,-1.77979551853007,-13.1271782591657));
#20166=CARTESIAN_POINT('Ctrl Pts',(15.8,-2.65861538791894,-14.8852993681237));
#20167=CARTESIAN_POINT('Ctrl Pts',(10.0502525316942,-0.0579833517275581,
-9.36700900338232));
#20168=CARTESIAN_POINT('Ctrl Pts',(11.9668350211294,-0.920984711114089,
-11.07518337287));
#20169=CARTESIAN_POINT('Ctrl Pts',(13.8834175105647,-1.78409102238058,-12.7833535968728));
#20170=CARTESIAN_POINT('Ctrl Pts',(15.8,-2.64709238176712,-14.4915279663605));
#20171=CARTESIAN_POINT('Ctrl Pts',(10.0502525316942,-0.0555068892974584,
-9.243940799223));
#20172=CARTESIAN_POINT('Ctrl Pts',(11.9668350211294,-0.906948929192826,
-10.9288207869826));
#20173=CARTESIAN_POINT('Ctrl Pts',(13.8834175105647,-1.75838634306183,-12.6136545606744));
#20174=CARTESIAN_POINT('Ctrl Pts',(15.8,-2.6098283829572,-14.298534548434));
#20175=CARTESIAN_POINT('Ctrl Pts',(10.0502525316942,-0.0459743785884374,
-9.16181196696065));
#20176=CARTESIAN_POINT('Ctrl Pts',(11.9668350211294,-0.888076944549316,
-10.8318459401268));
#20177=CARTESIAN_POINT('Ctrl Pts',(13.8834175105647,-1.73017951051019,-12.501879913293));
#20178=CARTESIAN_POINT('Ctrl Pts',(15.8,-2.57228207647107,-14.1719138864591));
#20179=CARTESIAN_POINT('Ctrl Pts',(15.8,-2.58416182157067,-14.2136654476498));
#20180=CARTESIAN_POINT('Ctrl Pts',(15.8,-2.58188195244865,-14.2053014035364));
#20181=CARTESIAN_POINT('Ctrl Pts',(15.8,-2.57955403215479,-14.1969442272588));
#20182=CARTESIAN_POINT('Ctrl Pts',(15.8,-2.57717807460939,-14.1885939163425));
#20183=CARTESIAN_POINT('Ctrl Pts',(15.8,-2.57475408927931,-14.1802504694012));
#20184=CARTESIAN_POINT('Ctrl Pts',(15.8,-2.57228207647107,-14.1719138864591));
#20185=CARTESIAN_POINT('Origin',(15.8,-1.34555140976956,-14.999291632217));
#20186=CARTESIAN_POINT('Ctrl Pts',(10.0502525316942,-2.13832987737225,-10.5463163022605));
#20187=CARTESIAN_POINT('Ctrl Pts',(11.9668350211294,-3.48877307262933,-12.2789538289737));
#20188=CARTESIAN_POINT('Ctrl Pts',(13.8834175105647,-4.8392162678864,-14.0115913556869));
#20189=CARTESIAN_POINT('Ctrl Pts',(15.8,-6.18965946314348,-15.7442288824001));
#20190=CARTESIAN_POINT('Ctrl Pts',(10.0502525316942,-2.39160131057558,-10.4407180108925));
#20191=CARTESIAN_POINT('Ctrl Pts',(11.9668350211294,-3.77416649083142,-12.1359573145141));
#20192=CARTESIAN_POINT('Ctrl Pts',(13.8834175105647,-5.15732892266062,-13.8309364798931));
#20193=CARTESIAN_POINT('Ctrl Pts',(15.8,-6.53989410291645,-15.5261757835147));
#20194=CARTESIAN_POINT('Ctrl Pts',(10.0502525316942,-2.7604211119455,-10.2391038402362));
#20195=CARTESIAN_POINT('Ctrl Pts',(11.9668350211294,-4.18872035504581,-11.8698223691572));
#20196=CARTESIAN_POINT('Ctrl Pts',(13.8834175105647,-5.61629814839675,-13.5008577836237));
#20197=CARTESIAN_POINT('Ctrl Pts',(15.8,-7.04459739149706,-15.1315763125447));
#20198=CARTESIAN_POINT('Ctrl Pts',(10.0502525316942,-2.88380634898391,-10.0106660065973));
#20199=CARTESIAN_POINT('Ctrl Pts',(11.9668350211294,-4.31947109051326,-11.5875472242667));
#20200=CARTESIAN_POINT('Ctrl Pts',(13.8834175105647,-5.75550424110768,-13.1642822866715));
#20201=CARTESIAN_POINT('Ctrl Pts',(15.8,-7.19116898263704,-14.7411635043409));
#20202=CARTESIAN_POINT('Ctrl Pts',(10.0502525316942,-2.90441220847246,-9.83366631411429));
#20203=CARTESIAN_POINT('Ctrl Pts',(11.9668350211294,-4.33027001363173,-11.3745625747195));
#20204=CARTESIAN_POINT('Ctrl Pts',(13.8834175105647,-5.75638324902558,-12.9152995332973));
#20205=CARTESIAN_POINT('Ctrl Pts',(15.8,-7.18224105418486,-14.4561957939025));
#20206=CARTESIAN_POINT('Ctrl Pts',(10.0502525316941,-2.93414649567711,-9.65650945139357));
#20207=CARTESIAN_POINT('Ctrl Pts',(11.9668350211294,-4.34899924292338,-11.1613433397504));
#20208=CARTESIAN_POINT('Ctrl Pts',(13.8834175105647,-5.76416819477548,-12.6660861533134));
#20209=CARTESIAN_POINT('Ctrl Pts',(15.8,-7.17902094202174,-14.1709200416702));
#20210=CARTESIAN_POINT('Ctrl Pts',(10.0502525316942,-3.00074150798573,-9.38996734645582));
#20211=CARTESIAN_POINT('Ctrl Pts',(11.9668350211294,-4.40343923355922,-10.8390518176275));
#20212=CARTESIAN_POINT('Ctrl Pts',(13.8834175105647,-5.80619247524441,-12.2880463890102));
#20213=CARTESIAN_POINT('Ctrl Pts',(15.8,-7.20889020081791,-13.7371308601818));
#20214=CARTESIAN_POINT('Ctrl Pts',(10.0502525316942,-2.99092345166592,-9.13374448664767));
#20215=CARTESIAN_POINT('Ctrl Pts',(11.9668350211294,-4.37002011593521,-10.5342467491227));
#20216=CARTESIAN_POINT('Ctrl Pts',(13.8834175105647,-5.74920012742636,-11.9347028120052));
#20217=CARTESIAN_POINT('Ctrl Pts',(15.8,-7.12829679169565,-13.3352050744803));
#20218=CARTESIAN_POINT('Ctrl Pts',(10.0502525316942,-2.94970615383951,-8.89063737063807));
#20219=CARTESIAN_POINT('Ctrl Pts',(11.9668350211294,-4.29832412978306,-10.2485256494886));
#20220=CARTESIAN_POINT('Ctrl Pts',(13.8834175105647,-5.64703889510256,-11.6063785007713));
#20221=CARTESIAN_POINT('Ctrl Pts',(15.8,-6.99565687104611,-12.9642667796218));
#20222=CARTESIAN_POINT('Ctrl Pts',(10.0502525316942,-2.90932499072146,-8.77435756124985));
#20223=CARTESIAN_POINT('Ctrl Pts',(11.9668350211294,-4.23975104071156,-10.113663592731));
#20224=CARTESIAN_POINT('Ctrl Pts',(13.8834175105647,-5.57015841015682,-11.4529271015425));
#20225=CARTESIAN_POINT('Ctrl Pts',(15.8,-6.90058446014692,-12.7922331330237));
#20226=CARTESIAN_POINT('Ctrl Pts',(10.0502525316942,-2.87487982939776,-8.69919410795919));
#20227=CARTESIAN_POINT('Ctrl Pts',(11.9668350211294,-4.19183584103558,-10.0272667966845));
#20228=CARTESIAN_POINT('Ctrl Pts',(13.8834175105647,-5.5087918526734,-11.3553394854098));
#20229=CARTESIAN_POINT('Ctrl Pts',(15.8,-6.82574786431122,-12.6834121741351));
#20230=CARTESIAN_POINT('Ctrl Pts',(15.8,-6.84994811524973,-12.7194492253464));
#20231=CARTESIAN_POINT('Ctrl Pts',(15.8,-6.84519519909218,-12.7121990649934));
#20232=CARTESIAN_POINT('Ctrl Pts',(15.8,-6.84039870583253,-12.7049702849691));
#20233=CARTESIAN_POINT('Ctrl Pts',(15.8,-6.83555864794507,-12.6977628786185));
#20234=CARTESIAN_POINT('Ctrl Pts',(15.8,-6.83067503400497,-12.6905768416977));
#20235=CARTESIAN_POINT('Ctrl Pts',(15.8,-6.82574786431122,-12.6834121741351));
#20236=CARTESIAN_POINT('Origin',(15.8,-5.91473145421246,-13.8493757942074));
#20237=CARTESIAN_POINT('Ctrl Pts',(10.0502525316942,-5.29266352931554,-9.36936257048691));
#20238=CARTESIAN_POINT('Ctrl Pts',(11.9668350211294,-7.11242577089738,-10.5998888833726));
#20239=CARTESIAN_POINT('Ctrl Pts',(13.8834175105647,-8.93218801247923,-11.8304151962582));
#20240=CARTESIAN_POINT('Ctrl Pts',(15.8,-10.7519502540611,-13.0609415091439));
#20241=CARTESIAN_POINT('Ctrl Pts',(10.0502525316942,-5.50090730964532,-9.19066745032221));
#20242=CARTESIAN_POINT('Ctrl Pts',(11.9668350211294,-7.33966268788185,-10.3756997001811));
#20243=CARTESIAN_POINT('Ctrl Pts',(13.8834175105647,-9.17890569898124,-11.5602999829831));
#20244=CARTESIAN_POINT('Ctrl Pts',(15.8,-11.0176610772178,-12.745332232842));
#20245=CARTESIAN_POINT('Ctrl Pts',(10.0502525316942,-5.78937538435653,-8.88494866314842));
#20246=CARTESIAN_POINT('Ctrl Pts',(11.9668350211294,-7.65168842520523,-9.99448540715111));
#20247=CARTESIAN_POINT('Ctrl Pts',(13.8834175105647,-9.51341402508183,-11.104545703274));
#20248=CARTESIAN_POINT('Ctrl Pts',(15.8,-11.3757270659305,-12.2140824472766));
#20249=CARTESIAN_POINT('Ctrl Pts',(10.0502525316942,-5.83613263565859,-8.62956238511758));
#20250=CARTESIAN_POINT('Ctrl Pts',(11.9668350211294,-7.68881403767578,-9.68562073924798));
#20251=CARTESIAN_POINT('Ctrl Pts',(13.8834175105647,-9.54180236671465,-10.7414245752752));
#20252=CARTESIAN_POINT('Ctrl Pts',(15.8,-11.3944837687318,-11.7974829294056));
#20253=CARTESIAN_POINT('Ctrl Pts',(10.0502525316942,-5.80103525788045,-8.45485763321061));
#20254=CARTESIAN_POINT('Ctrl Pts',(11.9668350211294,-7.6332697458833,-9.47972276943763));
#20255=CARTESIAN_POINT('Ctrl Pts',(13.8834175105647,-9.46570011434025,-10.5043553237743));
#20256=CARTESIAN_POINT('Ctrl Pts',(15.8,-11.2979346023431,-11.5292204600013));
#20257=CARTESIAN_POINT('Ctrl Pts',(10.0502525316941,-5.77456941285602,-8.27718317134364));
#20258=CARTESIAN_POINT('Ctrl Pts',(11.9668350211294,-7.58519358293626,-9.27115170336996));
#20259=CARTESIAN_POINT('Ctrl Pts',(13.8834175105647,-9.39609248134292,-10.2649338319875));
#20260=CARTESIAN_POINT('Ctrl Pts',(15.8,-11.2067166514232,-11.2589023640139));
#20261=CARTESIAN_POINT('Ctrl Pts',(10.0502525316942,-5.75553891274799,-8.0031076613001));
#20262=CARTESIAN_POINT('Ctrl Pts',(11.9668350211295,-7.53737545292393,-8.94781145509674));
#20263=CARTESIAN_POINT('Ctrl Pts',(13.8834175105647,-9.31923862861202,-9.89241088219744));
#20264=CARTESIAN_POINT('Ctrl Pts',(15.8,-11.101075168788,-10.8371146759941));
#20265=CARTESIAN_POINT('Ctrl Pts',(10.0502525316942,-5.66702291215723,-7.76245969237558));
#20266=CARTESIAN_POINT('Ctrl Pts',(11.9668350211294,-7.4114007810768,-8.66825218904355));
#20267=CARTESIAN_POINT('Ctrl Pts',(13.8834175105647,-9.1558448117796,-9.57397375447812));
#20268=CARTESIAN_POINT('Ctrl Pts',(15.8,-10.9002226806992,-10.4797662511461));
#20269=CARTESIAN_POINT('Ctrl Pts',(10.0502525316942,-5.55269814935977,-7.54398815168985));
#20270=CARTESIAN_POINT('Ctrl Pts',(11.9668350211294,-7.25492061800102,-8.41867077420536));
#20271=CARTESIAN_POINT('Ctrl Pts',(13.8834175105647,-8.95722517253276,-9.29328875951756));
#20272=CARTESIAN_POINT('Ctrl Pts',(15.8,-10.659447641174,-10.1679713820331));
#20273=CARTESIAN_POINT('Ctrl Pts',(10.0502525316942,-5.47835809159451,-7.44587907063767));
#20274=CARTESIAN_POINT('Ctrl Pts',(11.9668350211294,-7.15753678028296,-8.30851053998513));
#20275=CARTESIAN_POINT('Ctrl Pts',(13.8834175105647,-8.83668456248994,-9.17110734047641));
#20276=CARTESIAN_POINT('Ctrl Pts',(15.8,-10.5158632511784,-10.0337388098239));
#20277=CARTESIAN_POINT('Ctrl Pts',(10.0502525316942,-5.42237201204004,-7.38503851882133));
#20278=CARTESIAN_POINT('Ctrl Pts',(11.9668350211294,-7.08526863916361,-8.24114891510682));
#20279=CARTESIAN_POINT('Ctrl Pts',(13.8834175105647,-8.74816526628719,-9.09725931139231));
#20280=CARTESIAN_POINT('Ctrl Pts',(15.8,-10.4110618934108,-9.95336970767779));
#20281=CARTESIAN_POINT('Ctrl Pts',(15.8,-10.4452137610133,-9.9801646912522));
#20282=CARTESIAN_POINT('Ctrl Pts',(15.8,-10.4384530463692,-9.97473811086981));
#20283=CARTESIAN_POINT('Ctrl Pts',(15.8,-10.4316574943231,-9.96934533045351));
#20284=CARTESIAN_POINT('Ctrl Pts',(15.8,-10.4248271146823,-9.96398633981914));
#20285=CARTESIAN_POINT('Ctrl Pts',(15.8,-10.4179619142908,-9.95866113228077));
#20286=CARTESIAN_POINT('Ctrl Pts',(15.8,-10.4110618934108,-9.95336970767779));
#20287=CARTESIAN_POINT('Origin',(15.8,-9.90493637355978,-11.3437865591856));
#20288=CARTESIAN_POINT('Ctrl Pts',(10.0502525316942,-7.92891439885425,-7.2752703501265));
#20289=CARTESIAN_POINT('Ctrl Pts',(11.9668350211294,-10.0398646795257,-7.88323296009842));
#20290=CARTESIAN_POINT('Ctrl Pts',(13.8834175105647,-12.1508149601973,-8.49119557007034));
#20291=CARTESIAN_POINT('Ctrl Pts',(15.8,-14.2617652408688,-9.09915818004226));
#20292=CARTESIAN_POINT('Ctrl Pts',(10.0502525316942,-8.07174617417205,-7.04097032456894));
#20293=CARTESIAN_POINT('Ctrl Pts',(11.9668350211294,-10.186749261509,-7.59972129962698));
#20294=CARTESIAN_POINT('Ctrl Pts',(13.8834175105647,-12.3019395333854,-8.15813578620935));
#20295=CARTESIAN_POINT('Ctrl Pts',(15.8,-14.4169426207224,-8.71688676126738));
#20296=CARTESIAN_POINT('Ctrl Pts',(10.0502525316942,-8.25126590443755,-6.66138127597024));
#20297=CARTESIAN_POINT('Ctrl Pts',(11.9668350211294,-10.365200404417,-7.14127838379811));
#20298=CARTESIAN_POINT('Ctrl Pts',(13.8834175105647,-12.4788866778492,-7.62165928459738));
#20299=CARTESIAN_POINT('Ctrl Pts',(15.8,-14.5928211778286,-8.10155639242525));
#20300=CARTESIAN_POINT('Ctrl Pts',(10.0502525316942,-8.22079862024226,-6.42930419296208));
#20301=CARTESIAN_POINT('Ctrl Pts',(11.9668350211294,-10.3118069242151,-6.86580395314969));
#20302=CARTESIAN_POINT('Ctrl Pts',(13.8834175105647,-12.4027801127282,-7.30234839548021));
#20303=CARTESIAN_POINT('Ctrl Pts',(15.8,-14.493788416701,-7.73884815566781));
#20304=CARTESIAN_POINT('Ctrl Pts',(10.0502525316942,-8.16221173215364,-6.30697938690416));
#20305=CARTESIAN_POINT('Ctrl Pts',(11.9668350211294,-10.2323186327506,-6.72434771418858));
#20306=CARTESIAN_POINT('Ctrl Pts',(13.8834175105647,-12.3026176380752,-7.1413715062851));
#20307=CARTESIAN_POINT('Ctrl Pts',(15.8,-14.3727245386721,-7.55873983356951));
#20308=CARTESIAN_POINT('Ctrl Pts',(10.0502525316942,-8.12000643506485,-6.22815403351084));
#20309=CARTESIAN_POINT('Ctrl Pts',(11.9668350211294,-10.1755454476056,-6.63375833246636));
#20310=CARTESIAN_POINT('Ctrl Pts',(13.8834175105647,-12.2311493413123,-7.03916552489902));
#20311=CARTESIAN_POINT('Ctrl Pts',(15.8,-14.2866883538531,-7.44476982385454));
#20312=CARTESIAN_POINT('Ctrl Pts',(10.0502525316942,-8.04942040067478,-6.08789997184504));
#20313=CARTESIAN_POINT('Ctrl Pts',(11.9668350211294,-10.0785454407991,-6.47376321403759));
#20314=CARTESIAN_POINT('Ctrl Pts',(13.8834175105647,-12.1078515605739,-6.85942462405723));
#20315=CARTESIAN_POINT('Ctrl Pts',(15.8,-14.1369766006982,-7.24528786624978));
#20316=CARTESIAN_POINT('Ctrl Pts',(10.0502525316942,-7.94713925110583,-5.83267830770086));
#20317=CARTESIAN_POINT('Ctrl Pts',(11.9668350211294,-9.93371906448112,-6.18048893841474));
#20318=CARTESIAN_POINT('Ctrl Pts',(13.8834175105647,-11.920292369998,-6.52817426230451));
#20319=CARTESIAN_POINT('Ctrl Pts',(15.8,-13.9068721833733,-6.87598489301839));
#20320=CARTESIAN_POINT('Ctrl Pts',(10.0502525316942,-7.78832910259187,-5.63138575926579));
#20321=CARTESIAN_POINT('Ctrl Pts',(11.9668350211294,-9.7272251121909,-5.95382183425815));
#20322=CARTESIAN_POINT('Ctrl Pts',(13.8834175105647,-11.6661698490829,-6.27616146093385));
#20323=CARTESIAN_POINT('Ctrl Pts',(15.8,-13.605065858682,-6.59859753592622));
#20324=CARTESIAN_POINT('Ctrl Pts',(10.0502525316942,-7.61219406851115,-5.45884429554414));
#20325=CARTESIAN_POINT('Ctrl Pts',(11.9668350211294,-9.50140467053763,-5.76468621283309));
#20326=CARTESIAN_POINT('Ctrl Pts',(13.8834175105648,-11.3906602079427,-6.07045912241827));
#20327=CARTESIAN_POINT('Ctrl Pts',(15.8,-13.2798708099692,-6.37630103970722));
#20328=CARTESIAN_POINT('Ctrl Pts',(10.0502525316942,-7.51113133249701,-5.38854605810145));
#20329=CARTESIAN_POINT('Ctrl Pts',(11.9668350211294,-9.37468648227302,-5.69007333772413));
#20330=CARTESIAN_POINT('Ctrl Pts',(13.8834175105647,-11.238220929081,-5.99154494312677));
#20331=CARTESIAN_POINT('Ctrl Pts',(15.8,-13.101776078857,-6.29307222274945));
#20332=CARTESIAN_POINT('Ctrl Pts',(10.0502525316942,-7.43908464225652,-5.34798390487229));
#20333=CARTESIAN_POINT('Ctrl Pts',(11.9668350211294,-9.28514597692092,-5.64832995825767));
#20334=CARTESIAN_POINT('Ctrl Pts',(13.8834175105647,-11.1312073115853,-5.94867601164304));
#20335=CARTESIAN_POINT('Ctrl Pts',(15.8,-12.9772686462497,-6.24902206502841));
#20336=CARTESIAN_POINT('Ctrl Pts',(15.8,-13.0180291077652,-6.26395210128206));
#20337=CARTESIAN_POINT('Ctrl Pts',(15.8,-13.0099223804886,-6.26088029236732));
#20338=CARTESIAN_POINT('Ctrl Pts',(15.8,-13.0017929656379,-6.25785139447984));
#20339=CARTESIAN_POINT('Ctrl Pts',(15.8,-12.993640869393,-6.25486539490331));
#20340=CARTESIAN_POINT('Ctrl Pts',(15.8,-12.985466096197,-6.25192228516409));
#20341=CARTESIAN_POINT('Ctrl Pts',(15.8,-12.9772686462497,-6.24902206502841));
#20342=CARTESIAN_POINT('Origin',(15.8,-12.9255771089134,-7.7277884589423));
#20343=CARTESIAN_POINT('Ctrl Pts',(10.0502525316942,-9.78902788303806,-4.46902397810655));
#20344=CARTESIAN_POINT('Ctrl Pts',(11.9668350211294,-11.9845316814717,-4.39491126897609));
#20345=CARTESIAN_POINT('Ctrl Pts',(13.8834175105647,-14.1800354799052,-4.32079855984563));
#20346=CARTESIAN_POINT('Ctrl Pts',(15.8,-16.3755392783388,-4.24668585071518));
#20347=CARTESIAN_POINT('Ctrl Pts',(10.0502525316942,-9.8524662840083,-4.20205396612197));
#20348=CARTESIAN_POINT('Ctrl Pts',(11.9668350211294,-12.036617299121,-4.07988582479457));
#20349=CARTESIAN_POINT('Ctrl Pts',(13.8834175105647,-14.2208423566523,-3.95733982070599));
#20350=CARTESIAN_POINT('Ctrl Pts',(15.8,-16.404993371765,-3.83517167937859));
#20351=CARTESIAN_POINT('Ctrl Pts',(10.0502525316942,-9.90590216992165,-3.78556561092159));
#20352=CARTESIAN_POINT('Ctrl Pts',(11.9668350211295,-12.0646697130184,-3.58873319698333));
#20353=CARTESIAN_POINT('Ctrl Pts',(13.8834175105647,-14.2233509855394,-3.39243568541409));
#20354=CARTESIAN_POINT('Ctrl Pts',(15.8,-16.3821185286362,-3.19560327147583));
#20355=CARTESIAN_POINT('Ctrl Pts',(10.0502525316942,-9.80521299123422,-3.57425782911966));
#20356=CARTESIAN_POINT('Ctrl Pts',(11.9668350211295,-11.9287659082934,-3.34323666910061));
#20357=CARTESIAN_POINT('Ctrl Pts',(13.8834175105647,-14.0522999619539,-3.11226431322854));
#20358=CARTESIAN_POINT('Ctrl Pts',(15.8,-16.1758528790132,-2.8812431532095));
#20359=CARTESIAN_POINT('Ctrl Pts',(10.0502525316942,-9.71169428155716,-3.47602249721152));
#20360=CARTESIAN_POINT('Ctrl Pts',(11.9668350211295,-11.8094568448422,-3.23326515211326));
#20361=CARTESIAN_POINT('Ctrl Pts',(13.8834175105647,-13.9072965714997,-2.99011502771357));
#20362=CARTESIAN_POINT('Ctrl Pts',(15.8,-16.0050591347847,-2.74735768261532));
#20363=CARTESIAN_POINT('Ctrl Pts',(10.0502525316942,-9.64719632995103,-3.414097226746));
#20364=CARTESIAN_POINT('Ctrl Pts',(11.9668350211295,-11.7274687236956,-3.16465335082917));
#20365=CARTESIAN_POINT('Ctrl Pts',(13.8834175105647,-13.8077428217682,-2.91499625447087));
#20366=CARTESIAN_POINT('Ctrl Pts',(15.8,-15.8880152155128,-2.66555237855405));
#20367=CARTESIAN_POINT('Ctrl Pts',(10.0502525316942,-9.53672408685997,-3.30251999207182));
#20368=CARTESIAN_POINT('Ctrl Pts',(11.9668350211294,-11.58577497799,-3.04246362184766));
#20369=CARTESIAN_POINT('Ctrl Pts',(13.8834175105647,-13.6349367240444,-2.78215337892879));
#20370=CARTESIAN_POINT('Ctrl Pts',(15.8,-15.6839876151744,-2.52209700870464));
#20371=CARTESIAN_POINT('Ctrl Pts',(10.0502525316942,-9.36058107581316,-3.09139659750779));
#20372=CARTESIAN_POINT('Ctrl Pts',(11.9668350211295,-11.357410148179,-2.80829724126978));
#20373=CARTESIAN_POINT('Ctrl Pts',(13.8834175105647,-13.3541948572957,-2.52507603204706));
#20374=CARTESIAN_POINT('Ctrl Pts',(15.8,-15.3510239296616,-2.24197667580905));
#20375=CARTESIAN_POINT('Ctrl Pts',(10.0502525316942,-9.14733948977135,-2.94903314862294));
#20376=CARTESIAN_POINT('Ctrl Pts',(11.9668350211294,-11.0909774008914,-2.65653626154118));
#20377=CARTESIAN_POINT('Ctrl Pts',(13.8834175105647,-13.0346322911662,-2.3639289644162));
#20378=CARTESIAN_POINT('Ctrl Pts',(15.8,-14.9782702022863,-2.07143207733444));
#20379=CARTESIAN_POINT('Ctrl Pts',(10.0502525316942,-8.92650608260145,-2.83936642791009));
#20380=CARTESIAN_POINT('Ctrl Pts',(11.9668350211294,-10.8177624863471,-2.54644119432444));
#20381=CARTESIAN_POINT('Ctrl Pts',(13.8834175105648,-12.7090406610097,-2.2534334908895));
#20382=CARTESIAN_POINT('Ctrl Pts',(15.8,-14.6002970647553,-1.96050825730385));
#20383=CARTESIAN_POINT('Ctrl Pts',(10.0502525316942,-8.80866270544546,-2.80374461319022));
#20384=CARTESIAN_POINT('Ctrl Pts',(11.9668350211294,-10.6741860277864,-2.51464388608039));
#20385=CARTESIAN_POINT('Ctrl Pts',(13.8834175105647,-12.5396724561545,-2.22549660720977));
#20386=CARTESIAN_POINT('Ctrl Pts',(15.8,-14.4051957784954,-1.93639588009993));
#20387=CARTESIAN_POINT('Ctrl Pts',(10.0502525316942,-8.7276078365385,-2.78743136471945));
#20388=CARTESIAN_POINT('Ctrl Pts',(11.9668350211294,-10.5761285330411,-2.50261311086535));
#20389=CARTESIAN_POINT('Ctrl Pts',(13.8834175105647,-12.4246492295437,-2.21779485701124));
#20390=CARTESIAN_POINT('Ctrl Pts',(15.8,-14.2731699260464,-1.93297660315714));
#20391=CARTESIAN_POINT('Ctrl Pts',(15.8,-14.3165490635069,-1.93458023611785));
#20392=CARTESIAN_POINT('Ctrl Pts',(15.8,-14.3078898665466,-1.93416388872989));
#20393=CARTESIAN_POINT('Ctrl Pts',(15.8,-14.2992223526576,-1.93379536300002));
#20394=CARTESIAN_POINT('Ctrl Pts',(15.8,-14.2905465237881,-1.93347464492456));
#20395=CARTESIAN_POINT('Ctrl Pts',(15.8,-14.2818623815451,-1.93320172507161));
#20396=CARTESIAN_POINT('Ctrl Pts',(15.8,-14.2731699260464,-1.93297660315714));
#20397=CARTESIAN_POINT('Origin',(15.8,-14.6809722990553,-3.35534058166953));
#20398=CARTESIAN_POINT('Ctrl Pts',(10.0502525316942,-10.6909231138624,-1.22531840158854));
#20399=CARTESIAN_POINT('Ctrl Pts',(11.9668350211294,-12.7560692212929,-0.47638504169901));
#20400=CARTESIAN_POINT('Ctrl Pts',(13.8834175105647,-14.8212153287235,0.272548318190525));
#20401=CARTESIAN_POINT('Ctrl Pts',(15.8,-16.886361436154,1.02148167808006));
#20402=CARTESIAN_POINT('Ctrl Pts',(10.0502525316942,-10.6687583477967,-0.951811288039438));
#20403=CARTESIAN_POINT('Ctrl Pts',(11.9668350211294,-12.7082628707158,-0.160771418505767));
#20404=CARTESIAN_POINT('Ctrl Pts',(13.8834175105647,-14.7477045483503,0.630916858166453));
#20405=CARTESIAN_POINT('Ctrl Pts',(15.8,-16.7872090712694,1.42195672770012));
#20406=CARTESIAN_POINT('Ctrl Pts',(10.0502525316942,-10.5909841198542,-0.538737970192931));
#20407=CARTESIAN_POINT('Ctrl Pts',(11.9668350211295,-12.5832583421986,0.315735593698358));
#20408=CARTESIAN_POINT('Ctrl Pts',(13.8834175105647,-14.5756107736058,1.16942659814004));
#20409=CARTESIAN_POINT('Ctrl Pts',(15.8,-16.5678849959503,2.02390016203133));
#20410=CARTESIAN_POINT('Ctrl Pts',(10.0502525316942,-10.4118557126012,-0.350797420983485));
#20411=CARTESIAN_POINT('Ctrl Pts',(11.9668350211295,-12.3552036734465,0.527317792292715));
#20412=CARTESIAN_POINT('Ctrl Pts',(13.8834175105647,-14.2985259967778,1.40583184426593));
#20413=CARTESIAN_POINT('Ctrl Pts',(15.8,-16.2418739576232,2.28394705754213));
#20414=CARTESIAN_POINT('Ctrl Pts',(10.0502525316942,-10.2498870013208,-0.276502431596343));
#20415=CARTESIAN_POINT('Ctrl Pts',(11.9668350211295,-12.1559807242605,0.603405794214881));
#20416=CARTESIAN_POINT('Ctrl Pts',(13.8834175105647,-14.0620012424206,1.48361038150706));
#20417=CARTESIAN_POINT('Ctrl Pts',(15.8,-15.9680949653604,2.36351860731828));
#20418=CARTESIAN_POINT('Ctrl Pts',(10.0502525316942,-10.0905890686414,-0.193479460458702));
#20419=CARTESIAN_POINT('Ctrl Pts',(11.9668350211294,-11.9589846875421,0.687106219194376));
#20420=CARTESIAN_POINT('Ctrl Pts',(13.8834175105647,-13.8273908205778,1.56802487912709));
#20421=CARTESIAN_POINT('Ctrl Pts',(15.8,-15.6957864394785,2.44861055878017));
#20422=CARTESIAN_POINT('Ctrl Pts',(10.0502525316942,-9.85767148446325,-0.0477779613143529));
#20423=CARTESIAN_POINT('Ctrl Pts',(11.9668350211294,-11.6692901486065,0.83847512310783));
#20424=CARTESIAN_POINT('Ctrl Pts',(13.8834175105647,-13.4808398643785,1.72481200902093));
#20425=CARTESIAN_POINT('Ctrl Pts',(15.8,-15.2924585285217,2.61106509344311));
#20426=CARTESIAN_POINT('Ctrl Pts',(10.0502525316942,-9.61095465953459,0.0220599042734176));
#20427=CARTESIAN_POINT('Ctrl Pts',(11.9668350211294,-11.3690757684926,0.900879773662287));
#20428=CARTESIAN_POINT('Ctrl Pts',(13.8834175105647,-13.1271782591657,1.77979551853006));
#20429=CARTESIAN_POINT('Ctrl Pts',(15.8,-14.8852993681237,2.65861538791893));
#20430=CARTESIAN_POINT('Ctrl Pts',(10.0502525316942,-9.36700900338232,0.0579833517275573));
#20431=CARTESIAN_POINT('Ctrl Pts',(11.9668350211294,-11.07518337287,0.92098471111409));
#20432=CARTESIAN_POINT('Ctrl Pts',(13.8834175105647,-12.7833535968728,1.78409102238058));
#20433=CARTESIAN_POINT('Ctrl Pts',(15.8,-14.4915279663605,2.64709238176711));
#20434=CARTESIAN_POINT('Ctrl Pts',(10.0502525316942,-9.243940799223,0.0555068892974579));
#20435=CARTESIAN_POINT('Ctrl Pts',(11.9668350211294,-10.9288207869826,0.906948929192824));
#20436=CARTESIAN_POINT('Ctrl Pts',(13.8834175105647,-12.6136545606744,1.75838634306183));
#20437=CARTESIAN_POINT('Ctrl Pts',(15.8,-14.298534548434,2.6098283829572));
#20438=CARTESIAN_POINT('Ctrl Pts',(10.0502525316942,-9.16181196696065,0.0459743785884369));
#20439=CARTESIAN_POINT('Ctrl Pts',(11.9668350211294,-10.8318459401268,0.888076944549315));
#20440=CARTESIAN_POINT('Ctrl Pts',(13.8834175105647,-12.501879913293,1.73017951051019));
#20441=CARTESIAN_POINT('Ctrl Pts',(15.8,-14.1719138864591,2.57228207647107));
#20442=CARTESIAN_POINT('Ctrl Pts',(15.8,-14.2136654476498,2.58416182157067));
#20443=CARTESIAN_POINT('Ctrl Pts',(15.8,-14.2053014035364,2.58188195244865));
#20444=CARTESIAN_POINT('Ctrl Pts',(15.8,-14.1969442272588,2.57955403215479));
#20445=CARTESIAN_POINT('Ctrl Pts',(15.8,-14.1885939163425,2.57717807460939));
#20446=CARTESIAN_POINT('Ctrl Pts',(15.8,-14.1802504694012,2.57475408927931));
#20447=CARTESIAN_POINT('Ctrl Pts',(15.8,-14.1719138864591,2.57228207647107));
#20448=CARTESIAN_POINT('Origin',(15.8,-14.999291632217,1.34555140976956));
#20449=CARTESIAN_POINT('Ctrl Pts',(10.0502525316942,-10.5463163022605,2.13832987737225));
#20450=CARTESIAN_POINT('Ctrl Pts',(11.9668350211294,-12.2789538289737,3.48877307262933));
#20451=CARTESIAN_POINT('Ctrl Pts',(13.8834175105647,-14.0115913556869,4.8392162678864));
#20452=CARTESIAN_POINT('Ctrl Pts',(15.8,-15.7442288824001,6.18965946314348));
#20453=CARTESIAN_POINT('Ctrl Pts',(10.0502525316942,-10.4407180108925,2.39160131057558));
#20454=CARTESIAN_POINT('Ctrl Pts',(11.9668350211294,-12.1359573145141,3.77416649083142));
#20455=CARTESIAN_POINT('Ctrl Pts',(13.8834175105647,-13.8309364798931,5.15732892266062));
#20456=CARTESIAN_POINT('Ctrl Pts',(15.8,-15.5261757835147,6.53989410291645));
#20457=CARTESIAN_POINT('Ctrl Pts',(10.0502525316942,-10.2391038402362,2.76042111194549));
#20458=CARTESIAN_POINT('Ctrl Pts',(11.9668350211294,-11.8698223691572,4.18872035504581));
#20459=CARTESIAN_POINT('Ctrl Pts',(13.8834175105647,-13.5008577836237,5.61629814839673));
#20460=CARTESIAN_POINT('Ctrl Pts',(15.8,-15.1315763125447,7.04459739149705));
#20461=CARTESIAN_POINT('Ctrl Pts',(10.0502525316942,-10.0106660065973,2.88380634898392));
#20462=CARTESIAN_POINT('Ctrl Pts',(11.9668350211294,-11.5875472242667,4.31947109051328));
#20463=CARTESIAN_POINT('Ctrl Pts',(13.8834175105647,-13.1642822866715,5.75550424110768));
#20464=CARTESIAN_POINT('Ctrl Pts',(15.8,-14.7411635043409,7.19116898263704));
#20465=CARTESIAN_POINT('Ctrl Pts',(10.0502525316942,-9.83366631411429,2.90441220847246));
#20466=CARTESIAN_POINT('Ctrl Pts',(11.9668350211294,-11.3745625747195,4.33027001363174));
#20467=CARTESIAN_POINT('Ctrl Pts',(13.8834175105647,-12.9152995332973,5.75638324902558));
#20468=CARTESIAN_POINT('Ctrl Pts',(15.8,-14.4561957939025,7.18224105418486));
#20469=CARTESIAN_POINT('Ctrl Pts',(10.0502525316941,-9.65650945139357,2.93414649567711));
#20470=CARTESIAN_POINT('Ctrl Pts',(11.9668350211294,-11.1613433397504,4.34899924292338));
#20471=CARTESIAN_POINT('Ctrl Pts',(13.8834175105647,-12.6660861533134,5.76416819477547));
#20472=CARTESIAN_POINT('Ctrl Pts',(15.8,-14.1709200416702,7.17902094202174));
#20473=CARTESIAN_POINT('Ctrl Pts',(10.0502525316942,-9.38996734645582,3.00074150798572));
#20474=CARTESIAN_POINT('Ctrl Pts',(11.9668350211294,-10.8390518176275,4.40343923355921));
#20475=CARTESIAN_POINT('Ctrl Pts',(13.8834175105647,-12.2880463890101,5.8061924752444));
#20476=CARTESIAN_POINT('Ctrl Pts',(15.8,-13.7371308601818,7.20889020081789));
#20477=CARTESIAN_POINT('Ctrl Pts',(10.0502525316942,-9.13374448664767,2.99092345166592));
#20478=CARTESIAN_POINT('Ctrl Pts',(11.9668350211294,-10.5342467491227,4.37002011593521));
#20479=CARTESIAN_POINT('Ctrl Pts',(13.8834175105647,-11.9347028120052,5.74920012742636));
#20480=CARTESIAN_POINT('Ctrl Pts',(15.8,-13.3352050744802,7.12829679169565));
#20481=CARTESIAN_POINT('Ctrl Pts',(10.0502525316942,-8.89063737063807,2.94970615383951));
#20482=CARTESIAN_POINT('Ctrl Pts',(11.9668350211294,-10.2485256494886,4.29832412978306));
#20483=CARTESIAN_POINT('Ctrl Pts',(13.8834175105647,-11.6063785007713,5.64703889510258));
#20484=CARTESIAN_POINT('Ctrl Pts',(15.8,-12.9642667796218,6.99565687104613));
#20485=CARTESIAN_POINT('Ctrl Pts',(10.0502525316942,-8.77435756124986,2.90932499072146));
#20486=CARTESIAN_POINT('Ctrl Pts',(11.9668350211294,-10.113663592731,4.23975104071156));
#20487=CARTESIAN_POINT('Ctrl Pts',(13.8834175105647,-11.4529271015425,5.57015841015681));
#20488=CARTESIAN_POINT('Ctrl Pts',(15.8,-12.7922331330237,6.90058446014691));
#20489=CARTESIAN_POINT('Ctrl Pts',(10.0502525316942,-8.69919410795919,2.87487982939776));
#20490=CARTESIAN_POINT('Ctrl Pts',(11.9668350211294,-10.0272667966845,4.19183584103558));
#20491=CARTESIAN_POINT('Ctrl Pts',(13.8834175105647,-11.3553394854098,5.5087918526734));
#20492=CARTESIAN_POINT('Ctrl Pts',(15.8,-12.6834121741351,6.82574786431122));
#20493=CARTESIAN_POINT('Ctrl Pts',(15.8,-12.7194492253464,6.84994811524973));
#20494=CARTESIAN_POINT('Ctrl Pts',(15.8,-12.7121990649934,6.84519519909218));
#20495=CARTESIAN_POINT('Ctrl Pts',(15.8,-12.7049702849691,6.84039870583253));
#20496=CARTESIAN_POINT('Ctrl Pts',(15.8,-12.6977628786185,6.83555864794507));
#20497=CARTESIAN_POINT('Ctrl Pts',(15.8,-12.6905768416977,6.83067503400497));
#20498=CARTESIAN_POINT('Ctrl Pts',(15.8,-12.6834121741351,6.82574786431122));
#20499=CARTESIAN_POINT('Origin',(15.8,-13.8493757942074,5.91473145421246));
#20500=CARTESIAN_POINT('Ctrl Pts',(10.0502525316942,-9.36936257048691,5.29266352931554));
#20501=CARTESIAN_POINT('Ctrl Pts',(11.9668350211294,-10.5998888833726,7.11242577089738));
#20502=CARTESIAN_POINT('Ctrl Pts',(13.8834175105647,-11.8304151962582,8.93218801247923));
#20503=CARTESIAN_POINT('Ctrl Pts',(15.8,-13.0609415091439,10.7519502540611));
#20504=CARTESIAN_POINT('Ctrl Pts',(10.0502525316942,-9.19066745032221,5.50090730964532));
#20505=CARTESIAN_POINT('Ctrl Pts',(11.9668350211294,-10.3756997001811,7.33966268788185));
#20506=CARTESIAN_POINT('Ctrl Pts',(13.8834175105647,-11.5602999829831,9.17890569898124));
#20507=CARTESIAN_POINT('Ctrl Pts',(15.8,-12.745332232842,11.0176610772178));
#20508=CARTESIAN_POINT('Ctrl Pts',(10.0502525316942,-8.88494866314842,5.78937538435653));
#20509=CARTESIAN_POINT('Ctrl Pts',(11.9668350211294,-9.99448540715111,7.65168842520523));
#20510=CARTESIAN_POINT('Ctrl Pts',(13.8834175105647,-11.104545703274,9.51341402508183));
#20511=CARTESIAN_POINT('Ctrl Pts',(15.8,-12.2140824472766,11.3757270659305));
#20512=CARTESIAN_POINT('Ctrl Pts',(10.0502525316942,-8.62956238511758,5.83613263565859));
#20513=CARTESIAN_POINT('Ctrl Pts',(11.9668350211294,-9.68562073924798,7.68881403767578));
#20514=CARTESIAN_POINT('Ctrl Pts',(13.8834175105647,-10.7414245752752,9.54180236671465));
#20515=CARTESIAN_POINT('Ctrl Pts',(15.8,-11.7974829294056,11.3944837687318));
#20516=CARTESIAN_POINT('Ctrl Pts',(10.0502525316942,-8.45485763321061,5.80103525788045));
#20517=CARTESIAN_POINT('Ctrl Pts',(11.9668350211294,-9.47972276943763,7.6332697458833));
#20518=CARTESIAN_POINT('Ctrl Pts',(13.8834175105647,-10.5043553237743,9.46570011434025));
#20519=CARTESIAN_POINT('Ctrl Pts',(15.8,-11.5292204600013,11.2979346023431));
#20520=CARTESIAN_POINT('Ctrl Pts',(10.0502525316941,-8.27718317134364,5.77456941285602));
#20521=CARTESIAN_POINT('Ctrl Pts',(11.9668350211294,-9.27115170336996,7.58519358293626));
#20522=CARTESIAN_POINT('Ctrl Pts',(13.8834175105647,-10.2649338319875,9.39609248134292));
#20523=CARTESIAN_POINT('Ctrl Pts',(15.8,-11.2589023640139,11.2067166514232));
#20524=CARTESIAN_POINT('Ctrl Pts',(10.0502525316942,-8.0031076613001,5.75553891274799));
#20525=CARTESIAN_POINT('Ctrl Pts',(11.9668350211295,-8.94781145509674,7.53737545292393));
#20526=CARTESIAN_POINT('Ctrl Pts',(13.8834175105647,-9.89241088219744,9.31923862861202));
#20527=CARTESIAN_POINT('Ctrl Pts',(15.8,-10.8371146759941,11.101075168788));
#20528=CARTESIAN_POINT('Ctrl Pts',(10.0502525316942,-7.76245969237558,5.66702291215723));
#20529=CARTESIAN_POINT('Ctrl Pts',(11.9668350211294,-8.66825218904355,7.4114007810768));
#20530=CARTESIAN_POINT('Ctrl Pts',(13.8834175105647,-9.57397375447812,9.1558448117796));
#20531=CARTESIAN_POINT('Ctrl Pts',(15.8,-10.4797662511461,10.9002226806992));
#20532=CARTESIAN_POINT('Ctrl Pts',(10.0502525316942,-7.54398815168985,5.55269814935977));
#20533=CARTESIAN_POINT('Ctrl Pts',(11.9668350211294,-8.41867077420536,7.25492061800102));
#20534=CARTESIAN_POINT('Ctrl Pts',(13.8834175105647,-9.29328875951756,8.95722517253276));
#20535=CARTESIAN_POINT('Ctrl Pts',(15.8,-10.1679713820331,10.659447641174));
#20536=CARTESIAN_POINT('Ctrl Pts',(10.0502525316942,-7.44587907063767,5.47835809159451));
#20537=CARTESIAN_POINT('Ctrl Pts',(11.9668350211294,-8.30851053998513,7.15753678028296));
#20538=CARTESIAN_POINT('Ctrl Pts',(13.8834175105647,-9.17110734047641,8.83668456248994));
#20539=CARTESIAN_POINT('Ctrl Pts',(15.8,-10.0337388098239,10.5158632511784));
#20540=CARTESIAN_POINT('Ctrl Pts',(10.0502525316942,-7.38503851882133,5.42237201204004));
#20541=CARTESIAN_POINT('Ctrl Pts',(11.9668350211294,-8.24114891510682,7.08526863916361));
#20542=CARTESIAN_POINT('Ctrl Pts',(13.8834175105647,-9.09725931139231,8.74816526628719));
#20543=CARTESIAN_POINT('Ctrl Pts',(15.8,-9.95336970767779,10.4110618934108));
#20544=CARTESIAN_POINT('Ctrl Pts',(15.8,-9.9801646912522,10.4452137610133));
#20545=CARTESIAN_POINT('Ctrl Pts',(15.8,-9.97473811086981,10.4384530463692));
#20546=CARTESIAN_POINT('Ctrl Pts',(15.8,-9.96934533045351,10.4316574943231));
#20547=CARTESIAN_POINT('Ctrl Pts',(15.8,-9.96398633981914,10.4248271146823));
#20548=CARTESIAN_POINT('Ctrl Pts',(15.8,-9.95866113228077,10.4179619142908));
#20549=CARTESIAN_POINT('Ctrl Pts',(15.8,-9.95336970767779,10.4110618934108));
#20550=CARTESIAN_POINT('Origin',(15.8,-11.3437865591856,9.90493637355978));
#20551=CARTESIAN_POINT('Ctrl Pts',(10.0502525316942,-7.2752703501265,7.92891439885425));
#20552=CARTESIAN_POINT('Ctrl Pts',(11.9668350211294,-7.88323296009842,10.0398646795257));
#20553=CARTESIAN_POINT('Ctrl Pts',(13.8834175105647,-8.49119557007034,12.1508149601973));
#20554=CARTESIAN_POINT('Ctrl Pts',(15.8,-9.09915818004226,14.2617652408688));
#20555=CARTESIAN_POINT('Ctrl Pts',(10.0502525316942,-7.04097032456894,8.07174617417205));
#20556=CARTESIAN_POINT('Ctrl Pts',(11.9668350211294,-7.59972129962698,10.186749261509));
#20557=CARTESIAN_POINT('Ctrl Pts',(13.8834175105647,-8.15813578620935,12.3019395333854));
#20558=CARTESIAN_POINT('Ctrl Pts',(15.8,-8.71688676126738,14.4169426207224));
#20559=CARTESIAN_POINT('Ctrl Pts',(10.0502525316942,-6.66138127597024,8.25126590443755));
#20560=CARTESIAN_POINT('Ctrl Pts',(11.9668350211294,-7.14127838379811,10.365200404417));
#20561=CARTESIAN_POINT('Ctrl Pts',(13.8834175105647,-7.62165928459738,12.4788866778492));
#20562=CARTESIAN_POINT('Ctrl Pts',(15.8,-8.10155639242525,14.5928211778286));
#20563=CARTESIAN_POINT('Ctrl Pts',(10.0502525316942,-6.42930419296208,8.22079862024225));
#20564=CARTESIAN_POINT('Ctrl Pts',(11.9668350211294,-6.86580395314968,10.3118069242151));
#20565=CARTESIAN_POINT('Ctrl Pts',(13.8834175105647,-7.3023483954802,12.4027801127282));
#20566=CARTESIAN_POINT('Ctrl Pts',(15.8,-7.73884815566781,14.493788416701));
#20567=CARTESIAN_POINT('Ctrl Pts',(10.0502525316942,-6.30697938690416,8.16221173215364));
#20568=CARTESIAN_POINT('Ctrl Pts',(11.9668350211294,-6.72434771418857,10.2323186327506));
#20569=CARTESIAN_POINT('Ctrl Pts',(13.8834175105647,-7.14137150628509,12.3026176380752));
#20570=CARTESIAN_POINT('Ctrl Pts',(15.8,-7.5587398335695,14.3727245386721));
#20571=CARTESIAN_POINT('Ctrl Pts',(10.0502525316942,-6.22815403351084,8.12000643506485));
#20572=CARTESIAN_POINT('Ctrl Pts',(11.9668350211294,-6.63375833246635,10.1755454476056));
#20573=CARTESIAN_POINT('Ctrl Pts',(13.8834175105647,-7.03916552489902,12.2311493413123));
#20574=CARTESIAN_POINT('Ctrl Pts',(15.8,-7.44476982385453,14.2866883538531));
#20575=CARTESIAN_POINT('Ctrl Pts',(10.0502525316942,-6.08789997184504,8.04942040067478));
#20576=CARTESIAN_POINT('Ctrl Pts',(11.9668350211294,-6.47376321403759,10.0785454407991));
#20577=CARTESIAN_POINT('Ctrl Pts',(13.8834175105647,-6.85942462405723,12.1078515605739));
#20578=CARTESIAN_POINT('Ctrl Pts',(15.8,-7.24528786624977,14.1369766006982));
#20579=CARTESIAN_POINT('Ctrl Pts',(10.0502525316942,-5.83267830770085,7.94713925110583));
#20580=CARTESIAN_POINT('Ctrl Pts',(11.9668350211294,-6.18048893841474,9.93371906448112));
#20581=CARTESIAN_POINT('Ctrl Pts',(13.8834175105647,-6.52817426230451,11.920292369998));
#20582=CARTESIAN_POINT('Ctrl Pts',(15.8,-6.87598489301839,13.9068721833733));
#20583=CARTESIAN_POINT('Ctrl Pts',(10.0502525316942,-5.63138575926578,7.78832910259187));
#20584=CARTESIAN_POINT('Ctrl Pts',(11.9668350211294,-5.95382183425814,9.7272251121909));
#20585=CARTESIAN_POINT('Ctrl Pts',(13.8834175105647,-6.27616146093385,11.6661698490829));
#20586=CARTESIAN_POINT('Ctrl Pts',(15.8,-6.59859753592621,13.605065858682));
#20587=CARTESIAN_POINT('Ctrl Pts',(10.0502525316942,-5.45884429554414,7.61219406851115));
#20588=CARTESIAN_POINT('Ctrl Pts',(11.9668350211294,-5.76468621283309,9.50140467053763));
#20589=CARTESIAN_POINT('Ctrl Pts',(13.8834175105647,-6.07045912241827,11.3906602079427));
#20590=CARTESIAN_POINT('Ctrl Pts',(15.8,-6.37630103970722,13.2798708099692));
#20591=CARTESIAN_POINT('Ctrl Pts',(10.0502525316942,-5.38854605810145,7.51113133249701));
#20592=CARTESIAN_POINT('Ctrl Pts',(11.9668350211294,-5.69007333772413,9.37468648227302));
#20593=CARTESIAN_POINT('Ctrl Pts',(13.8834175105647,-5.99154494312677,11.238220929081));
#20594=CARTESIAN_POINT('Ctrl Pts',(15.8,-6.29307222274945,13.101776078857));
#20595=CARTESIAN_POINT('Ctrl Pts',(10.0502525316942,-5.34798390487229,7.43908464225652));
#20596=CARTESIAN_POINT('Ctrl Pts',(11.9668350211294,-5.64832995825767,9.28514597692092));
#20597=CARTESIAN_POINT('Ctrl Pts',(13.8834175105647,-5.94867601164304,11.1312073115853));
#20598=CARTESIAN_POINT('Ctrl Pts',(15.8,-6.24902206502841,12.9772686462497));
#20599=CARTESIAN_POINT('Ctrl Pts',(15.8,-6.26395210128206,13.0180291077652));
#20600=CARTESIAN_POINT('Ctrl Pts',(15.8,-6.26088029236732,13.0099223804886));
#20601=CARTESIAN_POINT('Ctrl Pts',(15.8,-6.25785139447984,13.0017929656379));
#20602=CARTESIAN_POINT('Ctrl Pts',(15.8,-6.25486539490331,12.993640869393));
#20603=CARTESIAN_POINT('Ctrl Pts',(15.8,-6.25192228516409,12.985466096197));
#20604=CARTESIAN_POINT('Ctrl Pts',(15.8,-6.24902206502841,12.9772686462497));
#20605=CARTESIAN_POINT('Origin',(15.8,-7.7277884589423,12.9255771089134));
#20606=CARTESIAN_POINT('Ctrl Pts',(10.0502525316942,-4.46902397810655,9.78902788303806));
#20607=CARTESIAN_POINT('Ctrl Pts',(11.9668350211294,-4.39491126897609,11.9845316814717));
#20608=CARTESIAN_POINT('Ctrl Pts',(13.8834175105647,-4.32079855984564,14.1800354799052));
#20609=CARTESIAN_POINT('Ctrl Pts',(15.8,-4.24668585071518,16.3755392783388));
#20610=CARTESIAN_POINT('Ctrl Pts',(10.0502525316942,-4.20205396612196,9.8524662840083));
#20611=CARTESIAN_POINT('Ctrl Pts',(11.9668350211294,-4.07988582479457,12.036617299121));
#20612=CARTESIAN_POINT('Ctrl Pts',(13.8834175105647,-3.95733982070598,14.2208423566523));
#20613=CARTESIAN_POINT('Ctrl Pts',(15.8,-3.83517167937858,16.404993371765));
#20614=CARTESIAN_POINT('Ctrl Pts',(10.0502525316942,-3.78556561092159,9.90590216992165));
#20615=CARTESIAN_POINT('Ctrl Pts',(11.9668350211295,-3.58873319698333,12.0646697130184));
#20616=CARTESIAN_POINT('Ctrl Pts',(13.8834175105647,-3.39243568541408,14.2233509855394));
#20617=CARTESIAN_POINT('Ctrl Pts',(15.8,-3.19560327147581,16.3821185286362));
#20618=CARTESIAN_POINT('Ctrl Pts',(10.0502525316942,-3.57425782911967,9.80521299123422));
#20619=CARTESIAN_POINT('Ctrl Pts',(11.9668350211295,-3.34323666910062,11.9287659082934));
#20620=CARTESIAN_POINT('Ctrl Pts',(13.8834175105647,-3.11226431322854,14.0522999619539));
#20621=CARTESIAN_POINT('Ctrl Pts',(15.8,-2.8812431532095,16.1758528790131));
#20622=CARTESIAN_POINT('Ctrl Pts',(10.0502525316942,-3.47602249721152,9.71169428155716));
#20623=CARTESIAN_POINT('Ctrl Pts',(11.9668350211295,-3.23326515211327,11.8094568448422));
#20624=CARTESIAN_POINT('Ctrl Pts',(13.8834175105647,-2.99011502771357,13.9072965714997));
#20625=CARTESIAN_POINT('Ctrl Pts',(15.8,-2.74735768261532,16.0050591347847));
#20626=CARTESIAN_POINT('Ctrl Pts',(10.0502525316942,-3.414097226746,9.64719632995103));
#20627=CARTESIAN_POINT('Ctrl Pts',(11.9668350211295,-3.16465335082918,11.7274687236956));
#20628=CARTESIAN_POINT('Ctrl Pts',(13.8834175105647,-2.91499625447087,13.8077428217682));
#20629=CARTESIAN_POINT('Ctrl Pts',(15.8,-2.66555237855405,15.8880152155128));
#20630=CARTESIAN_POINT('Ctrl Pts',(10.0502525316942,-3.30251999207182,9.53672408685997));
#20631=CARTESIAN_POINT('Ctrl Pts',(11.9668350211294,-3.04246362184766,11.58577497799));
#20632=CARTESIAN_POINT('Ctrl Pts',(13.8834175105647,-2.7821533789288,13.6349367240444));
#20633=CARTESIAN_POINT('Ctrl Pts',(15.8,-2.52209700870464,15.6839876151744));
#20634=CARTESIAN_POINT('Ctrl Pts',(10.0502525316942,-3.09139659750779,9.36058107581316));
#20635=CARTESIAN_POINT('Ctrl Pts',(11.9668350211295,-2.80829724126978,11.357410148179));
#20636=CARTESIAN_POINT('Ctrl Pts',(13.8834175105647,-2.52507603204707,13.3541948572957));
#20637=CARTESIAN_POINT('Ctrl Pts',(15.8,-2.24197667580906,15.3510239296616));
#20638=CARTESIAN_POINT('Ctrl Pts',(10.0502525316942,-2.94903314862294,9.14733948977135));
#20639=CARTESIAN_POINT('Ctrl Pts',(11.9668350211294,-2.65653626154119,11.0909774008914));
#20640=CARTESIAN_POINT('Ctrl Pts',(13.8834175105647,-2.36392896441619,13.0346322911662));
#20641=CARTESIAN_POINT('Ctrl Pts',(15.8,-2.07143207733444,14.9782702022863));
#20642=CARTESIAN_POINT('Ctrl Pts',(10.0502525316942,-2.83936642791009,8.92650608260145));
#20643=CARTESIAN_POINT('Ctrl Pts',(11.9668350211294,-2.54644119432445,10.8177624863471));
#20644=CARTESIAN_POINT('Ctrl Pts',(13.8834175105648,-2.25343349088951,12.7090406610097));
#20645=CARTESIAN_POINT('Ctrl Pts',(15.8,-1.96050825730386,14.6002970647553));
#20646=CARTESIAN_POINT('Ctrl Pts',(10.0502525316942,-2.80374461319022,8.80866270544546));
#20647=CARTESIAN_POINT('Ctrl Pts',(11.9668350211294,-2.51464388608039,10.6741860277864));
#20648=CARTESIAN_POINT('Ctrl Pts',(13.8834175105647,-2.22549660720977,12.5396724561545));
#20649=CARTESIAN_POINT('Ctrl Pts',(15.8,-1.93639588009993,14.4051957784954));
#20650=CARTESIAN_POINT('Ctrl Pts',(10.0502525316942,-2.78743136471945,8.7276078365385));
#20651=CARTESIAN_POINT('Ctrl Pts',(11.9668350211294,-2.50261311086535,10.5761285330411));
#20652=CARTESIAN_POINT('Ctrl Pts',(13.8834175105647,-2.21779485701124,12.4246492295437));
#20653=CARTESIAN_POINT('Ctrl Pts',(15.8,-1.93297660315714,14.2731699260464));
#20654=CARTESIAN_POINT('Ctrl Pts',(15.8,-1.93458023611785,14.3165490635069));
#20655=CARTESIAN_POINT('Ctrl Pts',(15.8,-1.93416388872989,14.3078898665466));
#20656=CARTESIAN_POINT('Ctrl Pts',(15.8,-1.93379536300002,14.2992223526576));
#20657=CARTESIAN_POINT('Ctrl Pts',(15.8,-1.93347464492456,14.2905465237881));
#20658=CARTESIAN_POINT('Ctrl Pts',(15.8,-1.93320172507161,14.2818623815451));
#20659=CARTESIAN_POINT('Ctrl Pts',(15.8,-1.93297660315714,14.2731699260464));
#20660=CARTESIAN_POINT('Origin',(15.8,-3.35534058166953,14.6809722990553));
#20661=CARTESIAN_POINT('Ctrl Pts',(10.0502525316942,-1.22531840158854,10.6909231138624));
#20662=CARTESIAN_POINT('Ctrl Pts',(11.9668350211294,-0.47638504169901,12.7560692212929));
#20663=CARTESIAN_POINT('Ctrl Pts',(13.8834175105647,0.272548318190524,14.8212153287235));
#20664=CARTESIAN_POINT('Ctrl Pts',(15.8,1.02148167808006,16.886361436154));
#20665=CARTESIAN_POINT('Ctrl Pts',(10.0502525316942,-0.951811288039438,
10.6687583477967));
#20666=CARTESIAN_POINT('Ctrl Pts',(11.9668350211294,-0.160771418505768,
12.7082628707158));
#20667=CARTESIAN_POINT('Ctrl Pts',(13.8834175105647,0.630916858166453,14.7477045483503));
#20668=CARTESIAN_POINT('Ctrl Pts',(15.8,1.42195672770012,16.7872090712694));
#20669=CARTESIAN_POINT('Ctrl Pts',(10.0502525316942,-0.538737970192933,
10.5909841198542));
#20670=CARTESIAN_POINT('Ctrl Pts',(11.9668350211295,0.315735593698357,12.5832583421986));
#20671=CARTESIAN_POINT('Ctrl Pts',(13.8834175105647,1.16942659814005,14.5756107736058));
#20672=CARTESIAN_POINT('Ctrl Pts',(15.8,2.02390016203134,16.5678849959503));
#20673=CARTESIAN_POINT('Ctrl Pts',(10.0502525316942,-0.350797420983486,
10.4118557126012));
#20674=CARTESIAN_POINT('Ctrl Pts',(11.9668350211295,0.527317792292715,12.3552036734465));
#20675=CARTESIAN_POINT('Ctrl Pts',(13.8834175105647,1.40583184426593,14.2985259967778));
#20676=CARTESIAN_POINT('Ctrl Pts',(15.8,2.28394705754214,16.2418739576232));
#20677=CARTESIAN_POINT('Ctrl Pts',(10.0502525316942,-0.276502431596344,
10.2498870013208));
#20678=CARTESIAN_POINT('Ctrl Pts',(11.9668350211295,0.60340579421488,12.1559807242605));
#20679=CARTESIAN_POINT('Ctrl Pts',(13.8834175105647,1.48361038150706,14.0620012424206));
#20680=CARTESIAN_POINT('Ctrl Pts',(15.8,2.36351860731828,15.9680949653604));
#20681=CARTESIAN_POINT('Ctrl Pts',(10.0502525316942,-0.193479460458703,
10.0905890686414));
#20682=CARTESIAN_POINT('Ctrl Pts',(11.9668350211294,0.687106219194375,11.9589846875421));
#20683=CARTESIAN_POINT('Ctrl Pts',(13.8834175105647,1.56802487912709,13.8273908205778));
#20684=CARTESIAN_POINT('Ctrl Pts',(15.8,2.44861055878017,15.6957864394785));
#20685=CARTESIAN_POINT('Ctrl Pts',(10.0502525316942,-0.0477779613143534,
9.85767148446325));
#20686=CARTESIAN_POINT('Ctrl Pts',(11.9668350211294,0.838475123107829,11.6692901486065));
#20687=CARTESIAN_POINT('Ctrl Pts',(13.8834175105647,1.72481200902093,13.4808398643785));
#20688=CARTESIAN_POINT('Ctrl Pts',(15.8,2.61106509344311,15.2924585285217));
#20689=CARTESIAN_POINT('Ctrl Pts',(10.0502525316942,0.0220599042734169,
9.61095465953459));
#20690=CARTESIAN_POINT('Ctrl Pts',(11.9668350211294,0.900879773662288,11.3690757684926));
#20691=CARTESIAN_POINT('Ctrl Pts',(13.8834175105647,1.77979551853006,13.1271782591657));
#20692=CARTESIAN_POINT('Ctrl Pts',(15.8,2.65861538791893,14.8852993681237));
#20693=CARTESIAN_POINT('Ctrl Pts',(10.0502525316942,0.0579833517275568,
9.36700900338232));
#20694=CARTESIAN_POINT('Ctrl Pts',(11.9668350211294,0.920984711114088,11.07518337287));
#20695=CARTESIAN_POINT('Ctrl Pts',(13.8834175105647,1.78409102238058,12.7833535968728));
#20696=CARTESIAN_POINT('Ctrl Pts',(15.8,2.64709238176711,14.4915279663605));
#20697=CARTESIAN_POINT('Ctrl Pts',(10.0502525316942,0.0555068892974573,
9.243940799223));
#20698=CARTESIAN_POINT('Ctrl Pts',(11.9668350211294,0.906948929192825,10.9288207869826));
#20699=CARTESIAN_POINT('Ctrl Pts',(13.8834175105647,1.75838634306183,12.6136545606744));
#20700=CARTESIAN_POINT('Ctrl Pts',(15.8,2.6098283829572,14.298534548434));
#20701=CARTESIAN_POINT('Ctrl Pts',(10.0502525316942,0.0459743785884363,
9.16181196696065));
#20702=CARTESIAN_POINT('Ctrl Pts',(11.9668350211294,0.888076944549314,10.8318459401268));
#20703=CARTESIAN_POINT('Ctrl Pts',(13.8834175105647,1.73017951051019,12.501879913293));
#20704=CARTESIAN_POINT('Ctrl Pts',(15.8,2.57228207647107,14.1719138864591));
#20705=CARTESIAN_POINT('Ctrl Pts',(15.8,2.58416182157067,14.2136654476498));
#20706=CARTESIAN_POINT('Ctrl Pts',(15.8,2.58188195244865,14.2053014035364));
#20707=CARTESIAN_POINT('Ctrl Pts',(15.8,2.57955403215479,14.1969442272588));
#20708=CARTESIAN_POINT('Ctrl Pts',(15.8,2.57717807460939,14.1885939163425));
#20709=CARTESIAN_POINT('Ctrl Pts',(15.8,2.57475408927931,14.1802504694012));
#20710=CARTESIAN_POINT('Ctrl Pts',(15.8,2.57228207647107,14.1719138864591));
#20711=CARTESIAN_POINT('Origin',(15.8,1.34555140976955,14.999291632217));
#20712=CARTESIAN_POINT('Ctrl Pts',(10.0502525316942,2.13832987737225,10.5463163022605));
#20713=CARTESIAN_POINT('Ctrl Pts',(11.9668350211294,3.48877307262933,12.2789538289737));
#20714=CARTESIAN_POINT('Ctrl Pts',(13.8834175105647,4.8392162678864,14.0115913556869));
#20715=CARTESIAN_POINT('Ctrl Pts',(15.8,6.18965946314348,15.7442288824001));
#20716=CARTESIAN_POINT('Ctrl Pts',(10.0502525316942,2.39160131057558,10.4407180108925));
#20717=CARTESIAN_POINT('Ctrl Pts',(11.9668350211294,3.77416649083142,12.1359573145141));
#20718=CARTESIAN_POINT('Ctrl Pts',(13.8834175105647,5.15732892266062,13.8309364798931));
#20719=CARTESIAN_POINT('Ctrl Pts',(15.8,6.53989410291645,15.5261757835147));
#20720=CARTESIAN_POINT('Ctrl Pts',(10.0502525316942,2.7604211119455,10.2391038402362));
#20721=CARTESIAN_POINT('Ctrl Pts',(11.9668350211294,4.18872035504581,11.8698223691572));
#20722=CARTESIAN_POINT('Ctrl Pts',(13.8834175105647,5.61629814839674,13.5008577836237));
#20723=CARTESIAN_POINT('Ctrl Pts',(15.8,7.04459739149705,15.1315763125447));
#20724=CARTESIAN_POINT('Ctrl Pts',(10.0502525316942,2.88380634898392,10.0106660065973));
#20725=CARTESIAN_POINT('Ctrl Pts',(11.9668350211294,4.31947109051328,11.5875472242667));
#20726=CARTESIAN_POINT('Ctrl Pts',(13.8834175105647,5.75550424110768,13.1642822866716));
#20727=CARTESIAN_POINT('Ctrl Pts',(15.8,7.19116898263704,14.7411635043409));
#20728=CARTESIAN_POINT('Ctrl Pts',(10.0502525316942,2.90441220847246,9.83366631411431));
#20729=CARTESIAN_POINT('Ctrl Pts',(11.9668350211294,4.33027001363173,11.3745625747195));
#20730=CARTESIAN_POINT('Ctrl Pts',(13.8834175105647,5.75638324902558,12.9152995332973));
#20731=CARTESIAN_POINT('Ctrl Pts',(15.8,7.18224105418486,14.4561957939025));
#20732=CARTESIAN_POINT('Ctrl Pts',(10.0502525316941,2.93414649567711,9.65650945139357));
#20733=CARTESIAN_POINT('Ctrl Pts',(11.9668350211294,4.34899924292338,11.1613433397504));
#20734=CARTESIAN_POINT('Ctrl Pts',(13.8834175105647,5.76416819477547,12.6660861533134));
#20735=CARTESIAN_POINT('Ctrl Pts',(15.8,7.17902094202174,14.1709200416702));
#20736=CARTESIAN_POINT('Ctrl Pts',(10.0502525316942,3.00074150798572,9.38996734645583));
#20737=CARTESIAN_POINT('Ctrl Pts',(11.9668350211294,4.40343923355921,10.8390518176275));
#20738=CARTESIAN_POINT('Ctrl Pts',(13.8834175105647,5.8061924752444,12.2880463890102));
#20739=CARTESIAN_POINT('Ctrl Pts',(15.8,7.20889020081789,13.7371308601818));
#20740=CARTESIAN_POINT('Ctrl Pts',(10.0502525316942,2.99092345166592,9.13374448664766));
#20741=CARTESIAN_POINT('Ctrl Pts',(11.9668350211294,4.37002011593521,10.5342467491227));
#20742=CARTESIAN_POINT('Ctrl Pts',(13.8834175105647,5.74920012742636,11.9347028120052));
#20743=CARTESIAN_POINT('Ctrl Pts',(15.8,7.12829679169565,13.3352050744803));
#20744=CARTESIAN_POINT('Ctrl Pts',(10.0502525316942,2.94970615383951,8.89063737063806));
#20745=CARTESIAN_POINT('Ctrl Pts',(11.9668350211294,4.29832412978306,10.2485256494886));
#20746=CARTESIAN_POINT('Ctrl Pts',(13.8834175105647,5.64703889510258,11.6063785007713));
#20747=CARTESIAN_POINT('Ctrl Pts',(15.8,6.99565687104613,12.9642667796218));
#20748=CARTESIAN_POINT('Ctrl Pts',(10.0502525316942,2.90932499072146,8.77435756124986));
#20749=CARTESIAN_POINT('Ctrl Pts',(11.9668350211294,4.23975104071156,10.113663592731));
#20750=CARTESIAN_POINT('Ctrl Pts',(13.8834175105647,5.57015841015681,11.4529271015425));
#20751=CARTESIAN_POINT('Ctrl Pts',(15.8,6.90058446014691,12.7922331330237));
#20752=CARTESIAN_POINT('Ctrl Pts',(10.0502525316942,2.87487982939776,8.69919410795919));
#20753=CARTESIAN_POINT('Ctrl Pts',(11.9668350211294,4.19183584103558,10.0272667966845));
#20754=CARTESIAN_POINT('Ctrl Pts',(13.8834175105647,5.5087918526734,11.3553394854098));
#20755=CARTESIAN_POINT('Ctrl Pts',(15.8,6.82574786431122,12.6834121741351));
#20756=CARTESIAN_POINT('Ctrl Pts',(15.8,6.84994811524973,12.7194492253464));
#20757=CARTESIAN_POINT('Ctrl Pts',(15.8,6.84519519909218,12.7121990649934));
#20758=CARTESIAN_POINT('Ctrl Pts',(15.8,6.84039870583253,12.7049702849691));
#20759=CARTESIAN_POINT('Ctrl Pts',(15.8,6.83555864794507,12.6977628786185));
#20760=CARTESIAN_POINT('Ctrl Pts',(15.8,6.83067503400497,12.6905768416977));
#20761=CARTESIAN_POINT('Ctrl Pts',(15.8,6.82574786431122,12.6834121741351));
#20762=CARTESIAN_POINT('Origin',(15.8,5.91473145421246,13.8493757942074));
#20763=CARTESIAN_POINT('Ctrl Pts',(10.0502525316942,5.29266352931554,9.36936257048691));
#20764=CARTESIAN_POINT('Ctrl Pts',(11.9668350211294,7.11242577089738,10.5998888833726));
#20765=CARTESIAN_POINT('Ctrl Pts',(13.8834175105647,8.93218801247923,11.8304151962582));
#20766=CARTESIAN_POINT('Ctrl Pts',(15.8,10.7519502540611,13.0609415091439));
#20767=CARTESIAN_POINT('Ctrl Pts',(10.0502525316942,5.50090730964532,9.19066745032222));
#20768=CARTESIAN_POINT('Ctrl Pts',(11.9668350211294,7.33966268788185,10.3756997001811));
#20769=CARTESIAN_POINT('Ctrl Pts',(13.8834175105647,9.17890569898124,11.5602999829831));
#20770=CARTESIAN_POINT('Ctrl Pts',(15.8,11.0176610772178,12.745332232842));
#20771=CARTESIAN_POINT('Ctrl Pts',(10.0502525316942,5.78937538435654,8.88494866314842));
#20772=CARTESIAN_POINT('Ctrl Pts',(11.9668350211294,7.65168842520523,9.99448540715111));
#20773=CARTESIAN_POINT('Ctrl Pts',(13.8834175105647,9.51341402508183,11.104545703274));
#20774=CARTESIAN_POINT('Ctrl Pts',(15.8,11.3757270659305,12.2140824472767));
#20775=CARTESIAN_POINT('Ctrl Pts',(10.0502525316942,5.83613263565858,8.62956238511758));
#20776=CARTESIAN_POINT('Ctrl Pts',(11.9668350211294,7.68881403767577,9.68562073924798));
#20777=CARTESIAN_POINT('Ctrl Pts',(13.8834175105647,9.54180236671465,10.7414245752752));
#20778=CARTESIAN_POINT('Ctrl Pts',(15.8,11.3944837687318,11.7974829294056));
#20779=CARTESIAN_POINT('Ctrl Pts',(10.0502525316942,5.80103525788045,8.45485763321062));
#20780=CARTESIAN_POINT('Ctrl Pts',(11.9668350211294,7.63326974588329,9.47972276943764));
#20781=CARTESIAN_POINT('Ctrl Pts',(13.8834175105647,9.46570011434026,10.5043553237743));
#20782=CARTESIAN_POINT('Ctrl Pts',(15.8,11.2979346023431,11.5292204600013));
#20783=CARTESIAN_POINT('Ctrl Pts',(10.0502525316941,5.77456941285602,8.27718317134364));
#20784=CARTESIAN_POINT('Ctrl Pts',(11.9668350211294,7.58519358293626,9.27115170336997));
#20785=CARTESIAN_POINT('Ctrl Pts',(13.8834175105647,9.39609248134292,10.2649338319875));
#20786=CARTESIAN_POINT('Ctrl Pts',(15.8,11.2067166514232,11.2589023640138));
#20787=CARTESIAN_POINT('Ctrl Pts',(10.0502525316942,5.75553891274797,8.00310766130011));
#20788=CARTESIAN_POINT('Ctrl Pts',(11.9668350211295,7.53737545292391,8.94781145509674));
#20789=CARTESIAN_POINT('Ctrl Pts',(13.8834175105647,9.31923862861205,9.89241088219743));
#20790=CARTESIAN_POINT('Ctrl Pts',(15.8,11.101075168788,10.8371146759941));
#20791=CARTESIAN_POINT('Ctrl Pts',(10.0502525316942,5.66702291215725,7.76245969237559));
#20792=CARTESIAN_POINT('Ctrl Pts',(11.9668350211294,7.41140078107682,8.66825218904356));
#20793=CARTESIAN_POINT('Ctrl Pts',(13.8834175105647,9.15584481177958,9.57397375447815));
#20794=CARTESIAN_POINT('Ctrl Pts',(15.8,10.9002226806991,10.4797662511461));
#20795=CARTESIAN_POINT('Ctrl Pts',(10.0502525316942,5.55269814935977,7.54398815168985));
#20796=CARTESIAN_POINT('Ctrl Pts',(11.9668350211294,7.25492061800102,8.41867077420536));
#20797=CARTESIAN_POINT('Ctrl Pts',(13.8834175105647,8.95722517253276,9.29328875951754));
#20798=CARTESIAN_POINT('Ctrl Pts',(15.8,10.659447641174,10.167971382033));
#20799=CARTESIAN_POINT('Ctrl Pts',(10.0502525316942,5.47835809159451,7.44587907063767));
#20800=CARTESIAN_POINT('Ctrl Pts',(11.9668350211294,7.15753678028296,8.30851053998513));
#20801=CARTESIAN_POINT('Ctrl Pts',(13.8834175105647,8.83668456248994,9.17110734047641));
#20802=CARTESIAN_POINT('Ctrl Pts',(15.8,10.5158632511784,10.0337388098239));
#20803=CARTESIAN_POINT('Ctrl Pts',(10.0502525316942,5.42237201204004,7.38503851882133));
#20804=CARTESIAN_POINT('Ctrl Pts',(11.9668350211294,7.08526863916361,8.24114891510682));
#20805=CARTESIAN_POINT('Ctrl Pts',(13.8834175105647,8.74816526628719,9.09725931139231));
#20806=CARTESIAN_POINT('Ctrl Pts',(15.8,10.4110618934108,9.9533697076778));
#20807=CARTESIAN_POINT('Ctrl Pts',(15.8,10.4452137610132,9.98016469125221));
#20808=CARTESIAN_POINT('Ctrl Pts',(15.8,10.4384530463692,9.97473811086981));
#20809=CARTESIAN_POINT('Ctrl Pts',(15.8,10.4316574943231,9.96934533045351));
#20810=CARTESIAN_POINT('Ctrl Pts',(15.8,10.4248271146823,9.96398633981914));
#20811=CARTESIAN_POINT('Ctrl Pts',(15.8,10.4179619142908,9.95866113228077));
#20812=CARTESIAN_POINT('Ctrl Pts',(15.8,10.4110618934108,9.9533697076778));
#20813=CARTESIAN_POINT('Origin',(15.8,9.90493637355978,11.3437865591856));
#20814=CARTESIAN_POINT('Ctrl Pts',(10.0502525316942,7.92891439885425,7.2752703501265));
#20815=CARTESIAN_POINT('Ctrl Pts',(11.9668350211294,10.0398646795257,7.88323296009842));
#20816=CARTESIAN_POINT('Ctrl Pts',(13.8834175105647,12.1508149601973,8.49119557007034));
#20817=CARTESIAN_POINT('Ctrl Pts',(15.8,14.2617652408688,9.09915818004226));
#20818=CARTESIAN_POINT('Ctrl Pts',(10.0502525316942,8.07174617417204,7.04097032456894));
#20819=CARTESIAN_POINT('Ctrl Pts',(11.9668350211294,10.186749261509,7.59972129962697));
#20820=CARTESIAN_POINT('Ctrl Pts',(13.8834175105647,12.3019395333854,8.15813578620935));
#20821=CARTESIAN_POINT('Ctrl Pts',(15.8,14.4169426207224,8.71688676126738));
#20822=CARTESIAN_POINT('Ctrl Pts',(10.0502525316942,8.25126590443757,6.66138127597024));
#20823=CARTESIAN_POINT('Ctrl Pts',(11.9668350211294,10.365200404417,7.14127838379811));
#20824=CARTESIAN_POINT('Ctrl Pts',(13.8834175105647,12.4788866778492,7.62165928459738));
#20825=CARTESIAN_POINT('Ctrl Pts',(15.8,14.5928211778287,8.10155639242526));
#20826=CARTESIAN_POINT('Ctrl Pts',(10.0502525316942,8.22079862024226,6.42930419296207));
#20827=CARTESIAN_POINT('Ctrl Pts',(11.9668350211294,10.3118069242151,6.86580395314968));
#20828=CARTESIAN_POINT('Ctrl Pts',(13.8834175105647,12.4027801127282,7.30234839548021));
#20829=CARTESIAN_POINT('Ctrl Pts',(15.8,14.493788416701,7.73884815566781));
#20830=CARTESIAN_POINT('Ctrl Pts',(10.0502525316942,8.16221173215365,6.30697938690416));
#20831=CARTESIAN_POINT('Ctrl Pts',(11.9668350211294,10.2323186327506,6.72434771418857));
#20832=CARTESIAN_POINT('Ctrl Pts',(13.8834175105647,12.3026176380752,7.1413715062851));
#20833=CARTESIAN_POINT('Ctrl Pts',(15.8,14.3727245386721,7.55873983356951));
#20834=CARTESIAN_POINT('Ctrl Pts',(10.0502525316942,8.12000643506487,6.22815403351084));
#20835=CARTESIAN_POINT('Ctrl Pts',(11.9668350211294,10.1755454476056,6.63375833246636));
#20836=CARTESIAN_POINT('Ctrl Pts',(13.8834175105647,12.2311493413123,7.03916552489903));
#20837=CARTESIAN_POINT('Ctrl Pts',(15.8,14.2866883538531,7.44476982385454));
#20838=CARTESIAN_POINT('Ctrl Pts',(10.0502525316942,8.04942040067478,6.08789997184504));
#20839=CARTESIAN_POINT('Ctrl Pts',(11.9668350211294,10.0785454407991,6.47376321403759));
#20840=CARTESIAN_POINT('Ctrl Pts',(13.8834175105647,12.1078515605739,6.85942462405723));
#20841=CARTESIAN_POINT('Ctrl Pts',(15.8,14.1369766006982,7.24528786624978));
#20842=CARTESIAN_POINT('Ctrl Pts',(10.0502525316942,7.94713925110584,5.83267830770086));
#20843=CARTESIAN_POINT('Ctrl Pts',(11.9668350211294,9.93371906448114,6.18048893841474));
#20844=CARTESIAN_POINT('Ctrl Pts',(13.8834175105647,11.920292369998,6.52817426230452));
#20845=CARTESIAN_POINT('Ctrl Pts',(15.8,13.9068721833733,6.8759848930184));
#20846=CARTESIAN_POINT('Ctrl Pts',(10.0502525316942,7.78832910259186,5.63138575926578));
#20847=CARTESIAN_POINT('Ctrl Pts',(11.9668350211294,9.72722511219089,5.95382183425815));
#20848=CARTESIAN_POINT('Ctrl Pts',(13.8834175105647,11.6661698490829,6.27616146093386));
#20849=CARTESIAN_POINT('Ctrl Pts',(15.8,13.605065858682,6.59859753592622));
#20850=CARTESIAN_POINT('Ctrl Pts',(10.0502525316942,7.61219406851114,5.45884429554414));
#20851=CARTESIAN_POINT('Ctrl Pts',(11.9668350211294,9.50140467053761,5.76468621283309));
#20852=CARTESIAN_POINT('Ctrl Pts',(13.8834175105648,11.3906602079427,6.07045912241829));
#20853=CARTESIAN_POINT('Ctrl Pts',(15.8,13.2798708099692,6.37630103970724));
#20854=CARTESIAN_POINT('Ctrl Pts',(10.0502525316942,7.51113133249701,5.38854605810145));
#20855=CARTESIAN_POINT('Ctrl Pts',(11.9668350211294,9.37468648227302,5.69007333772413));
#20856=CARTESIAN_POINT('Ctrl Pts',(13.8834175105647,11.238220929081,5.99154494312677));
#20857=CARTESIAN_POINT('Ctrl Pts',(15.8,13.101776078857,6.29307222274946));
#20858=CARTESIAN_POINT('Ctrl Pts',(10.0502525316942,7.43908464225652,5.34798390487229));
#20859=CARTESIAN_POINT('Ctrl Pts',(11.9668350211294,9.28514597692092,5.64832995825767));
#20860=CARTESIAN_POINT('Ctrl Pts',(13.8834175105647,11.1312073115853,5.94867601164304));
#20861=CARTESIAN_POINT('Ctrl Pts',(15.8,12.9772686462497,6.24902206502841));
#20862=CARTESIAN_POINT('Ctrl Pts',(15.8,13.0180291077652,6.26395210128207));
#20863=CARTESIAN_POINT('Ctrl Pts',(15.8,13.0099223804886,6.26088029236733));
#20864=CARTESIAN_POINT('Ctrl Pts',(15.8,13.0017929656379,6.25785139447984));
#20865=CARTESIAN_POINT('Ctrl Pts',(15.8,12.993640869393,6.25486539490331));
#20866=CARTESIAN_POINT('Ctrl Pts',(15.8,12.985466096197,6.25192228516409));
#20867=CARTESIAN_POINT('Ctrl Pts',(15.8,12.9772686462497,6.24902206502841));
#20868=CARTESIAN_POINT('Origin',(15.8,12.9255771089134,7.7277884589423));
#20869=CARTESIAN_POINT('Ctrl Pts',(10.0502525316942,9.78902788303806,4.46902397810655));
#20870=CARTESIAN_POINT('Ctrl Pts',(11.9668350211294,11.9845316814717,4.39491126897609));
#20871=CARTESIAN_POINT('Ctrl Pts',(13.8834175105647,14.1800354799052,4.32079855984564));
#20872=CARTESIAN_POINT('Ctrl Pts',(15.8,16.3755392783388,4.24668585071518));
#20873=CARTESIAN_POINT('Ctrl Pts',(10.0502525316942,9.8524662840083,4.20205396612197));
#20874=CARTESIAN_POINT('Ctrl Pts',(11.9668350211294,12.036617299121,4.07988582479457));
#20875=CARTESIAN_POINT('Ctrl Pts',(13.8834175105647,14.2208423566523,3.95733982070599));
#20876=CARTESIAN_POINT('Ctrl Pts',(15.8,16.404993371765,3.83517167937859));
#20877=CARTESIAN_POINT('Ctrl Pts',(10.0502525316942,9.90590216992165,3.7855656109216));
#20878=CARTESIAN_POINT('Ctrl Pts',(11.9668350211295,12.0646697130184,3.58873319698334));
#20879=CARTESIAN_POINT('Ctrl Pts',(13.8834175105648,14.2233509855394,3.39243568541407));
#20880=CARTESIAN_POINT('Ctrl Pts',(15.8,16.3821185286362,3.19560327147581));
#20881=CARTESIAN_POINT('Ctrl Pts',(10.0502525316942,9.80521299123423,3.57425782911967));
#20882=CARTESIAN_POINT('Ctrl Pts',(11.9668350211295,11.9287659082934,3.34323666910062));
#20883=CARTESIAN_POINT('Ctrl Pts',(13.8834175105647,14.052299961954,3.11226431322855));
#20884=CARTESIAN_POINT('Ctrl Pts',(15.8,16.1758528790132,2.8812431532095));
#20885=CARTESIAN_POINT('Ctrl Pts',(10.0502525316942,9.71169428155717,3.47602249721153));
#20886=CARTESIAN_POINT('Ctrl Pts',(11.9668350211295,11.8094568448422,3.23326515211327));
#20887=CARTESIAN_POINT('Ctrl Pts',(13.8834175105647,13.9072965714997,2.99011502771358));
#20888=CARTESIAN_POINT('Ctrl Pts',(15.8,16.0050591347847,2.74735768261532));
#20889=CARTESIAN_POINT('Ctrl Pts',(10.0502525316942,9.64719632995104,3.41409722674601));
#20890=CARTESIAN_POINT('Ctrl Pts',(11.9668350211295,11.7274687236956,3.16465335082919));
#20891=CARTESIAN_POINT('Ctrl Pts',(13.8834175105648,13.8077428217682,2.91499625447087));
#20892=CARTESIAN_POINT('Ctrl Pts',(15.8,15.8880152155128,2.66555237855405));
#20893=CARTESIAN_POINT('Ctrl Pts',(10.0502525316942,9.53672408685998,3.30251999207182));
#20894=CARTESIAN_POINT('Ctrl Pts',(11.9668350211294,11.58577497799,3.04246362184767));
#20895=CARTESIAN_POINT('Ctrl Pts',(13.8834175105647,13.6349367240444,2.78215337892879));
#20896=CARTESIAN_POINT('Ctrl Pts',(15.8,15.6839876151744,2.52209700870464));
#20897=CARTESIAN_POINT('Ctrl Pts',(10.0502525316942,9.36058107581317,3.09139659750778));
#20898=CARTESIAN_POINT('Ctrl Pts',(11.9668350211295,11.357410148179,2.80829724126977));
#20899=CARTESIAN_POINT('Ctrl Pts',(13.8834175105647,13.3541948572957,2.52507603204707));
#20900=CARTESIAN_POINT('Ctrl Pts',(15.8,15.3510239296616,2.24197667580906));
#20901=CARTESIAN_POINT('Ctrl Pts',(10.0502525316942,9.14733948977136,2.94903314862295));
#20902=CARTESIAN_POINT('Ctrl Pts',(11.9668350211294,11.0909774008914,2.65653626154119));
#20903=CARTESIAN_POINT('Ctrl Pts',(13.8834175105647,13.0346322911662,2.3639289644162));
#20904=CARTESIAN_POINT('Ctrl Pts',(15.8,14.9782702022862,2.07143207733445));
#20905=CARTESIAN_POINT('Ctrl Pts',(10.0502525316942,8.92650608260145,2.83936642791009));
#20906=CARTESIAN_POINT('Ctrl Pts',(11.9668350211294,10.8177624863471,2.54644119432445));
#20907=CARTESIAN_POINT('Ctrl Pts',(13.8834175105648,12.7090406610097,2.25343349088951));
#20908=CARTESIAN_POINT('Ctrl Pts',(15.8,14.6002970647553,1.96050825730386));
#20909=CARTESIAN_POINT('Ctrl Pts',(10.0502525316942,8.80866270544546,2.80374461319022));
#20910=CARTESIAN_POINT('Ctrl Pts',(11.9668350211294,10.6741860277864,2.51464388608039));
#20911=CARTESIAN_POINT('Ctrl Pts',(13.8834175105647,12.5396724561545,2.22549660720977));
#20912=CARTESIAN_POINT('Ctrl Pts',(15.8,14.4051957784954,1.93639588009994));
#20913=CARTESIAN_POINT('Ctrl Pts',(10.0502525316942,8.7276078365385,2.78743136471945));
#20914=CARTESIAN_POINT('Ctrl Pts',(11.9668350211294,10.5761285330411,2.50261311086535));
#20915=CARTESIAN_POINT('Ctrl Pts',(13.8834175105647,12.4246492295437,2.21779485701125));
#20916=CARTESIAN_POINT('Ctrl Pts',(15.8,14.2731699260464,1.93297660315714));
#20917=CARTESIAN_POINT('Ctrl Pts',(15.8,14.3165490635069,1.93458023611785));
#20918=CARTESIAN_POINT('Ctrl Pts',(15.8,14.3078898665466,1.93416388872989));
#20919=CARTESIAN_POINT('Ctrl Pts',(15.8,14.2992223526576,1.93379536300002));
#20920=CARTESIAN_POINT('Ctrl Pts',(15.8,14.2905465237881,1.93347464492456));
#20921=CARTESIAN_POINT('Ctrl Pts',(15.8,14.2818623815451,1.93320172507161));
#20922=CARTESIAN_POINT('Ctrl Pts',(15.8,14.2731699260464,1.93297660315714));
#20923=CARTESIAN_POINT('Origin',(15.8,14.6809722990553,3.35534058166953));
#20924=CARTESIAN_POINT('Ctrl Pts',(10.0502525316942,10.6909231138624,1.22531840158854));
#20925=CARTESIAN_POINT('Ctrl Pts',(11.9668350211294,12.7560692212929,0.476385041699011));
#20926=CARTESIAN_POINT('Ctrl Pts',(13.8834175105647,14.8212153287235,-0.272548318190523));
#20927=CARTESIAN_POINT('Ctrl Pts',(15.8,16.886361436154,-1.02148167808006));
#20928=CARTESIAN_POINT('Ctrl Pts',(10.0502525316942,10.6687583477967,0.951811288039439));
#20929=CARTESIAN_POINT('Ctrl Pts',(11.9668350211294,12.7082628707158,0.160771418505769));
#20930=CARTESIAN_POINT('Ctrl Pts',(13.8834175105647,14.7477045483503,-0.630916858166452));
#20931=CARTESIAN_POINT('Ctrl Pts',(15.8,16.7872090712694,-1.42195672770012));
#20932=CARTESIAN_POINT('Ctrl Pts',(10.0502525316942,10.5909841198542,0.538737970192933));
#20933=CARTESIAN_POINT('Ctrl Pts',(11.9668350211295,12.5832583421986,-0.315735593698355));
#20934=CARTESIAN_POINT('Ctrl Pts',(13.8834175105647,14.5756107736058,-1.16942659814004));
#20935=CARTESIAN_POINT('Ctrl Pts',(15.8,16.5678849959503,-2.02390016203133));
#20936=CARTESIAN_POINT('Ctrl Pts',(10.0502525316942,10.4118557126012,0.350797420983487));
#20937=CARTESIAN_POINT('Ctrl Pts',(11.9668350211295,12.3552036734465,-0.527317792292714));
#20938=CARTESIAN_POINT('Ctrl Pts',(13.8834175105647,14.2985259967778,-1.40583184426593));
#20939=CARTESIAN_POINT('Ctrl Pts',(15.8,16.2418739576232,-2.28394705754213));
#20940=CARTESIAN_POINT('Ctrl Pts',(10.0502525316942,10.2498870013208,0.276502431596345));
#20941=CARTESIAN_POINT('Ctrl Pts',(11.9668350211295,12.1559807242605,-0.603405794214879));
#20942=CARTESIAN_POINT('Ctrl Pts',(13.8834175105647,14.0620012424206,-1.48361038150706));
#20943=CARTESIAN_POINT('Ctrl Pts',(15.8,15.9680949653604,-2.36351860731828));
#20944=CARTESIAN_POINT('Ctrl Pts',(10.0502525316942,10.0905890686414,0.193479460458704));
#20945=CARTESIAN_POINT('Ctrl Pts',(11.9668350211294,11.9589846875421,-0.687106219194374));
#20946=CARTESIAN_POINT('Ctrl Pts',(13.8834175105647,13.8273908205778,-1.56802487912709));
#20947=CARTESIAN_POINT('Ctrl Pts',(15.8,15.6957864394785,-2.44861055878017));
#20948=CARTESIAN_POINT('Ctrl Pts',(10.0502525316942,9.85767148446325,0.0477779613143544));
#20949=CARTESIAN_POINT('Ctrl Pts',(11.9668350211294,11.6692901486065,-0.83847512310783));
#20950=CARTESIAN_POINT('Ctrl Pts',(13.8834175105647,13.4808398643785,-1.72481200902093));
#20951=CARTESIAN_POINT('Ctrl Pts',(15.8,15.2924585285217,-2.61106509344312));
#20952=CARTESIAN_POINT('Ctrl Pts',(10.0502525316942,9.61095465953459,-0.0220599042734161));
#20953=CARTESIAN_POINT('Ctrl Pts',(11.9668350211294,11.3690757684926,-0.900879773662285));
#20954=CARTESIAN_POINT('Ctrl Pts',(13.8834175105647,13.1271782591657,-1.77979551853006));
#20955=CARTESIAN_POINT('Ctrl Pts',(15.8,14.8852993681237,-2.65861538791893));
#20956=CARTESIAN_POINT('Ctrl Pts',(10.0502525316942,9.36700900338232,-0.0579833517275561));
#20957=CARTESIAN_POINT('Ctrl Pts',(11.9668350211294,11.07518337287,-0.920984711114089));
#20958=CARTESIAN_POINT('Ctrl Pts',(13.8834175105647,12.7833535968728,-1.78409102238058));
#20959=CARTESIAN_POINT('Ctrl Pts',(15.8,14.4915279663605,-2.64709238176711));
#20960=CARTESIAN_POINT('Ctrl Pts',(10.0502525316942,9.243940799223,-0.0555068892974567));
#20961=CARTESIAN_POINT('Ctrl Pts',(11.9668350211294,10.9288207869826,-0.906948929192822));
#20962=CARTESIAN_POINT('Ctrl Pts',(13.8834175105647,12.6136545606744,-1.75838634306183));
#20963=CARTESIAN_POINT('Ctrl Pts',(15.8,14.298534548434,-2.6098283829572));
#20964=CARTESIAN_POINT('Ctrl Pts',(10.0502525316942,9.16181196696065,-0.0459743785884358));
#20965=CARTESIAN_POINT('Ctrl Pts',(11.9668350211294,10.8318459401268,-0.888076944549314));
#20966=CARTESIAN_POINT('Ctrl Pts',(13.8834175105647,12.501879913293,-1.73017951051019));
#20967=CARTESIAN_POINT('Ctrl Pts',(15.8,14.1719138864591,-2.57228207647107));
#20968=CARTESIAN_POINT('Ctrl Pts',(15.8,14.2136654476498,-2.58416182157067));
#20969=CARTESIAN_POINT('Ctrl Pts',(15.8,14.2053014035364,-2.58188195244865));
#20970=CARTESIAN_POINT('Ctrl Pts',(15.8,14.1969442272588,-2.57955403215479));
#20971=CARTESIAN_POINT('Ctrl Pts',(15.8,14.1885939163425,-2.57717807460939));
#20972=CARTESIAN_POINT('Ctrl Pts',(15.8,14.1802504694012,-2.57475408927931));
#20973=CARTESIAN_POINT('Ctrl Pts',(15.8,14.1719138864591,-2.57228207647107));
#20974=CARTESIAN_POINT('Origin',(15.8,14.999291632217,-1.34555140976955));
#20975=CARTESIAN_POINT('Origin',(21.,10.,0.));
#23234=UNCERTAINTY_MEASURE_WITH_UNIT(LENGTH_MEASURE(0.01),#23255,
'DISTANCE_ACCURACY_VALUE',
'Maximum model space distance between geometric entities at asserted c
onnectivities');
#23242=UNCERTAINTY_MEASURE_WITH_UNIT(LENGTH_MEASURE(0.01),#23255,
'DISTANCE_ACCURACY_VALUE',
'Maximum model space distance between geometric entities at asserted c
onnectivities');
#23246=(
GEOMETRIC_REPRESENTATION_CONTEXT(3)
GLOBAL_UNCERTAINTY_ASSIGNED_CONTEXT((#23234))
GLOBAL_UNIT_ASSIGNED_CONTEXT((#23255,#23257,#23258))
REPRESENTATION_CONTEXT('','3D')
);
#23254=(
GEOMETRIC_REPRESENTATION_CONTEXT(3)
GLOBAL_UNCERTAINTY_ASSIGNED_CONTEXT((#23242))
GLOBAL_UNIT_ASSIGNED_CONTEXT((#23255,#23257,#23258))
REPRESENTATION_CONTEXT('','3D')
);
#23255=(
LENGTH_UNIT()
NAMED_UNIT(*)
SI_UNIT(.MILLI.,.METRE.)
);
#23257=(
NAMED_UNIT(*)
PLANE_ANGLE_UNIT()
SI_UNIT($,.RADIAN.)
);
#23258=(
NAMED_UNIT(*)
SI_UNIT($,.STERADIAN.)
SOLID_ANGLE_UNIT()
);
#23262=SHAPE_DEFINITION_REPRESENTATION(#23273,#23302);
#23273=PRODUCT_DEFINITION_SHAPE('',$,#23314);
#23302=SHAPE_REPRESENTATION('',(#7412),#23246);
#23310=PRODUCT_DEFINITION_CONTEXT('part definition',#23345,'design');
#23314=PRODUCT_DEFINITION('2026-10-11-09-11-49-846',
'03_Spiral_Bevel_Output_Gear_M1.5_Z20_RH',#23325,#23310);
#23325=PRODUCT_DEFINITION_FORMATION('',$,#23350);
#23345=APPLICATION_CONTEXT(
'Core Data for Automotive Mechanical Design Process');
#23346=PRODUCT_CONTEXT('part definition',#23345,'mechanical');
#23350=PRODUCT('2026-10-11-09-11-49-846',
'03_Spiral_Bevel_Output_Gear_M1.5_Z20_RH',$,(#23346));
#23449=COLOUR_RGB('Sky Blue',0.24,0.69,0.87);
#23450=FILL_AREA_STYLE_COLOUR('',#23449);
#23451=FILL_AREA_STYLE('',(#23450));
#23452=SURFACE_STYLE_FILL_AREA(#23451);
#23453=SURFACE_SIDE_STYLE('',(#23452));
#23454=SURFACE_STYLE_USAGE(.BOTH.,#23453);
#23455=PRESENTATION_STYLE_ASSIGNMENT((#23454));
ENDSEC;
END-ISO-10303-21;
